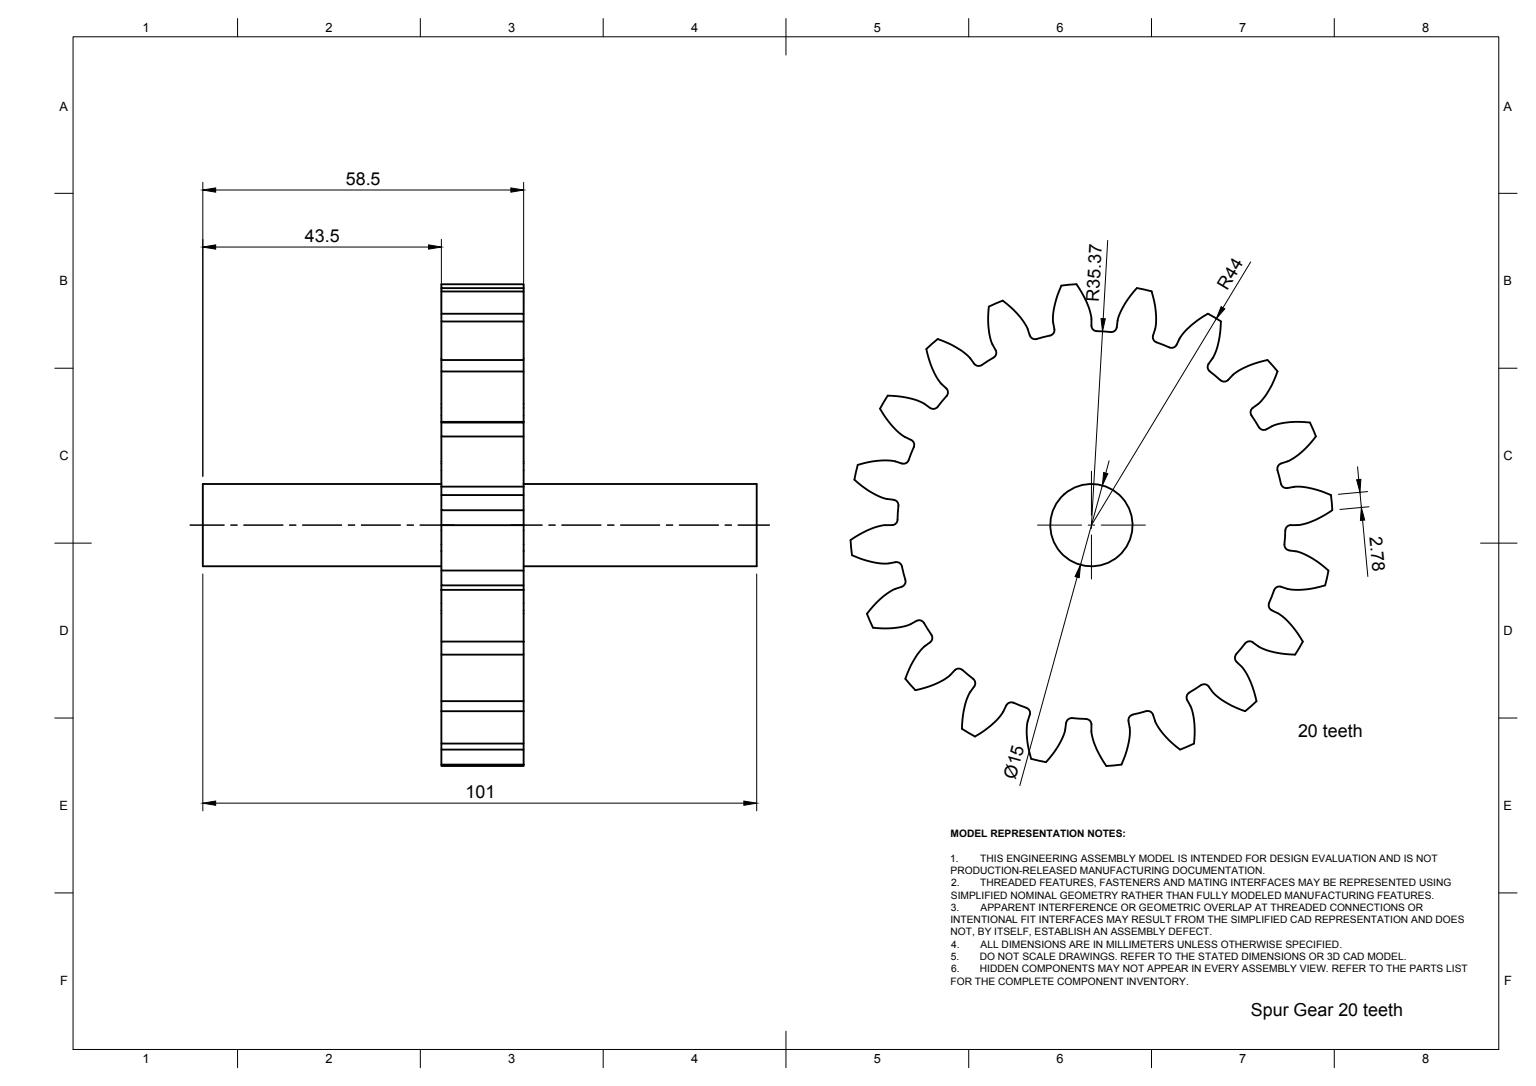
ISO-10303-21;
HEADER;
/* Generated by software containing ST-Developer
 * from STEP Tools, Inc. (www.steptools.com) 
 */

FILE_DESCRIPTION(
/* description */ (''),
/* implementation_level */ '2;1');

FILE_NAME(
/* name */ 'Spur Gear 20 teeth.step',
/* time_stamp */ '2026-10-05T21:54:13-07:00',
/* author */ (''),
/* organization */ (''),
/* preprocessor_version */ 'ST-DEVELOPER v20.2',
/* originating_system */ 'Autodesk Translation Framework v15.15.0.0',
/* authorisation */ '');

FILE_SCHEMA (('AUTOMOTIVE_DESIGN { 1 0 10303 214 3 1 1 }'));
ENDSEC;

DATA;
#10=MECHANICAL_DESIGN_GEOMETRIC_PRESENTATION_REPRESENTATION('',(#191),#43781);
#175=SHAPE_REPRESENTATION_RELATIONSHIP('SRR','None',#43813,#183);
#183=ADVANCED_BREP_SHAPE_REPRESENTATION('',(#235),#43773);
#191=STYLED_ITEM('',(#43862),#235);
#235=MANIFOLD_SOLID_BREP('Body1',#13051);
#279=FACE_BOUND('',#2177,.T.);
#280=FACE_BOUND('',#2179,.T.);
#491=B_SPLINE_CURVE_WITH_KNOTS('',5,(#19556,#19557,#19558,#19559,#19560,
#19561,#19562,#19563,#19564,#19565,#19566,#19567,#19568,#19569,#19570,#19571,
#19572,#19573,#19574,#19575,#19576,#19577,#19578,#19579,#19580,#19581,#19582,
#19583,#19584,#19585,#19586,#19587,#19588,#19589,#19590,#19591,#19592,#19593,
#19594,#19595,#19596,#19597,#19598,#19599,#19600,#19601,#19602,#19603,#19604,
#19605,#19606,#19607,#19608,#19609,#19610,#19611,#19612,#19613,#19614,#19615,
#19616,#19617,#19618,#19619,#19620,#19621,#19622,#19623,#19624,#19625,#19626,
#19627,#19628,#19629),.UNSPECIFIED.,.F.,.F.,(6,1,1,1,1,1,1,1,1,1,1,1,1,
1,1,1,1,1,1,1,1,1,1,1,1,1,1,1,1,1,1,1,1,1,1,1,1,1,1,1,1,1,1,1,1,1,1,1,1,
1,1,1,1,1,1,1,1,1,1,1,1,1,1,1,1,1,1,1,1,6),(0.,0.0142857142857143,0.0285714285714286,
0.0428571428571429,0.0571428571428571,0.0714285714285714,0.0857142857142857,
0.1,0.114285714285714,0.128571428571429,0.142857142857143,0.157142857142857,
0.171428571428571,0.185714285714286,0.2,0.214285714285714,0.228571428571429,
0.242857142857143,0.257142857142857,0.271428571428571,0.285714285714286,
0.3,0.314285714285714,0.328571428571429,0.342857142857143,0.357142857142857,
0.371428571428571,0.385714285714286,0.4,0.414285714285714,0.428571428571429,
0.442857142857143,0.457142857142857,0.471428571428572,0.485714285714286,
0.5,0.514285714285714,0.528571428571429,0.542857142857143,0.557142857142857,
0.571428571428571,0.585714285714286,0.6,0.614285714285714,0.628571428571428,
0.642857142857142,0.657142857142857,0.671428571428571,0.685714285714285,
0.699999999999999,0.714285714285714,0.728571428571428,0.742857142857142,
0.757142857142856,0.771428571428571,0.785714285714285,0.799999999999999,
0.814285714285713,0.828571428571428,0.842857142857142,0.857142857142856,
0.87142857142857,0.885714285714284,0.899999999999999,0.914285714285713,
0.928571428571427,0.942857142857141,0.957142857142856,0.97142857142857,
1.),.UNSPECIFIED.);
#492=B_SPLINE_CURVE_WITH_KNOTS('',5,(#19631,#19632,#19633,#19634,#19635,
#19636,#19637,#19638,#19639,#19640,#19641,#19642,#19643,#19644,#19645,#19646,
#19647,#19648,#19649,#19650,#19651,#19652,#19653,#19654,#19655,#19656,#19657,
#19658,#19659,#19660,#19661,#19662,#19663,#19664,#19665,#19666,#19667,#19668,
#19669,#19670,#19671,#19672,#19673,#19674,#19675,#19676,#19677,#19678,#19679,
#19680,#19681,#19682,#19683,#19684,#19685,#19686,#19687,#19688,#19689,#19690,
#19691,#19692,#19693,#19694,#19695,#19696,#19697,#19698,#19699,#19700,#19701,
#19702,#19703,#19704,#19705),.UNSPECIFIED.,.F.,.F.,(6,1,1,1,1,1,1,1,1,1,
1,1,1,1,1,1,1,1,1,1,1,1,1,1,1,1,1,1,1,1,1,1,1,1,1,1,1,1,1,1,1,1,1,1,1,1,
1,1,1,1,1,1,1,1,1,1,1,1,1,1,1,1,1,1,1,1,1,1,1,1,6),(-1.,-0.985714285714284,
-0.97142857142857,-0.957142857142856,-0.942857142857141,-0.928571428571427,
-0.914285714285713,-0.899999999999999,-0.885714285714284,-0.87142857142857,
-0.857142857142856,-0.842857142857142,-0.828571428571428,-0.814285714285713,
-0.799999999999999,-0.785714285714285,-0.771428571428571,-0.757142857142856,
-0.742857142857142,-0.728571428571428,-0.714285714285714,-0.699999999999999,
-0.685714285714285,-0.671428571428571,-0.657142857142857,-0.642857142857142,
-0.628571428571428,-0.614285714285714,-0.6,-0.585714285714286,-0.571428571428571,
-0.557142857142857,-0.542857142857143,-0.528571428571429,-0.514285714285714,
-0.5,-0.485714285714286,-0.471428571428572,-0.457142857142857,-0.442857142857143,
-0.428571428571429,-0.414285714285714,-0.4,-0.385714285714286,-0.371428571428571,
-0.357142857142857,-0.342857142857143,-0.328571428571429,-0.314285714285714,
-0.3,-0.285714285714286,-0.271428571428571,-0.257142857142857,-0.242857142857143,
-0.228571428571429,-0.214285714285714,-0.2,-0.185714285714286,-0.171428571428571,
-0.157142857142857,-0.142857142857143,-0.128571428571429,-0.114285714285714,
-0.1,-0.0857142857142857,-0.0714285714285714,-0.0571428571428571,-0.0428571428571429,
-0.0285714285714286,-0.0142857142857143,0.),.UNSPECIFIED.);
#493=B_SPLINE_CURVE_WITH_KNOTS('',5,(#19863,#19864,#19865,#19866,#19867,
#19868,#19869,#19870,#19871,#19872,#19873,#19874,#19875,#19876,#19877,#19878,
#19879,#19880,#19881,#19882,#19883,#19884,#19885,#19886,#19887,#19888,#19889,
#19890,#19891,#19892,#19893,#19894,#19895,#19896,#19897,#19898,#19899,#19900,
#19901,#19902,#19903,#19904,#19905,#19906,#19907,#19908,#19909,#19910,#19911,
#19912,#19913,#19914,#19915,#19916,#19917,#19918,#19919,#19920,#19921,#19922,
#19923,#19924,#19925,#19926,#19927,#19928,#19929,#19930,#19931,#19932,#19933,
#19934,#19935,#19936),.UNSPECIFIED.,.F.,.F.,(6,1,1,1,1,1,1,1,1,1,1,1,1,
1,1,1,1,1,1,1,1,1,1,1,1,1,1,1,1,1,1,1,1,1,1,1,1,1,1,1,1,1,1,1,1,1,1,1,1,
1,1,1,1,1,1,1,1,1,1,1,1,1,1,1,1,1,1,1,1,6),(0.,0.0142857142857143,0.0285714285714286,
0.0428571428571429,0.0571428571428571,0.0714285714285714,0.0857142857142857,
0.1,0.114285714285714,0.128571428571429,0.142857142857143,0.157142857142857,
0.171428571428571,0.185714285714286,0.2,0.214285714285714,0.228571428571429,
0.242857142857143,0.257142857142857,0.271428571428571,0.285714285714286,
0.3,0.314285714285714,0.328571428571429,0.342857142857143,0.357142857142857,
0.371428571428571,0.385714285714286,0.4,0.414285714285714,0.428571428571429,
0.442857142857143,0.457142857142857,0.471428571428572,0.485714285714286,
0.5,0.514285714285714,0.528571428571429,0.542857142857143,0.557142857142857,
0.571428571428571,0.585714285714286,0.6,0.614285714285714,0.628571428571428,
0.642857142857142,0.657142857142857,0.671428571428571,0.685714285714285,
0.699999999999999,0.714285714285714,0.728571428571428,0.742857142857142,
0.757142857142856,0.771428571428571,0.785714285714285,0.799999999999999,
0.814285714285713,0.828571428571428,0.842857142857142,0.857142857142856,
0.87142857142857,0.885714285714284,0.899999999999999,0.914285714285713,
0.928571428571427,0.942857142857141,0.957142857142856,0.97142857142857,
1.),.UNSPECIFIED.);
#494=B_SPLINE_CURVE_WITH_KNOTS('',5,(#19937,#19938,#19939,#19940,#19941,
#19942,#19943,#19944,#19945,#19946,#19947,#19948,#19949,#19950,#19951,#19952,
#19953,#19954,#19955,#19956,#19957,#19958,#19959,#19960,#19961,#19962,#19963,
#19964,#19965,#19966,#19967,#19968,#19969,#19970,#19971,#19972,#19973,#19974,
#19975,#19976,#19977,#19978,#19979,#19980,#19981,#19982,#19983,#19984,#19985,
#19986,#19987,#19988,#19989,#19990,#19991,#19992,#19993,#19994,#19995,#19996,
#19997,#19998,#19999,#20000,#20001,#20002,#20003,#20004,#20005,#20006,#20007,
#20008,#20009,#20010),.UNSPECIFIED.,.F.,.F.,(6,1,1,1,1,1,1,1,1,1,1,1,1,
1,1,1,1,1,1,1,1,1,1,1,1,1,1,1,1,1,1,1,1,1,1,1,1,1,1,1,1,1,1,1,1,1,1,1,1,
1,1,1,1,1,1,1,1,1,1,1,1,1,1,1,1,1,1,1,1,6),(0.,0.0142857142857143,0.0285714285714286,
0.0428571428571429,0.0571428571428571,0.0714285714285714,0.0857142857142857,
0.1,0.114285714285714,0.128571428571429,0.142857142857143,0.157142857142857,
0.171428571428571,0.185714285714286,0.2,0.214285714285714,0.228571428571429,
0.242857142857143,0.257142857142857,0.271428571428571,0.285714285714286,
0.3,0.314285714285714,0.328571428571429,0.342857142857143,0.357142857142857,
0.371428571428571,0.385714285714286,0.4,0.414285714285714,0.428571428571429,
0.442857142857143,0.457142857142857,0.471428571428572,0.485714285714286,
0.5,0.514285714285714,0.528571428571429,0.542857142857143,0.557142857142857,
0.571428571428571,0.585714285714286,0.6,0.614285714285714,0.628571428571428,
0.642857142857142,0.657142857142857,0.671428571428571,0.685714285714285,
0.699999999999999,0.714285714285714,0.728571428571428,0.742857142857142,
0.757142857142856,0.771428571428571,0.785714285714285,0.799999999999999,
0.814285714285713,0.828571428571428,0.842857142857142,0.857142857142856,
0.87142857142857,0.885714285714284,0.899999999999999,0.914285714285713,
0.928571428571427,0.942857142857141,0.957142857142856,0.97142857142857,
1.),.UNSPECIFIED.);
#495=B_SPLINE_CURVE_WITH_KNOTS('',5,(#20162,#20163,#20164,#20165,#20166,
#20167,#20168,#20169,#20170,#20171,#20172,#20173,#20174,#20175,#20176,#20177,
#20178,#20179,#20180,#20181,#20182,#20183,#20184,#20185,#20186,#20187,#20188,
#20189,#20190,#20191,#20192,#20193,#20194,#20195,#20196,#20197,#20198,#20199,
#20200,#20201,#20202,#20203,#20204,#20205,#20206,#20207,#20208,#20209,#20210,
#20211,#20212,#20213,#20214,#20215,#20216,#20217,#20218,#20219,#20220,#20221,
#20222,#20223,#20224,#20225,#20226,#20227,#20228,#20229,#20230,#20231,#20232,
#20233,#20234,#20235),.UNSPECIFIED.,.F.,.F.,(6,1,1,1,1,1,1,1,1,1,1,1,1,
1,1,1,1,1,1,1,1,1,1,1,1,1,1,1,1,1,1,1,1,1,1,1,1,1,1,1,1,1,1,1,1,1,1,1,1,
1,1,1,1,1,1,1,1,1,1,1,1,1,1,1,1,1,1,1,1,6),(0.,0.0142857142857143,0.0285714285714286,
0.0428571428571429,0.0571428571428571,0.0714285714285714,0.0857142857142857,
0.1,0.114285714285714,0.128571428571429,0.142857142857143,0.157142857142857,
0.171428571428571,0.185714285714286,0.2,0.214285714285714,0.228571428571429,
0.242857142857143,0.257142857142857,0.271428571428571,0.285714285714286,
0.3,0.314285714285714,0.328571428571429,0.342857142857143,0.357142857142857,
0.371428571428571,0.385714285714286,0.4,0.414285714285714,0.428571428571429,
0.442857142857143,0.457142857142857,0.471428571428572,0.485714285714286,
0.5,0.514285714285714,0.528571428571429,0.542857142857143,0.557142857142857,
0.571428571428571,0.585714285714286,0.6,0.614285714285714,0.628571428571428,
0.642857142857142,0.657142857142857,0.671428571428571,0.685714285714285,
0.699999999999999,0.714285714285714,0.728571428571428,0.742857142857142,
0.757142857142856,0.771428571428571,0.785714285714285,0.799999999999999,
0.814285714285713,0.828571428571428,0.842857142857142,0.857142857142856,
0.87142857142857,0.885714285714284,0.899999999999999,0.914285714285713,
0.928571428571427,0.942857142857141,0.957142857142856,0.97142857142857,
1.),.UNSPECIFIED.);
#496=B_SPLINE_CURVE_WITH_KNOTS('',5,(#20237,#20238,#20239,#20240,#20241,
#20242,#20243,#20244,#20245,#20246,#20247,#20248,#20249,#20250,#20251,#20252,
#20253,#20254,#20255,#20256,#20257,#20258,#20259,#20260,#20261,#20262,#20263,
#20264,#20265,#20266,#20267,#20268,#20269,#20270,#20271,#20272,#20273,#20274,
#20275,#20276,#20277,#20278,#20279,#20280,#20281,#20282,#20283,#20284,#20285,
#20286,#20287,#20288,#20289,#20290,#20291,#20292,#20293,#20294,#20295,#20296,
#20297,#20298,#20299,#20300,#20301,#20302,#20303,#20304,#20305,#20306,#20307,
#20308,#20309,#20310,#20311),.UNSPECIFIED.,.F.,.F.,(6,1,1,1,1,1,1,1,1,1,
1,1,1,1,1,1,1,1,1,1,1,1,1,1,1,1,1,1,1,1,1,1,1,1,1,1,1,1,1,1,1,1,1,1,1,1,
1,1,1,1,1,1,1,1,1,1,1,1,1,1,1,1,1,1,1,1,1,1,1,1,6),(-1.,-0.985714285714284,
-0.97142857142857,-0.957142857142856,-0.942857142857141,-0.928571428571427,
-0.914285714285713,-0.899999999999999,-0.885714285714284,-0.87142857142857,
-0.857142857142856,-0.842857142857142,-0.828571428571428,-0.814285714285713,
-0.799999999999999,-0.785714285714285,-0.771428571428571,-0.757142857142856,
-0.742857142857142,-0.728571428571428,-0.714285714285714,-0.699999999999999,
-0.685714285714285,-0.671428571428571,-0.657142857142857,-0.642857142857142,
-0.628571428571428,-0.614285714285714,-0.6,-0.585714285714286,-0.571428571428571,
-0.557142857142857,-0.542857142857143,-0.528571428571429,-0.514285714285714,
-0.5,-0.485714285714286,-0.471428571428572,-0.457142857142857,-0.442857142857143,
-0.428571428571429,-0.414285714285714,-0.4,-0.385714285714286,-0.371428571428571,
-0.357142857142857,-0.342857142857143,-0.328571428571429,-0.314285714285714,
-0.3,-0.285714285714286,-0.271428571428571,-0.257142857142857,-0.242857142857143,
-0.228571428571429,-0.214285714285714,-0.2,-0.185714285714286,-0.171428571428571,
-0.157142857142857,-0.142857142857143,-0.128571428571429,-0.114285714285714,
-0.1,-0.0857142857142857,-0.0714285714285714,-0.0571428571428571,-0.0428571428571429,
-0.0285714285714286,-0.0142857142857143,0.),.UNSPECIFIED.);
#497=B_SPLINE_CURVE_WITH_KNOTS('',5,(#20469,#20470,#20471,#20472,#20473,
#20474,#20475,#20476,#20477,#20478,#20479,#20480,#20481,#20482,#20483,#20484,
#20485,#20486,#20487,#20488,#20489,#20490,#20491,#20492,#20493,#20494,#20495,
#20496,#20497,#20498,#20499,#20500,#20501,#20502,#20503,#20504,#20505,#20506,
#20507,#20508,#20509,#20510,#20511,#20512,#20513,#20514,#20515,#20516,#20517,
#20518,#20519,#20520,#20521,#20522,#20523,#20524,#20525,#20526,#20527,#20528,
#20529,#20530,#20531,#20532,#20533,#20534,#20535,#20536,#20537,#20538,#20539,
#20540,#20541,#20542),.UNSPECIFIED.,.F.,.F.,(6,1,1,1,1,1,1,1,1,1,1,1,1,
1,1,1,1,1,1,1,1,1,1,1,1,1,1,1,1,1,1,1,1,1,1,1,1,1,1,1,1,1,1,1,1,1,1,1,1,
1,1,1,1,1,1,1,1,1,1,1,1,1,1,1,1,1,1,1,1,6),(0.,0.0142857142857143,0.0285714285714286,
0.0428571428571429,0.0571428571428571,0.0714285714285714,0.0857142857142857,
0.1,0.114285714285714,0.128571428571429,0.142857142857143,0.157142857142857,
0.171428571428571,0.185714285714286,0.2,0.214285714285714,0.228571428571429,
0.242857142857143,0.257142857142857,0.271428571428571,0.285714285714286,
0.3,0.314285714285714,0.328571428571429,0.342857142857143,0.357142857142857,
0.371428571428571,0.385714285714286,0.4,0.414285714285714,0.428571428571429,
0.442857142857143,0.457142857142857,0.471428571428572,0.485714285714286,
0.5,0.514285714285714,0.528571428571429,0.542857142857143,0.557142857142857,
0.571428571428571,0.585714285714286,0.6,0.614285714285714,0.628571428571428,
0.642857142857142,0.657142857142857,0.671428571428571,0.685714285714285,
0.699999999999999,0.714285714285714,0.728571428571428,0.742857142857142,
0.757142857142856,0.771428571428571,0.785714285714285,0.799999999999999,
0.814285714285713,0.828571428571428,0.842857142857142,0.857142857142856,
0.87142857142857,0.885714285714284,0.899999999999999,0.914285714285713,
0.928571428571427,0.942857142857141,0.957142857142856,0.97142857142857,
1.),.UNSPECIFIED.);
#498=B_SPLINE_CURVE_WITH_KNOTS('',5,(#20543,#20544,#20545,#20546,#20547,
#20548,#20549,#20550,#20551,#20552,#20553,#20554,#20555,#20556,#20557,#20558,
#20559,#20560,#20561,#20562,#20563,#20564,#20565,#20566,#20567,#20568,#20569,
#20570,#20571,#20572,#20573,#20574,#20575,#20576,#20577,#20578,#20579,#20580,
#20581,#20582,#20583,#20584,#20585,#20586,#20587,#20588,#20589,#20590,#20591,
#20592,#20593,#20594,#20595,#20596,#20597,#20598,#20599,#20600,#20601,#20602,
#20603,#20604,#20605,#20606,#20607,#20608,#20609,#20610,#20611,#20612,#20613,
#20614,#20615,#20616),.UNSPECIFIED.,.F.,.F.,(6,1,1,1,1,1,1,1,1,1,1,1,1,
1,1,1,1,1,1,1,1,1,1,1,1,1,1,1,1,1,1,1,1,1,1,1,1,1,1,1,1,1,1,1,1,1,1,1,1,
1,1,1,1,1,1,1,1,1,1,1,1,1,1,1,1,1,1,1,1,6),(0.,0.0142857142857143,0.0285714285714286,
0.0428571428571429,0.0571428571428571,0.0714285714285714,0.0857142857142857,
0.1,0.114285714285714,0.128571428571429,0.142857142857143,0.157142857142857,
0.171428571428571,0.185714285714286,0.2,0.214285714285714,0.228571428571429,
0.242857142857143,0.257142857142857,0.271428571428571,0.285714285714286,
0.3,0.314285714285714,0.328571428571429,0.342857142857143,0.357142857142857,
0.371428571428571,0.385714285714286,0.4,0.414285714285714,0.428571428571429,
0.442857142857143,0.457142857142857,0.471428571428572,0.485714285714286,
0.5,0.514285714285714,0.528571428571429,0.542857142857143,0.557142857142857,
0.571428571428571,0.585714285714286,0.6,0.614285714285714,0.628571428571428,
0.642857142857142,0.657142857142857,0.671428571428571,0.685714285714285,
0.699999999999999,0.714285714285714,0.728571428571428,0.742857142857142,
0.757142857142856,0.771428571428571,0.785714285714285,0.799999999999999,
0.814285714285713,0.828571428571428,0.842857142857142,0.857142857142856,
0.87142857142857,0.885714285714284,0.899999999999999,0.914285714285713,
0.928571428571427,0.942857142857141,0.957142857142856,0.97142857142857,
1.),.UNSPECIFIED.);
#499=B_SPLINE_CURVE_WITH_KNOTS('',5,(#20768,#20769,#20770,#20771,#20772,
#20773,#20774,#20775,#20776,#20777,#20778,#20779,#20780,#20781,#20782,#20783,
#20784,#20785,#20786,#20787,#20788,#20789,#20790,#20791,#20792,#20793,#20794,
#20795,#20796,#20797,#20798,#20799,#20800,#20801,#20802,#20803,#20804,#20805,
#20806,#20807,#20808,#20809,#20810,#20811,#20812,#20813,#20814,#20815,#20816,
#20817,#20818,#20819,#20820,#20821,#20822,#20823,#20824,#20825,#20826,#20827,
#20828,#20829,#20830,#20831,#20832,#20833,#20834,#20835,#20836,#20837,#20838,
#20839,#20840,#20841),.UNSPECIFIED.,.F.,.F.,(6,1,1,1,1,1,1,1,1,1,1,1,1,
1,1,1,1,1,1,1,1,1,1,1,1,1,1,1,1,1,1,1,1,1,1,1,1,1,1,1,1,1,1,1,1,1,1,1,1,
1,1,1,1,1,1,1,1,1,1,1,1,1,1,1,1,1,1,1,1,6),(0.,0.0142857142857143,0.0285714285714286,
0.0428571428571429,0.0571428571428571,0.0714285714285714,0.0857142857142857,
0.1,0.114285714285714,0.128571428571429,0.142857142857143,0.157142857142857,
0.171428571428571,0.185714285714286,0.2,0.214285714285714,0.228571428571429,
0.242857142857143,0.257142857142857,0.271428571428571,0.285714285714286,
0.3,0.314285714285714,0.328571428571429,0.342857142857143,0.357142857142857,
0.371428571428571,0.385714285714286,0.4,0.414285714285714,0.428571428571429,
0.442857142857143,0.457142857142857,0.471428571428572,0.485714285714286,
0.5,0.514285714285714,0.528571428571429,0.542857142857143,0.557142857142857,
0.571428571428571,0.585714285714286,0.6,0.614285714285714,0.628571428571428,
0.642857142857142,0.657142857142857,0.671428571428571,0.685714285714285,
0.699999999999999,0.714285714285714,0.728571428571428,0.742857142857142,
0.757142857142856,0.771428571428571,0.785714285714285,0.799999999999999,
0.814285714285713,0.828571428571428,0.842857142857142,0.857142857142856,
0.87142857142857,0.885714285714284,0.899999999999999,0.914285714285713,
0.928571428571427,0.942857142857141,0.957142857142856,0.97142857142857,
1.),.UNSPECIFIED.);
#500=B_SPLINE_CURVE_WITH_KNOTS('',5,(#20843,#20844,#20845,#20846,#20847,
#20848,#20849,#20850,#20851,#20852,#20853,#20854,#20855,#20856,#20857,#20858,
#20859,#20860,#20861,#20862,#20863,#20864,#20865,#20866,#20867,#20868,#20869,
#20870,#20871,#20872,#20873,#20874,#20875,#20876,#20877,#20878,#20879,#20880,
#20881,#20882,#20883,#20884,#20885,#20886,#20887,#20888,#20889,#20890,#20891,
#20892,#20893,#20894,#20895,#20896,#20897,#20898,#20899,#20900,#20901,#20902,
#20903,#20904,#20905,#20906,#20907,#20908,#20909,#20910,#20911,#20912,#20913,
#20914,#20915,#20916,#20917),.UNSPECIFIED.,.F.,.F.,(6,1,1,1,1,1,1,1,1,1,
1,1,1,1,1,1,1,1,1,1,1,1,1,1,1,1,1,1,1,1,1,1,1,1,1,1,1,1,1,1,1,1,1,1,1,1,
1,1,1,1,1,1,1,1,1,1,1,1,1,1,1,1,1,1,1,1,1,1,1,1,6),(-1.,-0.985714285714284,
-0.97142857142857,-0.957142857142856,-0.942857142857141,-0.928571428571427,
-0.914285714285713,-0.899999999999999,-0.885714285714284,-0.87142857142857,
-0.857142857142856,-0.842857142857142,-0.828571428571428,-0.814285714285713,
-0.799999999999999,-0.785714285714285,-0.771428571428571,-0.757142857142856,
-0.742857142857142,-0.728571428571428,-0.714285714285714,-0.699999999999999,
-0.685714285714285,-0.671428571428571,-0.657142857142857,-0.642857142857142,
-0.628571428571428,-0.614285714285714,-0.6,-0.585714285714286,-0.571428571428571,
-0.557142857142857,-0.542857142857143,-0.528571428571429,-0.514285714285714,
-0.5,-0.485714285714286,-0.471428571428572,-0.457142857142857,-0.442857142857143,
-0.428571428571429,-0.414285714285714,-0.4,-0.385714285714286,-0.371428571428571,
-0.357142857142857,-0.342857142857143,-0.328571428571429,-0.314285714285714,
-0.3,-0.285714285714286,-0.271428571428571,-0.257142857142857,-0.242857142857143,
-0.228571428571429,-0.214285714285714,-0.2,-0.185714285714286,-0.171428571428571,
-0.157142857142857,-0.142857142857143,-0.128571428571429,-0.114285714285714,
-0.1,-0.0857142857142857,-0.0714285714285714,-0.0571428571428571,-0.0428571428571429,
-0.0285714285714286,-0.0142857142857143,0.),.UNSPECIFIED.);
#501=B_SPLINE_CURVE_WITH_KNOTS('',5,(#21075,#21076,#21077,#21078,#21079,
#21080,#21081,#21082,#21083,#21084,#21085,#21086,#21087,#21088,#21089,#21090,
#21091,#21092,#21093,#21094,#21095,#21096,#21097,#21098,#21099,#21100,#21101,
#21102,#21103,#21104,#21105,#21106,#21107,#21108,#21109,#21110,#21111,#21112,
#21113,#21114,#21115,#21116,#21117,#21118,#21119,#21120,#21121,#21122,#21123,
#21124,#21125,#21126,#21127,#21128,#21129,#21130,#21131,#21132,#21133,#21134,
#21135,#21136,#21137,#21138,#21139,#21140,#21141,#21142,#21143,#21144,#21145,
#21146,#21147,#21148),.UNSPECIFIED.,.F.,.F.,(6,1,1,1,1,1,1,1,1,1,1,1,1,
1,1,1,1,1,1,1,1,1,1,1,1,1,1,1,1,1,1,1,1,1,1,1,1,1,1,1,1,1,1,1,1,1,1,1,1,
1,1,1,1,1,1,1,1,1,1,1,1,1,1,1,1,1,1,1,1,6),(0.,0.0142857142857143,0.0285714285714286,
0.0428571428571429,0.0571428571428571,0.0714285714285714,0.0857142857142857,
0.1,0.114285714285714,0.128571428571429,0.142857142857143,0.157142857142857,
0.171428571428571,0.185714285714286,0.2,0.214285714285714,0.228571428571429,
0.242857142857143,0.257142857142857,0.271428571428571,0.285714285714286,
0.3,0.314285714285714,0.328571428571429,0.342857142857143,0.357142857142857,
0.371428571428571,0.385714285714286,0.4,0.414285714285714,0.428571428571429,
0.442857142857143,0.457142857142857,0.471428571428572,0.485714285714286,
0.5,0.514285714285714,0.528571428571429,0.542857142857143,0.557142857142857,
0.571428571428571,0.585714285714286,0.6,0.614285714285714,0.628571428571428,
0.642857142857142,0.657142857142857,0.671428571428571,0.685714285714285,
0.699999999999999,0.714285714285714,0.728571428571428,0.742857142857142,
0.757142857142856,0.771428571428571,0.785714285714285,0.799999999999999,
0.814285714285713,0.828571428571428,0.842857142857142,0.857142857142856,
0.87142857142857,0.885714285714284,0.899999999999999,0.914285714285713,
0.928571428571427,0.942857142857141,0.957142857142856,0.97142857142857,
1.),.UNSPECIFIED.);
#502=B_SPLINE_CURVE_WITH_KNOTS('',5,(#21149,#21150,#21151,#21152,#21153,
#21154,#21155,#21156,#21157,#21158,#21159,#21160,#21161,#21162,#21163,#21164,
#21165,#21166,#21167,#21168,#21169,#21170,#21171,#21172,#21173,#21174,#21175,
#21176,#21177,#21178,#21179,#21180,#21181,#21182,#21183,#21184,#21185,#21186,
#21187,#21188,#21189,#21190,#21191,#21192,#21193,#21194,#21195,#21196,#21197,
#21198,#21199,#21200,#21201,#21202,#21203,#21204,#21205,#21206,#21207,#21208,
#21209,#21210,#21211,#21212,#21213,#21214,#21215,#21216,#21217,#21218,#21219,
#21220,#21221,#21222),.UNSPECIFIED.,.F.,.F.,(6,1,1,1,1,1,1,1,1,1,1,1,1,
1,1,1,1,1,1,1,1,1,1,1,1,1,1,1,1,1,1,1,1,1,1,1,1,1,1,1,1,1,1,1,1,1,1,1,1,
1,1,1,1,1,1,1,1,1,1,1,1,1,1,1,1,1,1,1,1,6),(0.,0.0142857142857143,0.0285714285714286,
0.0428571428571429,0.0571428571428571,0.0714285714285714,0.0857142857142857,
0.1,0.114285714285714,0.128571428571429,0.142857142857143,0.157142857142857,
0.171428571428571,0.185714285714286,0.2,0.214285714285714,0.228571428571429,
0.242857142857143,0.257142857142857,0.271428571428571,0.285714285714286,
0.3,0.314285714285714,0.328571428571429,0.342857142857143,0.357142857142857,
0.371428571428571,0.385714285714286,0.4,0.414285714285714,0.428571428571429,
0.442857142857143,0.457142857142857,0.471428571428572,0.485714285714286,
0.5,0.514285714285714,0.528571428571429,0.542857142857143,0.557142857142857,
0.571428571428571,0.585714285714286,0.6,0.614285714285714,0.628571428571428,
0.642857142857142,0.657142857142857,0.671428571428571,0.685714285714285,
0.699999999999999,0.714285714285714,0.728571428571428,0.742857142857142,
0.757142857142856,0.771428571428571,0.785714285714285,0.799999999999999,
0.814285714285713,0.828571428571428,0.842857142857142,0.857142857142856,
0.87142857142857,0.885714285714284,0.899999999999999,0.914285714285713,
0.928571428571427,0.942857142857141,0.957142857142856,0.97142857142857,
1.),.UNSPECIFIED.);
#503=B_SPLINE_CURVE_WITH_KNOTS('',5,(#21374,#21375,#21376,#21377,#21378,
#21379,#21380,#21381,#21382,#21383,#21384,#21385,#21386,#21387,#21388,#21389,
#21390,#21391,#21392,#21393,#21394,#21395,#21396,#21397,#21398,#21399,#21400,
#21401,#21402,#21403,#21404,#21405,#21406,#21407,#21408,#21409,#21410,#21411,
#21412,#21413,#21414,#21415,#21416,#21417,#21418,#21419,#21420,#21421,#21422,
#21423,#21424,#21425,#21426,#21427,#21428,#21429,#21430,#21431,#21432,#21433,
#21434,#21435,#21436,#21437,#21438,#21439,#21440,#21441,#21442,#21443,#21444,
#21445,#21446,#21447),.UNSPECIFIED.,.F.,.F.,(6,1,1,1,1,1,1,1,1,1,1,1,1,
1,1,1,1,1,1,1,1,1,1,1,1,1,1,1,1,1,1,1,1,1,1,1,1,1,1,1,1,1,1,1,1,1,1,1,1,
1,1,1,1,1,1,1,1,1,1,1,1,1,1,1,1,1,1,1,1,6),(0.,0.0142857142857143,0.0285714285714286,
0.0428571428571429,0.0571428571428571,0.0714285714285714,0.0857142857142857,
0.1,0.114285714285714,0.128571428571429,0.142857142857143,0.157142857142857,
0.171428571428571,0.185714285714286,0.2,0.214285714285714,0.228571428571429,
0.242857142857143,0.257142857142857,0.271428571428571,0.285714285714286,
0.3,0.314285714285714,0.328571428571429,0.342857142857143,0.357142857142857,
0.371428571428571,0.385714285714286,0.4,0.414285714285714,0.428571428571429,
0.442857142857143,0.457142857142857,0.471428571428572,0.485714285714286,
0.5,0.514285714285714,0.528571428571429,0.542857142857143,0.557142857142857,
0.571428571428571,0.585714285714286,0.6,0.614285714285714,0.628571428571428,
0.642857142857142,0.657142857142857,0.671428571428571,0.685714285714285,
0.699999999999999,0.714285714285714,0.728571428571428,0.742857142857142,
0.757142857142856,0.771428571428571,0.785714285714285,0.799999999999999,
0.814285714285713,0.828571428571428,0.842857142857142,0.857142857142856,
0.87142857142857,0.885714285714284,0.899999999999999,0.914285714285713,
0.928571428571427,0.942857142857141,0.957142857142856,0.97142857142857,
1.),.UNSPECIFIED.);
#504=B_SPLINE_CURVE_WITH_KNOTS('',5,(#21449,#21450,#21451,#21452,#21453,
#21454,#21455,#21456,#21457,#21458,#21459,#21460,#21461,#21462,#21463,#21464,
#21465,#21466,#21467,#21468,#21469,#21470,#21471,#21472,#21473,#21474,#21475,
#21476,#21477,#21478,#21479,#21480,#21481,#21482,#21483,#21484,#21485,#21486,
#21487,#21488,#21489,#21490,#21491,#21492,#21493,#21494,#21495,#21496,#21497,
#21498,#21499,#21500,#21501,#21502,#21503,#21504,#21505,#21506,#21507,#21508,
#21509,#21510,#21511,#21512,#21513,#21514,#21515,#21516,#21517,#21518,#21519,
#21520,#21521,#21522,#21523),.UNSPECIFIED.,.F.,.F.,(6,1,1,1,1,1,1,1,1,1,
1,1,1,1,1,1,1,1,1,1,1,1,1,1,1,1,1,1,1,1,1,1,1,1,1,1,1,1,1,1,1,1,1,1,1,1,
1,1,1,1,1,1,1,1,1,1,1,1,1,1,1,1,1,1,1,1,1,1,1,1,6),(-1.,-0.985714285714284,
-0.97142857142857,-0.957142857142856,-0.942857142857141,-0.928571428571427,
-0.914285714285713,-0.899999999999999,-0.885714285714284,-0.87142857142857,
-0.857142857142856,-0.842857142857142,-0.828571428571428,-0.814285714285713,
-0.799999999999999,-0.785714285714285,-0.771428571428571,-0.757142857142856,
-0.742857142857142,-0.728571428571428,-0.714285714285714,-0.699999999999999,
-0.685714285714285,-0.671428571428571,-0.657142857142857,-0.642857142857142,
-0.628571428571428,-0.614285714285714,-0.6,-0.585714285714286,-0.571428571428571,
-0.557142857142857,-0.542857142857143,-0.528571428571429,-0.514285714285714,
-0.5,-0.485714285714286,-0.471428571428572,-0.457142857142857,-0.442857142857143,
-0.428571428571429,-0.414285714285714,-0.4,-0.385714285714286,-0.371428571428571,
-0.357142857142857,-0.342857142857143,-0.328571428571429,-0.314285714285714,
-0.3,-0.285714285714286,-0.271428571428571,-0.257142857142857,-0.242857142857143,
-0.228571428571429,-0.214285714285714,-0.2,-0.185714285714286,-0.171428571428571,
-0.157142857142857,-0.142857142857143,-0.128571428571429,-0.114285714285714,
-0.1,-0.0857142857142857,-0.0714285714285714,-0.0571428571428571,-0.0428571428571429,
-0.0285714285714286,-0.0142857142857143,0.),.UNSPECIFIED.);
#505=B_SPLINE_CURVE_WITH_KNOTS('',5,(#21681,#21682,#21683,#21684,#21685,
#21686,#21687,#21688,#21689,#21690,#21691,#21692,#21693,#21694,#21695,#21696,
#21697,#21698,#21699,#21700,#21701,#21702,#21703,#21704,#21705,#21706,#21707,
#21708,#21709,#21710,#21711,#21712,#21713,#21714,#21715,#21716,#21717,#21718,
#21719,#21720,#21721,#21722,#21723,#21724,#21725,#21726,#21727,#21728,#21729,
#21730,#21731,#21732,#21733,#21734,#21735,#21736,#21737,#21738,#21739,#21740,
#21741,#21742,#21743,#21744,#21745,#21746,#21747,#21748,#21749,#21750,#21751,
#21752,#21753,#21754),.UNSPECIFIED.,.F.,.F.,(6,1,1,1,1,1,1,1,1,1,1,1,1,
1,1,1,1,1,1,1,1,1,1,1,1,1,1,1,1,1,1,1,1,1,1,1,1,1,1,1,1,1,1,1,1,1,1,1,1,
1,1,1,1,1,1,1,1,1,1,1,1,1,1,1,1,1,1,1,1,6),(0.,0.0142857142857143,0.0285714285714286,
0.0428571428571429,0.0571428571428571,0.0714285714285714,0.0857142857142857,
0.1,0.114285714285714,0.128571428571429,0.142857142857143,0.157142857142857,
0.171428571428571,0.185714285714286,0.2,0.214285714285714,0.228571428571429,
0.242857142857143,0.257142857142857,0.271428571428571,0.285714285714286,
0.3,0.314285714285714,0.328571428571429,0.342857142857143,0.357142857142857,
0.371428571428571,0.385714285714286,0.4,0.414285714285714,0.428571428571429,
0.442857142857143,0.457142857142857,0.471428571428572,0.485714285714286,
0.5,0.514285714285714,0.528571428571429,0.542857142857143,0.557142857142857,
0.571428571428571,0.585714285714286,0.6,0.614285714285714,0.628571428571428,
0.642857142857142,0.657142857142857,0.671428571428571,0.685714285714285,
0.699999999999999,0.714285714285714,0.728571428571428,0.742857142857142,
0.757142857142856,0.771428571428571,0.785714285714285,0.799999999999999,
0.814285714285713,0.828571428571428,0.842857142857142,0.857142857142856,
0.87142857142857,0.885714285714284,0.899999999999999,0.914285714285713,
0.928571428571427,0.942857142857141,0.957142857142856,0.97142857142857,
1.),.UNSPECIFIED.);
#506=B_SPLINE_CURVE_WITH_KNOTS('',5,(#21755,#21756,#21757,#21758,#21759,
#21760,#21761,#21762,#21763,#21764,#21765,#21766,#21767,#21768,#21769,#21770,
#21771,#21772,#21773,#21774,#21775,#21776,#21777,#21778,#21779,#21780,#21781,
#21782,#21783,#21784,#21785,#21786,#21787,#21788,#21789,#21790,#21791,#21792,
#21793,#21794,#21795,#21796,#21797,#21798,#21799,#21800,#21801,#21802,#21803,
#21804,#21805,#21806,#21807,#21808,#21809,#21810,#21811,#21812,#21813,#21814,
#21815,#21816,#21817,#21818,#21819,#21820,#21821,#21822,#21823,#21824,#21825,
#21826,#21827,#21828),.UNSPECIFIED.,.F.,.F.,(6,1,1,1,1,1,1,1,1,1,1,1,1,
1,1,1,1,1,1,1,1,1,1,1,1,1,1,1,1,1,1,1,1,1,1,1,1,1,1,1,1,1,1,1,1,1,1,1,1,
1,1,1,1,1,1,1,1,1,1,1,1,1,1,1,1,1,1,1,1,6),(0.,0.0142857142857143,0.0285714285714286,
0.0428571428571429,0.0571428571428571,0.0714285714285714,0.0857142857142857,
0.1,0.114285714285714,0.128571428571429,0.142857142857143,0.157142857142857,
0.171428571428571,0.185714285714286,0.2,0.214285714285714,0.228571428571429,
0.242857142857143,0.257142857142857,0.271428571428571,0.285714285714286,
0.3,0.314285714285714,0.328571428571429,0.342857142857143,0.357142857142857,
0.371428571428571,0.385714285714286,0.4,0.414285714285714,0.428571428571429,
0.442857142857143,0.457142857142857,0.471428571428572,0.485714285714286,
0.5,0.514285714285714,0.528571428571429,0.542857142857143,0.557142857142857,
0.571428571428571,0.585714285714286,0.6,0.614285714285714,0.628571428571428,
0.642857142857142,0.657142857142857,0.671428571428571,0.685714285714285,
0.699999999999999,0.714285714285714,0.728571428571428,0.742857142857142,
0.757142857142856,0.771428571428571,0.785714285714285,0.799999999999999,
0.814285714285713,0.828571428571428,0.842857142857142,0.857142857142856,
0.87142857142857,0.885714285714284,0.899999999999999,0.914285714285713,
0.928571428571427,0.942857142857141,0.957142857142856,0.97142857142857,
1.),.UNSPECIFIED.);
#507=B_SPLINE_CURVE_WITH_KNOTS('',5,(#21980,#21981,#21982,#21983,#21984,
#21985,#21986,#21987,#21988,#21989,#21990,#21991,#21992,#21993,#21994,#21995,
#21996,#21997,#21998,#21999,#22000,#22001,#22002,#22003,#22004,#22005,#22006,
#22007,#22008,#22009,#22010,#22011,#22012,#22013,#22014,#22015,#22016,#22017,
#22018,#22019,#22020,#22021,#22022,#22023,#22024,#22025,#22026,#22027,#22028,
#22029,#22030,#22031,#22032,#22033,#22034,#22035,#22036,#22037,#22038,#22039,
#22040,#22041,#22042,#22043,#22044,#22045,#22046,#22047,#22048,#22049,#22050,
#22051,#22052,#22053),.UNSPECIFIED.,.F.,.F.,(6,1,1,1,1,1,1,1,1,1,1,1,1,
1,1,1,1,1,1,1,1,1,1,1,1,1,1,1,1,1,1,1,1,1,1,1,1,1,1,1,1,1,1,1,1,1,1,1,1,
1,1,1,1,1,1,1,1,1,1,1,1,1,1,1,1,1,1,1,1,6),(0.,0.0142857142857143,0.0285714285714286,
0.0428571428571429,0.0571428571428571,0.0714285714285714,0.0857142857142857,
0.1,0.114285714285714,0.128571428571429,0.142857142857143,0.157142857142857,
0.171428571428571,0.185714285714286,0.2,0.214285714285714,0.228571428571429,
0.242857142857143,0.257142857142857,0.271428571428571,0.285714285714286,
0.3,0.314285714285714,0.328571428571429,0.342857142857143,0.357142857142857,
0.371428571428571,0.385714285714286,0.4,0.414285714285714,0.428571428571429,
0.442857142857143,0.457142857142857,0.471428571428572,0.485714285714286,
0.5,0.514285714285714,0.528571428571429,0.542857142857143,0.557142857142857,
0.571428571428571,0.585714285714286,0.6,0.614285714285714,0.628571428571428,
0.642857142857142,0.657142857142857,0.671428571428571,0.685714285714285,
0.699999999999999,0.714285714285714,0.728571428571428,0.742857142857142,
0.757142857142856,0.771428571428571,0.785714285714285,0.799999999999999,
0.814285714285713,0.828571428571428,0.842857142857142,0.857142857142856,
0.87142857142857,0.885714285714284,0.899999999999999,0.914285714285713,
0.928571428571427,0.942857142857141,0.957142857142856,0.97142857142857,
1.),.UNSPECIFIED.);
#508=B_SPLINE_CURVE_WITH_KNOTS('',5,(#22055,#22056,#22057,#22058,#22059,
#22060,#22061,#22062,#22063,#22064,#22065,#22066,#22067,#22068,#22069,#22070,
#22071,#22072,#22073,#22074,#22075,#22076,#22077,#22078,#22079,#22080,#22081,
#22082,#22083,#22084,#22085,#22086,#22087,#22088,#22089,#22090,#22091,#22092,
#22093,#22094,#22095,#22096,#22097,#22098,#22099,#22100,#22101,#22102,#22103,
#22104,#22105,#22106,#22107,#22108,#22109,#22110,#22111,#22112,#22113,#22114,
#22115,#22116,#22117,#22118,#22119,#22120,#22121,#22122,#22123,#22124,#22125,
#22126,#22127,#22128,#22129),.UNSPECIFIED.,.F.,.F.,(6,1,1,1,1,1,1,1,1,1,
1,1,1,1,1,1,1,1,1,1,1,1,1,1,1,1,1,1,1,1,1,1,1,1,1,1,1,1,1,1,1,1,1,1,1,1,
1,1,1,1,1,1,1,1,1,1,1,1,1,1,1,1,1,1,1,1,1,1,1,1,6),(-1.,-0.985714285714284,
-0.97142857142857,-0.957142857142856,-0.942857142857141,-0.928571428571427,
-0.914285714285713,-0.899999999999999,-0.885714285714284,-0.87142857142857,
-0.857142857142856,-0.842857142857142,-0.828571428571428,-0.814285714285713,
-0.799999999999999,-0.785714285714285,-0.771428571428571,-0.757142857142856,
-0.742857142857142,-0.728571428571428,-0.714285714285714,-0.699999999999999,
-0.685714285714285,-0.671428571428571,-0.657142857142857,-0.642857142857142,
-0.628571428571428,-0.614285714285714,-0.6,-0.585714285714286,-0.571428571428571,
-0.557142857142857,-0.542857142857143,-0.528571428571429,-0.514285714285714,
-0.5,-0.485714285714286,-0.471428571428572,-0.457142857142857,-0.442857142857143,
-0.428571428571429,-0.414285714285714,-0.4,-0.385714285714286,-0.371428571428571,
-0.357142857142857,-0.342857142857143,-0.328571428571429,-0.314285714285714,
-0.3,-0.285714285714286,-0.271428571428571,-0.257142857142857,-0.242857142857143,
-0.228571428571429,-0.214285714285714,-0.2,-0.185714285714286,-0.171428571428571,
-0.157142857142857,-0.142857142857143,-0.128571428571429,-0.114285714285714,
-0.1,-0.0857142857142857,-0.0714285714285714,-0.0571428571428571,-0.0428571428571429,
-0.0285714285714286,-0.0142857142857143,0.),.UNSPECIFIED.);
#509=B_SPLINE_CURVE_WITH_KNOTS('',5,(#22287,#22288,#22289,#22290,#22291,
#22292,#22293,#22294,#22295,#22296,#22297,#22298,#22299,#22300,#22301,#22302,
#22303,#22304,#22305,#22306,#22307,#22308,#22309,#22310,#22311,#22312,#22313,
#22314,#22315,#22316,#22317,#22318,#22319,#22320,#22321,#22322,#22323,#22324,
#22325,#22326,#22327,#22328,#22329,#22330,#22331,#22332,#22333,#22334,#22335,
#22336,#22337,#22338,#22339,#22340,#22341,#22342,#22343,#22344,#22345,#22346,
#22347,#22348,#22349,#22350,#22351,#22352,#22353,#22354,#22355,#22356,#22357,
#22358,#22359,#22360),.UNSPECIFIED.,.F.,.F.,(6,1,1,1,1,1,1,1,1,1,1,1,1,
1,1,1,1,1,1,1,1,1,1,1,1,1,1,1,1,1,1,1,1,1,1,1,1,1,1,1,1,1,1,1,1,1,1,1,1,
1,1,1,1,1,1,1,1,1,1,1,1,1,1,1,1,1,1,1,1,6),(0.,0.0142857142857143,0.0285714285714286,
0.0428571428571429,0.0571428571428571,0.0714285714285714,0.0857142857142857,
0.1,0.114285714285714,0.128571428571429,0.142857142857143,0.157142857142857,
0.171428571428571,0.185714285714286,0.2,0.214285714285714,0.228571428571429,
0.242857142857143,0.257142857142857,0.271428571428571,0.285714285714286,
0.3,0.314285714285714,0.328571428571429,0.342857142857143,0.357142857142857,
0.371428571428571,0.385714285714286,0.4,0.414285714285714,0.428571428571429,
0.442857142857143,0.457142857142857,0.471428571428572,0.485714285714286,
0.5,0.514285714285714,0.528571428571429,0.542857142857143,0.557142857142857,
0.571428571428571,0.585714285714286,0.6,0.614285714285714,0.628571428571428,
0.642857142857142,0.657142857142857,0.671428571428571,0.685714285714285,
0.699999999999999,0.714285714285714,0.728571428571428,0.742857142857142,
0.757142857142856,0.771428571428571,0.785714285714285,0.799999999999999,
0.814285714285713,0.828571428571428,0.842857142857142,0.857142857142856,
0.87142857142857,0.885714285714284,0.899999999999999,0.914285714285713,
0.928571428571427,0.942857142857141,0.957142857142856,0.97142857142857,
1.),.UNSPECIFIED.);
#510=B_SPLINE_CURVE_WITH_KNOTS('',5,(#22361,#22362,#22363,#22364,#22365,
#22366,#22367,#22368,#22369,#22370,#22371,#22372,#22373,#22374,#22375,#22376,
#22377,#22378,#22379,#22380,#22381,#22382,#22383,#22384,#22385,#22386,#22387,
#22388,#22389,#22390,#22391,#22392,#22393,#22394,#22395,#22396,#22397,#22398,
#22399,#22400,#22401,#22402,#22403,#22404,#22405,#22406,#22407,#22408,#22409,
#22410,#22411,#22412,#22413,#22414,#22415,#22416,#22417,#22418,#22419,#22420,
#22421,#22422,#22423,#22424,#22425,#22426,#22427,#22428,#22429,#22430,#22431,
#22432,#22433,#22434),.UNSPECIFIED.,.F.,.F.,(6,1,1,1,1,1,1,1,1,1,1,1,1,
1,1,1,1,1,1,1,1,1,1,1,1,1,1,1,1,1,1,1,1,1,1,1,1,1,1,1,1,1,1,1,1,1,1,1,1,
1,1,1,1,1,1,1,1,1,1,1,1,1,1,1,1,1,1,1,1,6),(0.,0.0142857142857143,0.0285714285714286,
0.0428571428571429,0.0571428571428571,0.0714285714285714,0.0857142857142857,
0.1,0.114285714285714,0.128571428571429,0.142857142857143,0.157142857142857,
0.171428571428571,0.185714285714286,0.2,0.214285714285714,0.228571428571429,
0.242857142857143,0.257142857142857,0.271428571428571,0.285714285714286,
0.3,0.314285714285714,0.328571428571429,0.342857142857143,0.357142857142857,
0.371428571428571,0.385714285714286,0.4,0.414285714285714,0.428571428571429,
0.442857142857143,0.457142857142857,0.471428571428572,0.485714285714286,
0.5,0.514285714285714,0.528571428571429,0.542857142857143,0.557142857142857,
0.571428571428571,0.585714285714286,0.6,0.614285714285714,0.628571428571428,
0.642857142857142,0.657142857142857,0.671428571428571,0.685714285714285,
0.699999999999999,0.714285714285714,0.728571428571428,0.742857142857142,
0.757142857142856,0.771428571428571,0.785714285714285,0.799999999999999,
0.814285714285713,0.828571428571428,0.842857142857142,0.857142857142856,
0.87142857142857,0.885714285714284,0.899999999999999,0.914285714285713,
0.928571428571427,0.942857142857141,0.957142857142856,0.97142857142857,
1.),.UNSPECIFIED.);
#511=B_SPLINE_CURVE_WITH_KNOTS('',5,(#22586,#22587,#22588,#22589,#22590,
#22591,#22592,#22593,#22594,#22595,#22596,#22597,#22598,#22599,#22600,#22601,
#22602,#22603,#22604,#22605,#22606,#22607,#22608,#22609,#22610,#22611,#22612,
#22613,#22614,#22615,#22616,#22617,#22618,#22619,#22620,#22621,#22622,#22623,
#22624,#22625,#22626,#22627,#22628,#22629,#22630,#22631,#22632,#22633,#22634,
#22635,#22636,#22637,#22638,#22639,#22640,#22641,#22642,#22643,#22644,#22645,
#22646,#22647,#22648,#22649,#22650,#22651,#22652,#22653,#22654,#22655,#22656,
#22657,#22658,#22659),.UNSPECIFIED.,.F.,.F.,(6,1,1,1,1,1,1,1,1,1,1,1,1,
1,1,1,1,1,1,1,1,1,1,1,1,1,1,1,1,1,1,1,1,1,1,1,1,1,1,1,1,1,1,1,1,1,1,1,1,
1,1,1,1,1,1,1,1,1,1,1,1,1,1,1,1,1,1,1,1,6),(0.,0.0142857142857143,0.0285714285714286,
0.0428571428571429,0.0571428571428571,0.0714285714285714,0.0857142857142857,
0.1,0.114285714285714,0.128571428571429,0.142857142857143,0.157142857142857,
0.171428571428571,0.185714285714286,0.2,0.214285714285714,0.228571428571429,
0.242857142857143,0.257142857142857,0.271428571428571,0.285714285714286,
0.3,0.314285714285714,0.328571428571429,0.342857142857143,0.357142857142857,
0.371428571428571,0.385714285714286,0.4,0.414285714285714,0.428571428571429,
0.442857142857143,0.457142857142857,0.471428571428572,0.485714285714286,
0.5,0.514285714285714,0.528571428571429,0.542857142857143,0.557142857142857,
0.571428571428571,0.585714285714286,0.6,0.614285714285714,0.628571428571428,
0.642857142857142,0.657142857142857,0.671428571428571,0.685714285714285,
0.699999999999999,0.714285714285714,0.728571428571428,0.742857142857142,
0.757142857142856,0.771428571428571,0.785714285714285,0.799999999999999,
0.814285714285713,0.828571428571428,0.842857142857142,0.857142857142856,
0.87142857142857,0.885714285714284,0.899999999999999,0.914285714285713,
0.928571428571427,0.942857142857141,0.957142857142856,0.97142857142857,
1.),.UNSPECIFIED.);
#512=B_SPLINE_CURVE_WITH_KNOTS('',5,(#22661,#22662,#22663,#22664,#22665,
#22666,#22667,#22668,#22669,#22670,#22671,#22672,#22673,#22674,#22675,#22676,
#22677,#22678,#22679,#22680,#22681,#22682,#22683,#22684,#22685,#22686,#22687,
#22688,#22689,#22690,#22691,#22692,#22693,#22694,#22695,#22696,#22697,#22698,
#22699,#22700,#22701,#22702,#22703,#22704,#22705,#22706,#22707,#22708,#22709,
#22710,#22711,#22712,#22713,#22714,#22715,#22716,#22717,#22718,#22719,#22720,
#22721,#22722,#22723,#22724,#22725,#22726,#22727,#22728,#22729,#22730,#22731,
#22732,#22733,#22734,#22735),.UNSPECIFIED.,.F.,.F.,(6,1,1,1,1,1,1,1,1,1,
1,1,1,1,1,1,1,1,1,1,1,1,1,1,1,1,1,1,1,1,1,1,1,1,1,1,1,1,1,1,1,1,1,1,1,1,
1,1,1,1,1,1,1,1,1,1,1,1,1,1,1,1,1,1,1,1,1,1,1,1,6),(-1.,-0.985714285714284,
-0.97142857142857,-0.957142857142856,-0.942857142857141,-0.928571428571427,
-0.914285714285713,-0.899999999999999,-0.885714285714284,-0.87142857142857,
-0.857142857142856,-0.842857142857142,-0.828571428571428,-0.814285714285713,
-0.799999999999999,-0.785714285714285,-0.771428571428571,-0.757142857142856,
-0.742857142857142,-0.728571428571428,-0.714285714285714,-0.699999999999999,
-0.685714285714285,-0.671428571428571,-0.657142857142857,-0.642857142857142,
-0.628571428571428,-0.614285714285714,-0.6,-0.585714285714286,-0.571428571428571,
-0.557142857142857,-0.542857142857143,-0.528571428571429,-0.514285714285714,
-0.5,-0.485714285714286,-0.471428571428572,-0.457142857142857,-0.442857142857143,
-0.428571428571429,-0.414285714285714,-0.4,-0.385714285714286,-0.371428571428571,
-0.357142857142857,-0.342857142857143,-0.328571428571429,-0.314285714285714,
-0.3,-0.285714285714286,-0.271428571428571,-0.257142857142857,-0.242857142857143,
-0.228571428571429,-0.214285714285714,-0.2,-0.185714285714286,-0.171428571428571,
-0.157142857142857,-0.142857142857143,-0.128571428571429,-0.114285714285714,
-0.1,-0.0857142857142857,-0.0714285714285714,-0.0571428571428571,-0.0428571428571429,
-0.0285714285714286,-0.0142857142857143,0.),.UNSPECIFIED.);
#513=B_SPLINE_CURVE_WITH_KNOTS('',5,(#22893,#22894,#22895,#22896,#22897,
#22898,#22899,#22900,#22901,#22902,#22903,#22904,#22905,#22906,#22907,#22908,
#22909,#22910,#22911,#22912,#22913,#22914,#22915,#22916,#22917,#22918,#22919,
#22920,#22921,#22922,#22923,#22924,#22925,#22926,#22927,#22928,#22929,#22930,
#22931,#22932,#22933,#22934,#22935,#22936,#22937,#22938,#22939,#22940,#22941,
#22942,#22943,#22944,#22945,#22946,#22947,#22948,#22949,#22950,#22951,#22952,
#22953,#22954,#22955,#22956,#22957,#22958,#22959,#22960,#22961,#22962,#22963,
#22964,#22965,#22966),.UNSPECIFIED.,.F.,.F.,(6,1,1,1,1,1,1,1,1,1,1,1,1,
1,1,1,1,1,1,1,1,1,1,1,1,1,1,1,1,1,1,1,1,1,1,1,1,1,1,1,1,1,1,1,1,1,1,1,1,
1,1,1,1,1,1,1,1,1,1,1,1,1,1,1,1,1,1,1,1,6),(0.,0.0142857142857143,0.0285714285714286,
0.0428571428571429,0.0571428571428571,0.0714285714285714,0.0857142857142857,
0.1,0.114285714285714,0.128571428571429,0.142857142857143,0.157142857142857,
0.171428571428571,0.185714285714286,0.2,0.214285714285714,0.228571428571429,
0.242857142857143,0.257142857142857,0.271428571428571,0.285714285714286,
0.3,0.314285714285714,0.328571428571429,0.342857142857143,0.357142857142857,
0.371428571428571,0.385714285714286,0.4,0.414285714285714,0.428571428571429,
0.442857142857143,0.457142857142857,0.471428571428572,0.485714285714286,
0.5,0.514285714285714,0.528571428571429,0.542857142857143,0.557142857142857,
0.571428571428571,0.585714285714286,0.6,0.614285714285714,0.628571428571428,
0.642857142857142,0.657142857142857,0.671428571428571,0.685714285714285,
0.699999999999999,0.714285714285714,0.728571428571428,0.742857142857142,
0.757142857142856,0.771428571428571,0.785714285714285,0.799999999999999,
0.814285714285713,0.828571428571428,0.842857142857142,0.857142857142856,
0.87142857142857,0.885714285714284,0.899999999999999,0.914285714285713,
0.928571428571427,0.942857142857141,0.957142857142856,0.97142857142857,
1.),.UNSPECIFIED.);
#514=B_SPLINE_CURVE_WITH_KNOTS('',5,(#22967,#22968,#22969,#22970,#22971,
#22972,#22973,#22974,#22975,#22976,#22977,#22978,#22979,#22980,#22981,#22982,
#22983,#22984,#22985,#22986,#22987,#22988,#22989,#22990,#22991,#22992,#22993,
#22994,#22995,#22996,#22997,#22998,#22999,#23000,#23001,#23002,#23003,#23004,
#23005,#23006,#23007,#23008,#23009,#23010,#23011,#23012,#23013,#23014,#23015,
#23016,#23017,#23018,#23019,#23020,#23021,#23022,#23023,#23024,#23025,#23026,
#23027,#23028,#23029,#23030,#23031,#23032,#23033,#23034,#23035,#23036,#23037,
#23038,#23039,#23040),.UNSPECIFIED.,.F.,.F.,(6,1,1,1,1,1,1,1,1,1,1,1,1,
1,1,1,1,1,1,1,1,1,1,1,1,1,1,1,1,1,1,1,1,1,1,1,1,1,1,1,1,1,1,1,1,1,1,1,1,
1,1,1,1,1,1,1,1,1,1,1,1,1,1,1,1,1,1,1,1,6),(0.,0.0142857142857143,0.0285714285714286,
0.0428571428571429,0.0571428571428571,0.0714285714285714,0.0857142857142857,
0.1,0.114285714285714,0.128571428571429,0.142857142857143,0.157142857142857,
0.171428571428571,0.185714285714286,0.2,0.214285714285714,0.228571428571429,
0.242857142857143,0.257142857142857,0.271428571428571,0.285714285714286,
0.3,0.314285714285714,0.328571428571429,0.342857142857143,0.357142857142857,
0.371428571428571,0.385714285714286,0.4,0.414285714285714,0.428571428571429,
0.442857142857143,0.457142857142857,0.471428571428572,0.485714285714286,
0.5,0.514285714285714,0.528571428571429,0.542857142857143,0.557142857142857,
0.571428571428571,0.585714285714286,0.6,0.614285714285714,0.628571428571428,
0.642857142857142,0.657142857142857,0.671428571428571,0.685714285714285,
0.699999999999999,0.714285714285714,0.728571428571428,0.742857142857142,
0.757142857142856,0.771428571428571,0.785714285714285,0.799999999999999,
0.814285714285713,0.828571428571428,0.842857142857142,0.857142857142856,
0.87142857142857,0.885714285714284,0.899999999999999,0.914285714285713,
0.928571428571427,0.942857142857141,0.957142857142856,0.97142857142857,
1.),.UNSPECIFIED.);
#515=B_SPLINE_CURVE_WITH_KNOTS('',5,(#23192,#23193,#23194,#23195,#23196,
#23197,#23198,#23199,#23200,#23201,#23202,#23203,#23204,#23205,#23206,#23207,
#23208,#23209,#23210,#23211,#23212,#23213,#23214,#23215,#23216,#23217,#23218,
#23219,#23220,#23221,#23222,#23223,#23224,#23225,#23226,#23227,#23228,#23229,
#23230,#23231,#23232,#23233,#23234,#23235,#23236,#23237,#23238,#23239,#23240,
#23241,#23242,#23243,#23244,#23245,#23246,#23247,#23248,#23249,#23250,#23251,
#23252,#23253,#23254,#23255,#23256,#23257,#23258,#23259,#23260,#23261,#23262,
#23263,#23264,#23265),.UNSPECIFIED.,.F.,.F.,(6,1,1,1,1,1,1,1,1,1,1,1,1,
1,1,1,1,1,1,1,1,1,1,1,1,1,1,1,1,1,1,1,1,1,1,1,1,1,1,1,1,1,1,1,1,1,1,1,1,
1,1,1,1,1,1,1,1,1,1,1,1,1,1,1,1,1,1,1,1,6),(0.,0.0142857142857143,0.0285714285714286,
0.0428571428571429,0.0571428571428571,0.0714285714285714,0.0857142857142857,
0.1,0.114285714285714,0.128571428571429,0.142857142857143,0.157142857142857,
0.171428571428571,0.185714285714286,0.2,0.214285714285714,0.228571428571429,
0.242857142857143,0.257142857142857,0.271428571428571,0.285714285714286,
0.3,0.314285714285714,0.328571428571429,0.342857142857143,0.357142857142857,
0.371428571428571,0.385714285714286,0.4,0.414285714285714,0.428571428571429,
0.442857142857143,0.457142857142857,0.471428571428572,0.485714285714286,
0.5,0.514285714285714,0.528571428571429,0.542857142857143,0.557142857142857,
0.571428571428571,0.585714285714286,0.6,0.614285714285714,0.628571428571428,
0.642857142857142,0.657142857142857,0.671428571428571,0.685714285714285,
0.699999999999999,0.714285714285714,0.728571428571428,0.742857142857142,
0.757142857142856,0.771428571428571,0.785714285714285,0.799999999999999,
0.814285714285713,0.828571428571428,0.842857142857142,0.857142857142856,
0.87142857142857,0.885714285714284,0.899999999999999,0.914285714285713,
0.928571428571427,0.942857142857141,0.957142857142856,0.97142857142857,
1.),.UNSPECIFIED.);
#516=B_SPLINE_CURVE_WITH_KNOTS('',5,(#23267,#23268,#23269,#23270,#23271,
#23272,#23273,#23274,#23275,#23276,#23277,#23278,#23279,#23280,#23281,#23282,
#23283,#23284,#23285,#23286,#23287,#23288,#23289,#23290,#23291,#23292,#23293,
#23294,#23295,#23296,#23297,#23298,#23299,#23300,#23301,#23302,#23303,#23304,
#23305,#23306,#23307,#23308,#23309,#23310,#23311,#23312,#23313,#23314,#23315,
#23316,#23317,#23318,#23319,#23320,#23321,#23322,#23323,#23324,#23325,#23326,
#23327,#23328,#23329,#23330,#23331,#23332,#23333,#23334,#23335,#23336,#23337,
#23338,#23339,#23340,#23341),.UNSPECIFIED.,.F.,.F.,(6,1,1,1,1,1,1,1,1,1,
1,1,1,1,1,1,1,1,1,1,1,1,1,1,1,1,1,1,1,1,1,1,1,1,1,1,1,1,1,1,1,1,1,1,1,1,
1,1,1,1,1,1,1,1,1,1,1,1,1,1,1,1,1,1,1,1,1,1,1,1,6),(-1.,-0.985714285714284,
-0.97142857142857,-0.957142857142856,-0.942857142857141,-0.928571428571427,
-0.914285714285713,-0.899999999999999,-0.885714285714284,-0.87142857142857,
-0.857142857142856,-0.842857142857142,-0.828571428571428,-0.814285714285713,
-0.799999999999999,-0.785714285714285,-0.771428571428571,-0.757142857142856,
-0.742857142857142,-0.728571428571428,-0.714285714285714,-0.699999999999999,
-0.685714285714285,-0.671428571428571,-0.657142857142857,-0.642857142857142,
-0.628571428571428,-0.614285714285714,-0.6,-0.585714285714286,-0.571428571428571,
-0.557142857142857,-0.542857142857143,-0.528571428571429,-0.514285714285714,
-0.5,-0.485714285714286,-0.471428571428572,-0.457142857142857,-0.442857142857143,
-0.428571428571429,-0.414285714285714,-0.4,-0.385714285714286,-0.371428571428571,
-0.357142857142857,-0.342857142857143,-0.328571428571429,-0.314285714285714,
-0.3,-0.285714285714286,-0.271428571428571,-0.257142857142857,-0.242857142857143,
-0.228571428571429,-0.214285714285714,-0.2,-0.185714285714286,-0.171428571428571,
-0.157142857142857,-0.142857142857143,-0.128571428571429,-0.114285714285714,
-0.1,-0.0857142857142857,-0.0714285714285714,-0.0571428571428571,-0.0428571428571429,
-0.0285714285714286,-0.0142857142857143,0.),.UNSPECIFIED.);
#517=B_SPLINE_CURVE_WITH_KNOTS('',5,(#23499,#23500,#23501,#23502,#23503,
#23504,#23505,#23506,#23507,#23508,#23509,#23510,#23511,#23512,#23513,#23514,
#23515,#23516,#23517,#23518,#23519,#23520,#23521,#23522,#23523,#23524,#23525,
#23526,#23527,#23528,#23529,#23530,#23531,#23532,#23533,#23534,#23535,#23536,
#23537,#23538,#23539,#23540,#23541,#23542,#23543,#23544,#23545,#23546,#23547,
#23548,#23549,#23550,#23551,#23552,#23553,#23554,#23555,#23556,#23557,#23558,
#23559,#23560,#23561,#23562,#23563,#23564,#23565,#23566,#23567,#23568,#23569,
#23570,#23571,#23572),.UNSPECIFIED.,.F.,.F.,(6,1,1,1,1,1,1,1,1,1,1,1,1,
1,1,1,1,1,1,1,1,1,1,1,1,1,1,1,1,1,1,1,1,1,1,1,1,1,1,1,1,1,1,1,1,1,1,1,1,
1,1,1,1,1,1,1,1,1,1,1,1,1,1,1,1,1,1,1,1,6),(0.,0.0142857142857143,0.0285714285714286,
0.0428571428571429,0.0571428571428571,0.0714285714285714,0.0857142857142857,
0.1,0.114285714285714,0.128571428571429,0.142857142857143,0.157142857142857,
0.171428571428571,0.185714285714286,0.2,0.214285714285714,0.228571428571429,
0.242857142857143,0.257142857142857,0.271428571428571,0.285714285714286,
0.3,0.314285714285714,0.328571428571429,0.342857142857143,0.357142857142857,
0.371428571428571,0.385714285714286,0.4,0.414285714285714,0.428571428571429,
0.442857142857143,0.457142857142857,0.471428571428572,0.485714285714286,
0.5,0.514285714285714,0.528571428571429,0.542857142857143,0.557142857142857,
0.571428571428571,0.585714285714286,0.6,0.614285714285714,0.628571428571428,
0.642857142857142,0.657142857142857,0.671428571428571,0.685714285714285,
0.699999999999999,0.714285714285714,0.728571428571428,0.742857142857142,
0.757142857142856,0.771428571428571,0.785714285714285,0.799999999999999,
0.814285714285713,0.828571428571428,0.842857142857142,0.857142857142856,
0.87142857142857,0.885714285714284,0.899999999999999,0.914285714285713,
0.928571428571427,0.942857142857141,0.957142857142856,0.97142857142857,
1.),.UNSPECIFIED.);
#518=B_SPLINE_CURVE_WITH_KNOTS('',5,(#23573,#23574,#23575,#23576,#23577,
#23578,#23579,#23580,#23581,#23582,#23583,#23584,#23585,#23586,#23587,#23588,
#23589,#23590,#23591,#23592,#23593,#23594,#23595,#23596,#23597,#23598,#23599,
#23600,#23601,#23602,#23603,#23604,#23605,#23606,#23607,#23608,#23609,#23610,
#23611,#23612,#23613,#23614,#23615,#23616,#23617,#23618,#23619,#23620,#23621,
#23622,#23623,#23624,#23625,#23626,#23627,#23628,#23629,#23630,#23631,#23632,
#23633,#23634,#23635,#23636,#23637,#23638,#23639,#23640,#23641,#23642,#23643,
#23644,#23645,#23646),.UNSPECIFIED.,.F.,.F.,(6,1,1,1,1,1,1,1,1,1,1,1,1,
1,1,1,1,1,1,1,1,1,1,1,1,1,1,1,1,1,1,1,1,1,1,1,1,1,1,1,1,1,1,1,1,1,1,1,1,
1,1,1,1,1,1,1,1,1,1,1,1,1,1,1,1,1,1,1,1,6),(0.,0.0142857142857143,0.0285714285714286,
0.0428571428571429,0.0571428571428571,0.0714285714285714,0.0857142857142857,
0.1,0.114285714285714,0.128571428571429,0.142857142857143,0.157142857142857,
0.171428571428571,0.185714285714286,0.2,0.214285714285714,0.228571428571429,
0.242857142857143,0.257142857142857,0.271428571428571,0.285714285714286,
0.3,0.314285714285714,0.328571428571429,0.342857142857143,0.357142857142857,
0.371428571428571,0.385714285714286,0.4,0.414285714285714,0.428571428571429,
0.442857142857143,0.457142857142857,0.471428571428572,0.485714285714286,
0.5,0.514285714285714,0.528571428571429,0.542857142857143,0.557142857142857,
0.571428571428571,0.585714285714286,0.6,0.614285714285714,0.628571428571428,
0.642857142857142,0.657142857142857,0.671428571428571,0.685714285714285,
0.699999999999999,0.714285714285714,0.728571428571428,0.742857142857142,
0.757142857142856,0.771428571428571,0.785714285714285,0.799999999999999,
0.814285714285713,0.828571428571428,0.842857142857142,0.857142857142856,
0.87142857142857,0.885714285714284,0.899999999999999,0.914285714285713,
0.928571428571427,0.942857142857141,0.957142857142856,0.97142857142857,
1.),.UNSPECIFIED.);
#519=B_SPLINE_CURVE_WITH_KNOTS('',5,(#23798,#23799,#23800,#23801,#23802,
#23803,#23804,#23805,#23806,#23807,#23808,#23809,#23810,#23811,#23812,#23813,
#23814,#23815,#23816,#23817,#23818,#23819,#23820,#23821,#23822,#23823,#23824,
#23825,#23826,#23827,#23828,#23829,#23830,#23831,#23832,#23833,#23834,#23835,
#23836,#23837,#23838,#23839,#23840,#23841,#23842,#23843,#23844,#23845,#23846,
#23847,#23848,#23849,#23850,#23851,#23852,#23853,#23854,#23855,#23856,#23857,
#23858,#23859,#23860,#23861,#23862,#23863,#23864,#23865,#23866,#23867,#23868,
#23869,#23870,#23871),.UNSPECIFIED.,.F.,.F.,(6,1,1,1,1,1,1,1,1,1,1,1,1,
1,1,1,1,1,1,1,1,1,1,1,1,1,1,1,1,1,1,1,1,1,1,1,1,1,1,1,1,1,1,1,1,1,1,1,1,
1,1,1,1,1,1,1,1,1,1,1,1,1,1,1,1,1,1,1,1,6),(0.,0.0142857142857143,0.0285714285714286,
0.0428571428571429,0.0571428571428571,0.0714285714285714,0.0857142857142857,
0.1,0.114285714285714,0.128571428571429,0.142857142857143,0.157142857142857,
0.171428571428571,0.185714285714286,0.2,0.214285714285714,0.228571428571429,
0.242857142857143,0.257142857142857,0.271428571428571,0.285714285714286,
0.3,0.314285714285714,0.328571428571429,0.342857142857143,0.357142857142857,
0.371428571428571,0.385714285714286,0.4,0.414285714285714,0.428571428571429,
0.442857142857143,0.457142857142857,0.471428571428572,0.485714285714286,
0.5,0.514285714285714,0.528571428571429,0.542857142857143,0.557142857142857,
0.571428571428571,0.585714285714286,0.6,0.614285714285714,0.628571428571428,
0.642857142857142,0.657142857142857,0.671428571428571,0.685714285714285,
0.699999999999999,0.714285714285714,0.728571428571428,0.742857142857142,
0.757142857142856,0.771428571428571,0.785714285714285,0.799999999999999,
0.814285714285713,0.828571428571428,0.842857142857142,0.857142857142856,
0.87142857142857,0.885714285714284,0.899999999999999,0.914285714285713,
0.928571428571427,0.942857142857141,0.957142857142856,0.97142857142857,
1.),.UNSPECIFIED.);
#520=B_SPLINE_CURVE_WITH_KNOTS('',5,(#23873,#23874,#23875,#23876,#23877,
#23878,#23879,#23880,#23881,#23882,#23883,#23884,#23885,#23886,#23887,#23888,
#23889,#23890,#23891,#23892,#23893,#23894,#23895,#23896,#23897,#23898,#23899,
#23900,#23901,#23902,#23903,#23904,#23905,#23906,#23907,#23908,#23909,#23910,
#23911,#23912,#23913,#23914,#23915,#23916,#23917,#23918,#23919,#23920,#23921,
#23922,#23923,#23924,#23925,#23926,#23927,#23928,#23929,#23930,#23931,#23932,
#23933,#23934,#23935,#23936,#23937,#23938,#23939,#23940,#23941,#23942,#23943,
#23944,#23945,#23946,#23947),.UNSPECIFIED.,.F.,.F.,(6,1,1,1,1,1,1,1,1,1,
1,1,1,1,1,1,1,1,1,1,1,1,1,1,1,1,1,1,1,1,1,1,1,1,1,1,1,1,1,1,1,1,1,1,1,1,
1,1,1,1,1,1,1,1,1,1,1,1,1,1,1,1,1,1,1,1,1,1,1,1,6),(-1.,-0.985714285714284,
-0.97142857142857,-0.957142857142856,-0.942857142857141,-0.928571428571427,
-0.914285714285713,-0.899999999999999,-0.885714285714284,-0.87142857142857,
-0.857142857142856,-0.842857142857142,-0.828571428571428,-0.814285714285713,
-0.799999999999999,-0.785714285714285,-0.771428571428571,-0.757142857142856,
-0.742857142857142,-0.728571428571428,-0.714285714285714,-0.699999999999999,
-0.685714285714285,-0.671428571428571,-0.657142857142857,-0.642857142857142,
-0.628571428571428,-0.614285714285714,-0.6,-0.585714285714286,-0.571428571428571,
-0.557142857142857,-0.542857142857143,-0.528571428571429,-0.514285714285714,
-0.5,-0.485714285714286,-0.471428571428572,-0.457142857142857,-0.442857142857143,
-0.428571428571429,-0.414285714285714,-0.4,-0.385714285714286,-0.371428571428571,
-0.357142857142857,-0.342857142857143,-0.328571428571429,-0.314285714285714,
-0.3,-0.285714285714286,-0.271428571428571,-0.257142857142857,-0.242857142857143,
-0.228571428571429,-0.214285714285714,-0.2,-0.185714285714286,-0.171428571428571,
-0.157142857142857,-0.142857142857143,-0.128571428571429,-0.114285714285714,
-0.1,-0.0857142857142857,-0.0714285714285714,-0.0571428571428571,-0.0428571428571429,
-0.0285714285714286,-0.0142857142857143,0.),.UNSPECIFIED.);
#521=B_SPLINE_CURVE_WITH_KNOTS('',5,(#24105,#24106,#24107,#24108,#24109,
#24110,#24111,#24112,#24113,#24114,#24115,#24116,#24117,#24118,#24119,#24120,
#24121,#24122,#24123,#24124,#24125,#24126,#24127,#24128,#24129,#24130,#24131,
#24132,#24133,#24134,#24135,#24136,#24137,#24138,#24139,#24140,#24141,#24142,
#24143,#24144,#24145,#24146,#24147,#24148,#24149,#24150,#24151,#24152,#24153,
#24154,#24155,#24156,#24157,#24158,#24159,#24160,#24161,#24162,#24163,#24164,
#24165,#24166,#24167,#24168,#24169,#24170,#24171,#24172,#24173,#24174,#24175,
#24176,#24177,#24178),.UNSPECIFIED.,.F.,.F.,(6,1,1,1,1,1,1,1,1,1,1,1,1,
1,1,1,1,1,1,1,1,1,1,1,1,1,1,1,1,1,1,1,1,1,1,1,1,1,1,1,1,1,1,1,1,1,1,1,1,
1,1,1,1,1,1,1,1,1,1,1,1,1,1,1,1,1,1,1,1,6),(0.,0.0142857142857143,0.0285714285714286,
0.0428571428571429,0.0571428571428571,0.0714285714285714,0.0857142857142857,
0.1,0.114285714285714,0.128571428571429,0.142857142857143,0.157142857142857,
0.171428571428571,0.185714285714286,0.2,0.214285714285714,0.228571428571429,
0.242857142857143,0.257142857142857,0.271428571428571,0.285714285714286,
0.3,0.314285714285714,0.328571428571429,0.342857142857143,0.357142857142857,
0.371428571428571,0.385714285714286,0.4,0.414285714285714,0.428571428571429,
0.442857142857143,0.457142857142857,0.471428571428572,0.485714285714286,
0.5,0.514285714285714,0.528571428571429,0.542857142857143,0.557142857142857,
0.571428571428571,0.585714285714286,0.6,0.614285714285714,0.628571428571428,
0.642857142857142,0.657142857142857,0.671428571428571,0.685714285714285,
0.699999999999999,0.714285714285714,0.728571428571428,0.742857142857142,
0.757142857142856,0.771428571428571,0.785714285714285,0.799999999999999,
0.814285714285713,0.828571428571428,0.842857142857142,0.857142857142856,
0.87142857142857,0.885714285714284,0.899999999999999,0.914285714285713,
0.928571428571427,0.942857142857141,0.957142857142856,0.97142857142857,
1.),.UNSPECIFIED.);
#522=B_SPLINE_CURVE_WITH_KNOTS('',5,(#24179,#24180,#24181,#24182,#24183,
#24184,#24185,#24186,#24187,#24188,#24189,#24190,#24191,#24192,#24193,#24194,
#24195,#24196,#24197,#24198,#24199,#24200,#24201,#24202,#24203,#24204,#24205,
#24206,#24207,#24208,#24209,#24210,#24211,#24212,#24213,#24214,#24215,#24216,
#24217,#24218,#24219,#24220,#24221,#24222,#24223,#24224,#24225,#24226,#24227,
#24228,#24229,#24230,#24231,#24232,#24233,#24234,#24235,#24236,#24237,#24238,
#24239,#24240,#24241,#24242,#24243,#24244,#24245,#24246,#24247,#24248,#24249,
#24250,#24251,#24252),.UNSPECIFIED.,.F.,.F.,(6,1,1,1,1,1,1,1,1,1,1,1,1,
1,1,1,1,1,1,1,1,1,1,1,1,1,1,1,1,1,1,1,1,1,1,1,1,1,1,1,1,1,1,1,1,1,1,1,1,
1,1,1,1,1,1,1,1,1,1,1,1,1,1,1,1,1,1,1,1,6),(0.,0.0142857142857143,0.0285714285714286,
0.0428571428571429,0.0571428571428571,0.0714285714285714,0.0857142857142857,
0.1,0.114285714285714,0.128571428571429,0.142857142857143,0.157142857142857,
0.171428571428571,0.185714285714286,0.2,0.214285714285714,0.228571428571429,
0.242857142857143,0.257142857142857,0.271428571428571,0.285714285714286,
0.3,0.314285714285714,0.328571428571429,0.342857142857143,0.357142857142857,
0.371428571428571,0.385714285714286,0.4,0.414285714285714,0.428571428571429,
0.442857142857143,0.457142857142857,0.471428571428572,0.485714285714286,
0.5,0.514285714285714,0.528571428571429,0.542857142857143,0.557142857142857,
0.571428571428571,0.585714285714286,0.6,0.614285714285714,0.628571428571428,
0.642857142857142,0.657142857142857,0.671428571428571,0.685714285714285,
0.699999999999999,0.714285714285714,0.728571428571428,0.742857142857142,
0.757142857142856,0.771428571428571,0.785714285714285,0.799999999999999,
0.814285714285713,0.828571428571428,0.842857142857142,0.857142857142856,
0.87142857142857,0.885714285714284,0.899999999999999,0.914285714285713,
0.928571428571427,0.942857142857141,0.957142857142856,0.97142857142857,
1.),.UNSPECIFIED.);
#523=B_SPLINE_CURVE_WITH_KNOTS('',5,(#24404,#24405,#24406,#24407,#24408,
#24409,#24410,#24411,#24412,#24413,#24414,#24415,#24416,#24417,#24418,#24419,
#24420,#24421,#24422,#24423,#24424,#24425,#24426,#24427,#24428,#24429,#24430,
#24431,#24432,#24433,#24434,#24435,#24436,#24437,#24438,#24439,#24440,#24441,
#24442,#24443,#24444,#24445,#24446,#24447,#24448,#24449,#24450,#24451,#24452,
#24453,#24454,#24455,#24456,#24457,#24458,#24459,#24460,#24461,#24462,#24463,
#24464,#24465,#24466,#24467,#24468,#24469,#24470,#24471,#24472,#24473,#24474,
#24475,#24476,#24477),.UNSPECIFIED.,.F.,.F.,(6,1,1,1,1,1,1,1,1,1,1,1,1,
1,1,1,1,1,1,1,1,1,1,1,1,1,1,1,1,1,1,1,1,1,1,1,1,1,1,1,1,1,1,1,1,1,1,1,1,
1,1,1,1,1,1,1,1,1,1,1,1,1,1,1,1,1,1,1,1,6),(0.,0.0142857142857143,0.0285714285714286,
0.0428571428571429,0.0571428571428571,0.0714285714285714,0.0857142857142857,
0.1,0.114285714285714,0.128571428571429,0.142857142857143,0.157142857142857,
0.171428571428571,0.185714285714286,0.2,0.214285714285714,0.228571428571429,
0.242857142857143,0.257142857142857,0.271428571428571,0.285714285714286,
0.3,0.314285714285714,0.328571428571429,0.342857142857143,0.357142857142857,
0.371428571428571,0.385714285714286,0.4,0.414285714285714,0.428571428571429,
0.442857142857143,0.457142857142857,0.471428571428572,0.485714285714286,
0.5,0.514285714285714,0.528571428571429,0.542857142857143,0.557142857142857,
0.571428571428571,0.585714285714286,0.6,0.614285714285714,0.628571428571428,
0.642857142857142,0.657142857142857,0.671428571428571,0.685714285714285,
0.699999999999999,0.714285714285714,0.728571428571428,0.742857142857142,
0.757142857142856,0.771428571428571,0.785714285714285,0.799999999999999,
0.814285714285713,0.828571428571428,0.842857142857142,0.857142857142856,
0.87142857142857,0.885714285714284,0.899999999999999,0.914285714285713,
0.928571428571427,0.942857142857141,0.957142857142856,0.97142857142857,
1.),.UNSPECIFIED.);
#524=B_SPLINE_CURVE_WITH_KNOTS('',5,(#24479,#24480,#24481,#24482,#24483,
#24484,#24485,#24486,#24487,#24488,#24489,#24490,#24491,#24492,#24493,#24494,
#24495,#24496,#24497,#24498,#24499,#24500,#24501,#24502,#24503,#24504,#24505,
#24506,#24507,#24508,#24509,#24510,#24511,#24512,#24513,#24514,#24515,#24516,
#24517,#24518,#24519,#24520,#24521,#24522,#24523,#24524,#24525,#24526,#24527,
#24528,#24529,#24530,#24531,#24532,#24533,#24534,#24535,#24536,#24537,#24538,
#24539,#24540,#24541,#24542,#24543,#24544,#24545,#24546,#24547,#24548,#24549,
#24550,#24551,#24552,#24553),.UNSPECIFIED.,.F.,.F.,(6,1,1,1,1,1,1,1,1,1,
1,1,1,1,1,1,1,1,1,1,1,1,1,1,1,1,1,1,1,1,1,1,1,1,1,1,1,1,1,1,1,1,1,1,1,1,
1,1,1,1,1,1,1,1,1,1,1,1,1,1,1,1,1,1,1,1,1,1,1,1,6),(-1.,-0.985714285714284,
-0.97142857142857,-0.957142857142856,-0.942857142857141,-0.928571428571427,
-0.914285714285713,-0.899999999999999,-0.885714285714284,-0.87142857142857,
-0.857142857142856,-0.842857142857142,-0.828571428571428,-0.814285714285713,
-0.799999999999999,-0.785714285714285,-0.771428571428571,-0.757142857142856,
-0.742857142857142,-0.728571428571428,-0.714285714285714,-0.699999999999999,
-0.685714285714285,-0.671428571428571,-0.657142857142857,-0.642857142857142,
-0.628571428571428,-0.614285714285714,-0.6,-0.585714285714286,-0.571428571428571,
-0.557142857142857,-0.542857142857143,-0.528571428571429,-0.514285714285714,
-0.5,-0.485714285714286,-0.471428571428572,-0.457142857142857,-0.442857142857143,
-0.428571428571429,-0.414285714285714,-0.4,-0.385714285714286,-0.371428571428571,
-0.357142857142857,-0.342857142857143,-0.328571428571429,-0.314285714285714,
-0.3,-0.285714285714286,-0.271428571428571,-0.257142857142857,-0.242857142857143,
-0.228571428571429,-0.214285714285714,-0.2,-0.185714285714286,-0.171428571428571,
-0.157142857142857,-0.142857142857143,-0.128571428571429,-0.114285714285714,
-0.1,-0.0857142857142857,-0.0714285714285714,-0.0571428571428571,-0.0428571428571429,
-0.0285714285714286,-0.0142857142857143,0.),.UNSPECIFIED.);
#525=B_SPLINE_CURVE_WITH_KNOTS('',5,(#24711,#24712,#24713,#24714,#24715,
#24716,#24717,#24718,#24719,#24720,#24721,#24722,#24723,#24724,#24725,#24726,
#24727,#24728,#24729,#24730,#24731,#24732,#24733,#24734,#24735,#24736,#24737,
#24738,#24739,#24740,#24741,#24742,#24743,#24744,#24745,#24746,#24747,#24748,
#24749,#24750,#24751,#24752,#24753,#24754,#24755,#24756,#24757,#24758,#24759,
#24760,#24761,#24762,#24763,#24764,#24765,#24766,#24767,#24768,#24769,#24770,
#24771,#24772,#24773,#24774,#24775,#24776,#24777,#24778,#24779,#24780,#24781,
#24782,#24783,#24784),.UNSPECIFIED.,.F.,.F.,(6,1,1,1,1,1,1,1,1,1,1,1,1,
1,1,1,1,1,1,1,1,1,1,1,1,1,1,1,1,1,1,1,1,1,1,1,1,1,1,1,1,1,1,1,1,1,1,1,1,
1,1,1,1,1,1,1,1,1,1,1,1,1,1,1,1,1,1,1,1,6),(0.,0.0142857142857143,0.0285714285714286,
0.0428571428571429,0.0571428571428571,0.0714285714285714,0.0857142857142857,
0.1,0.114285714285714,0.128571428571429,0.142857142857143,0.157142857142857,
0.171428571428571,0.185714285714286,0.2,0.214285714285714,0.228571428571429,
0.242857142857143,0.257142857142857,0.271428571428571,0.285714285714286,
0.3,0.314285714285714,0.328571428571429,0.342857142857143,0.357142857142857,
0.371428571428571,0.385714285714286,0.4,0.414285714285714,0.428571428571429,
0.442857142857143,0.457142857142857,0.471428571428572,0.485714285714286,
0.5,0.514285714285714,0.528571428571429,0.542857142857143,0.557142857142857,
0.571428571428571,0.585714285714286,0.6,0.614285714285714,0.628571428571428,
0.642857142857142,0.657142857142857,0.671428571428571,0.685714285714285,
0.699999999999999,0.714285714285714,0.728571428571428,0.742857142857142,
0.757142857142856,0.771428571428571,0.785714285714285,0.799999999999999,
0.814285714285713,0.828571428571428,0.842857142857142,0.857142857142856,
0.87142857142857,0.885714285714284,0.899999999999999,0.914285714285713,
0.928571428571427,0.942857142857141,0.957142857142856,0.97142857142857,
1.),.UNSPECIFIED.);
#526=B_SPLINE_CURVE_WITH_KNOTS('',5,(#24785,#24786,#24787,#24788,#24789,
#24790,#24791,#24792,#24793,#24794,#24795,#24796,#24797,#24798,#24799,#24800,
#24801,#24802,#24803,#24804,#24805,#24806,#24807,#24808,#24809,#24810,#24811,
#24812,#24813,#24814,#24815,#24816,#24817,#24818,#24819,#24820,#24821,#24822,
#24823,#24824,#24825,#24826,#24827,#24828,#24829,#24830,#24831,#24832,#24833,
#24834,#24835,#24836,#24837,#24838,#24839,#24840,#24841,#24842,#24843,#24844,
#24845,#24846,#24847,#24848,#24849,#24850,#24851,#24852,#24853,#24854,#24855,
#24856,#24857,#24858),.UNSPECIFIED.,.F.,.F.,(6,1,1,1,1,1,1,1,1,1,1,1,1,
1,1,1,1,1,1,1,1,1,1,1,1,1,1,1,1,1,1,1,1,1,1,1,1,1,1,1,1,1,1,1,1,1,1,1,1,
1,1,1,1,1,1,1,1,1,1,1,1,1,1,1,1,1,1,1,1,6),(0.,0.0142857142857143,0.0285714285714286,
0.0428571428571429,0.0571428571428571,0.0714285714285714,0.0857142857142857,
0.1,0.114285714285714,0.128571428571429,0.142857142857143,0.157142857142857,
0.171428571428571,0.185714285714286,0.2,0.214285714285714,0.228571428571429,
0.242857142857143,0.257142857142857,0.271428571428571,0.285714285714286,
0.3,0.314285714285714,0.328571428571429,0.342857142857143,0.357142857142857,
0.371428571428571,0.385714285714286,0.4,0.414285714285714,0.428571428571429,
0.442857142857143,0.457142857142857,0.471428571428572,0.485714285714286,
0.5,0.514285714285714,0.528571428571429,0.542857142857143,0.557142857142857,
0.571428571428571,0.585714285714286,0.6,0.614285714285714,0.628571428571428,
0.642857142857142,0.657142857142857,0.671428571428571,0.685714285714285,
0.699999999999999,0.714285714285714,0.728571428571428,0.742857142857142,
0.757142857142856,0.771428571428571,0.785714285714285,0.799999999999999,
0.814285714285713,0.828571428571428,0.842857142857142,0.857142857142856,
0.87142857142857,0.885714285714284,0.899999999999999,0.914285714285713,
0.928571428571427,0.942857142857141,0.957142857142856,0.97142857142857,
1.),.UNSPECIFIED.);
#527=B_SPLINE_CURVE_WITH_KNOTS('',5,(#25010,#25011,#25012,#25013,#25014,
#25015,#25016,#25017,#25018,#25019,#25020,#25021,#25022,#25023,#25024,#25025,
#25026,#25027,#25028,#25029,#25030,#25031,#25032,#25033,#25034,#25035,#25036,
#25037,#25038,#25039,#25040,#25041,#25042,#25043,#25044,#25045,#25046,#25047,
#25048,#25049,#25050,#25051,#25052,#25053,#25054,#25055,#25056,#25057,#25058,
#25059,#25060,#25061,#25062,#25063,#25064,#25065,#25066,#25067,#25068,#25069,
#25070,#25071,#25072,#25073,#25074,#25075,#25076,#25077,#25078,#25079,#25080,
#25081,#25082,#25083),.UNSPECIFIED.,.F.,.F.,(6,1,1,1,1,1,1,1,1,1,1,1,1,
1,1,1,1,1,1,1,1,1,1,1,1,1,1,1,1,1,1,1,1,1,1,1,1,1,1,1,1,1,1,1,1,1,1,1,1,
1,1,1,1,1,1,1,1,1,1,1,1,1,1,1,1,1,1,1,1,6),(0.,0.0142857142857143,0.0285714285714286,
0.0428571428571429,0.0571428571428571,0.0714285714285714,0.0857142857142857,
0.1,0.114285714285714,0.128571428571429,0.142857142857143,0.157142857142857,
0.171428571428571,0.185714285714286,0.2,0.214285714285714,0.228571428571429,
0.242857142857143,0.257142857142857,0.271428571428571,0.285714285714286,
0.3,0.314285714285714,0.328571428571429,0.342857142857143,0.357142857142857,
0.371428571428571,0.385714285714286,0.4,0.414285714285714,0.428571428571429,
0.442857142857143,0.457142857142857,0.471428571428572,0.485714285714286,
0.5,0.514285714285714,0.528571428571429,0.542857142857143,0.557142857142857,
0.571428571428571,0.585714285714286,0.6,0.614285714285714,0.628571428571428,
0.642857142857142,0.657142857142857,0.671428571428571,0.685714285714285,
0.699999999999999,0.714285714285714,0.728571428571428,0.742857142857142,
0.757142857142856,0.771428571428571,0.785714285714285,0.799999999999999,
0.814285714285713,0.828571428571428,0.842857142857142,0.857142857142856,
0.87142857142857,0.885714285714284,0.899999999999999,0.914285714285713,
0.928571428571427,0.942857142857141,0.957142857142856,0.97142857142857,
1.),.UNSPECIFIED.);
#528=B_SPLINE_CURVE_WITH_KNOTS('',5,(#25085,#25086,#25087,#25088,#25089,
#25090,#25091,#25092,#25093,#25094,#25095,#25096,#25097,#25098,#25099,#25100,
#25101,#25102,#25103,#25104,#25105,#25106,#25107,#25108,#25109,#25110,#25111,
#25112,#25113,#25114,#25115,#25116,#25117,#25118,#25119,#25120,#25121,#25122,
#25123,#25124,#25125,#25126,#25127,#25128,#25129,#25130,#25131,#25132,#25133,
#25134,#25135,#25136,#25137,#25138,#25139,#25140,#25141,#25142,#25143,#25144,
#25145,#25146,#25147,#25148,#25149,#25150,#25151,#25152,#25153,#25154,#25155,
#25156,#25157,#25158,#25159),.UNSPECIFIED.,.F.,.F.,(6,1,1,1,1,1,1,1,1,1,
1,1,1,1,1,1,1,1,1,1,1,1,1,1,1,1,1,1,1,1,1,1,1,1,1,1,1,1,1,1,1,1,1,1,1,1,
1,1,1,1,1,1,1,1,1,1,1,1,1,1,1,1,1,1,1,1,1,1,1,1,6),(-1.,-0.985714285714284,
-0.97142857142857,-0.957142857142856,-0.942857142857141,-0.928571428571427,
-0.914285714285713,-0.899999999999999,-0.885714285714284,-0.87142857142857,
-0.857142857142856,-0.842857142857142,-0.828571428571428,-0.814285714285713,
-0.799999999999999,-0.785714285714285,-0.771428571428571,-0.757142857142856,
-0.742857142857142,-0.728571428571428,-0.714285714285714,-0.699999999999999,
-0.685714285714285,-0.671428571428571,-0.657142857142857,-0.642857142857142,
-0.628571428571428,-0.614285714285714,-0.6,-0.585714285714286,-0.571428571428571,
-0.557142857142857,-0.542857142857143,-0.528571428571429,-0.514285714285714,
-0.5,-0.485714285714286,-0.471428571428572,-0.457142857142857,-0.442857142857143,
-0.428571428571429,-0.414285714285714,-0.4,-0.385714285714286,-0.371428571428571,
-0.357142857142857,-0.342857142857143,-0.328571428571429,-0.314285714285714,
-0.3,-0.285714285714286,-0.271428571428571,-0.257142857142857,-0.242857142857143,
-0.228571428571429,-0.214285714285714,-0.2,-0.185714285714286,-0.171428571428571,
-0.157142857142857,-0.142857142857143,-0.128571428571429,-0.114285714285714,
-0.1,-0.0857142857142857,-0.0714285714285714,-0.0571428571428571,-0.0428571428571429,
-0.0285714285714286,-0.0142857142857143,0.),.UNSPECIFIED.);
#529=B_SPLINE_CURVE_WITH_KNOTS('',5,(#25317,#25318,#25319,#25320,#25321,
#25322,#25323,#25324,#25325,#25326,#25327,#25328,#25329,#25330,#25331,#25332,
#25333,#25334,#25335,#25336,#25337,#25338,#25339,#25340,#25341,#25342,#25343,
#25344,#25345,#25346,#25347,#25348,#25349,#25350,#25351,#25352,#25353,#25354,
#25355,#25356,#25357,#25358,#25359,#25360,#25361,#25362,#25363,#25364,#25365,
#25366,#25367,#25368,#25369,#25370,#25371,#25372,#25373,#25374,#25375,#25376,
#25377,#25378,#25379,#25380,#25381,#25382,#25383,#25384,#25385,#25386,#25387,
#25388,#25389,#25390),.UNSPECIFIED.,.F.,.F.,(6,1,1,1,1,1,1,1,1,1,1,1,1,
1,1,1,1,1,1,1,1,1,1,1,1,1,1,1,1,1,1,1,1,1,1,1,1,1,1,1,1,1,1,1,1,1,1,1,1,
1,1,1,1,1,1,1,1,1,1,1,1,1,1,1,1,1,1,1,1,6),(0.,0.0142857142857143,0.0285714285714286,
0.0428571428571429,0.0571428571428571,0.0714285714285714,0.0857142857142857,
0.1,0.114285714285714,0.128571428571429,0.142857142857143,0.157142857142857,
0.171428571428571,0.185714285714286,0.2,0.214285714285714,0.228571428571429,
0.242857142857143,0.257142857142857,0.271428571428571,0.285714285714286,
0.3,0.314285714285714,0.328571428571429,0.342857142857143,0.357142857142857,
0.371428571428571,0.385714285714286,0.4,0.414285714285714,0.428571428571429,
0.442857142857143,0.457142857142857,0.471428571428572,0.485714285714286,
0.5,0.514285714285714,0.528571428571429,0.542857142857143,0.557142857142857,
0.571428571428571,0.585714285714286,0.6,0.614285714285714,0.628571428571428,
0.642857142857142,0.657142857142857,0.671428571428571,0.685714285714285,
0.699999999999999,0.714285714285714,0.728571428571428,0.742857142857142,
0.757142857142856,0.771428571428571,0.785714285714285,0.799999999999999,
0.814285714285713,0.828571428571428,0.842857142857142,0.857142857142856,
0.87142857142857,0.885714285714284,0.899999999999999,0.914285714285713,
0.928571428571427,0.942857142857141,0.957142857142856,0.97142857142857,
1.),.UNSPECIFIED.);
#530=B_SPLINE_CURVE_WITH_KNOTS('',5,(#25391,#25392,#25393,#25394,#25395,
#25396,#25397,#25398,#25399,#25400,#25401,#25402,#25403,#25404,#25405,#25406,
#25407,#25408,#25409,#25410,#25411,#25412,#25413,#25414,#25415,#25416,#25417,
#25418,#25419,#25420,#25421,#25422,#25423,#25424,#25425,#25426,#25427,#25428,
#25429,#25430,#25431,#25432,#25433,#25434,#25435,#25436,#25437,#25438,#25439,
#25440,#25441,#25442,#25443,#25444,#25445,#25446,#25447,#25448,#25449,#25450,
#25451,#25452,#25453,#25454,#25455,#25456,#25457,#25458,#25459,#25460,#25461,
#25462,#25463,#25464),.UNSPECIFIED.,.F.,.F.,(6,1,1,1,1,1,1,1,1,1,1,1,1,
1,1,1,1,1,1,1,1,1,1,1,1,1,1,1,1,1,1,1,1,1,1,1,1,1,1,1,1,1,1,1,1,1,1,1,1,
1,1,1,1,1,1,1,1,1,1,1,1,1,1,1,1,1,1,1,1,6),(0.,0.0142857142857143,0.0285714285714286,
0.0428571428571429,0.0571428571428571,0.0714285714285714,0.0857142857142857,
0.1,0.114285714285714,0.128571428571429,0.142857142857143,0.157142857142857,
0.171428571428571,0.185714285714286,0.2,0.214285714285714,0.228571428571429,
0.242857142857143,0.257142857142857,0.271428571428571,0.285714285714286,
0.3,0.314285714285714,0.328571428571429,0.342857142857143,0.357142857142857,
0.371428571428571,0.385714285714286,0.4,0.414285714285714,0.428571428571429,
0.442857142857143,0.457142857142857,0.471428571428572,0.485714285714286,
0.5,0.514285714285714,0.528571428571429,0.542857142857143,0.557142857142857,
0.571428571428571,0.585714285714286,0.6,0.614285714285714,0.628571428571428,
0.642857142857142,0.657142857142857,0.671428571428571,0.685714285714285,
0.699999999999999,0.714285714285714,0.728571428571428,0.742857142857142,
0.757142857142856,0.771428571428571,0.785714285714285,0.799999999999999,
0.814285714285713,0.828571428571428,0.842857142857142,0.857142857142856,
0.87142857142857,0.885714285714284,0.899999999999999,0.914285714285713,
0.928571428571427,0.942857142857141,0.957142857142856,0.97142857142857,
1.),.UNSPECIFIED.);
#531=B_SPLINE_CURVE_WITH_KNOTS('',5,(#25616,#25617,#25618,#25619,#25620,
#25621,#25622,#25623,#25624,#25625,#25626,#25627,#25628,#25629,#25630,#25631,
#25632,#25633,#25634,#25635,#25636,#25637,#25638,#25639,#25640,#25641,#25642,
#25643,#25644,#25645,#25646,#25647,#25648,#25649,#25650,#25651,#25652,#25653,
#25654,#25655,#25656,#25657,#25658,#25659,#25660,#25661,#25662,#25663,#25664,
#25665,#25666,#25667,#25668,#25669,#25670,#25671,#25672,#25673,#25674,#25675,
#25676,#25677,#25678,#25679,#25680,#25681,#25682,#25683,#25684,#25685,#25686,
#25687,#25688,#25689),.UNSPECIFIED.,.F.,.F.,(6,1,1,1,1,1,1,1,1,1,1,1,1,
1,1,1,1,1,1,1,1,1,1,1,1,1,1,1,1,1,1,1,1,1,1,1,1,1,1,1,1,1,1,1,1,1,1,1,1,
1,1,1,1,1,1,1,1,1,1,1,1,1,1,1,1,1,1,1,1,6),(0.,0.0142857142857143,0.0285714285714286,
0.0428571428571429,0.0571428571428571,0.0714285714285714,0.0857142857142857,
0.1,0.114285714285714,0.128571428571429,0.142857142857143,0.157142857142857,
0.171428571428571,0.185714285714286,0.2,0.214285714285714,0.228571428571429,
0.242857142857143,0.257142857142857,0.271428571428571,0.285714285714286,
0.3,0.314285714285714,0.328571428571429,0.342857142857143,0.357142857142857,
0.371428571428571,0.385714285714286,0.4,0.414285714285714,0.428571428571429,
0.442857142857143,0.457142857142857,0.471428571428572,0.485714285714286,
0.5,0.514285714285714,0.528571428571429,0.542857142857143,0.557142857142857,
0.571428571428571,0.585714285714286,0.6,0.614285714285714,0.628571428571428,
0.642857142857142,0.657142857142857,0.671428571428571,0.685714285714285,
0.699999999999999,0.714285714285714,0.728571428571428,0.742857142857142,
0.757142857142856,0.771428571428571,0.785714285714285,0.799999999999999,
0.814285714285713,0.828571428571428,0.842857142857142,0.857142857142856,
0.87142857142857,0.885714285714284,0.899999999999999,0.914285714285713,
0.928571428571427,0.942857142857141,0.957142857142856,0.97142857142857,
1.),.UNSPECIFIED.);
#532=B_SPLINE_CURVE_WITH_KNOTS('',5,(#25691,#25692,#25693,#25694,#25695,
#25696,#25697,#25698,#25699,#25700,#25701,#25702,#25703,#25704,#25705,#25706,
#25707,#25708,#25709,#25710,#25711,#25712,#25713,#25714,#25715,#25716,#25717,
#25718,#25719,#25720,#25721,#25722,#25723,#25724,#25725,#25726,#25727,#25728,
#25729,#25730,#25731,#25732,#25733,#25734,#25735,#25736,#25737,#25738,#25739,
#25740,#25741,#25742,#25743,#25744,#25745,#25746,#25747,#25748,#25749,#25750,
#25751,#25752,#25753,#25754,#25755,#25756,#25757,#25758,#25759,#25760,#25761,
#25762,#25763,#25764,#25765),.UNSPECIFIED.,.F.,.F.,(6,1,1,1,1,1,1,1,1,1,
1,1,1,1,1,1,1,1,1,1,1,1,1,1,1,1,1,1,1,1,1,1,1,1,1,1,1,1,1,1,1,1,1,1,1,1,
1,1,1,1,1,1,1,1,1,1,1,1,1,1,1,1,1,1,1,1,1,1,1,1,6),(-1.,-0.985714285714284,
-0.97142857142857,-0.957142857142856,-0.942857142857141,-0.928571428571427,
-0.914285714285713,-0.899999999999999,-0.885714285714284,-0.87142857142857,
-0.857142857142856,-0.842857142857142,-0.828571428571428,-0.814285714285713,
-0.799999999999999,-0.785714285714285,-0.771428571428571,-0.757142857142856,
-0.742857142857142,-0.728571428571428,-0.714285714285714,-0.699999999999999,
-0.685714285714285,-0.671428571428571,-0.657142857142857,-0.642857142857142,
-0.628571428571428,-0.614285714285714,-0.6,-0.585714285714286,-0.571428571428571,
-0.557142857142857,-0.542857142857143,-0.528571428571429,-0.514285714285714,
-0.5,-0.485714285714286,-0.471428571428572,-0.457142857142857,-0.442857142857143,
-0.428571428571429,-0.414285714285714,-0.4,-0.385714285714286,-0.371428571428571,
-0.357142857142857,-0.342857142857143,-0.328571428571429,-0.314285714285714,
-0.3,-0.285714285714286,-0.271428571428571,-0.257142857142857,-0.242857142857143,
-0.228571428571429,-0.214285714285714,-0.2,-0.185714285714286,-0.171428571428571,
-0.157142857142857,-0.142857142857143,-0.128571428571429,-0.114285714285714,
-0.1,-0.0857142857142857,-0.0714285714285714,-0.0571428571428571,-0.0428571428571429,
-0.0285714285714286,-0.0142857142857143,0.),.UNSPECIFIED.);
#533=B_SPLINE_CURVE_WITH_KNOTS('',5,(#25923,#25924,#25925,#25926,#25927,
#25928,#25929,#25930,#25931,#25932,#25933,#25934,#25935,#25936,#25937,#25938,
#25939,#25940,#25941,#25942,#25943,#25944,#25945,#25946,#25947,#25948,#25949,
#25950,#25951,#25952,#25953,#25954,#25955,#25956,#25957,#25958,#25959,#25960,
#25961,#25962,#25963,#25964,#25965,#25966,#25967,#25968,#25969,#25970,#25971,
#25972,#25973,#25974,#25975,#25976,#25977,#25978,#25979,#25980,#25981,#25982,
#25983,#25984,#25985,#25986,#25987,#25988,#25989,#25990,#25991,#25992,#25993,
#25994,#25995,#25996),.UNSPECIFIED.,.F.,.F.,(6,1,1,1,1,1,1,1,1,1,1,1,1,
1,1,1,1,1,1,1,1,1,1,1,1,1,1,1,1,1,1,1,1,1,1,1,1,1,1,1,1,1,1,1,1,1,1,1,1,
1,1,1,1,1,1,1,1,1,1,1,1,1,1,1,1,1,1,1,1,6),(0.,0.0142857142857143,0.0285714285714286,
0.0428571428571429,0.0571428571428571,0.0714285714285714,0.0857142857142857,
0.1,0.114285714285714,0.128571428571429,0.142857142857143,0.157142857142857,
0.171428571428571,0.185714285714286,0.2,0.214285714285714,0.228571428571429,
0.242857142857143,0.257142857142857,0.271428571428571,0.285714285714286,
0.3,0.314285714285714,0.328571428571429,0.342857142857143,0.357142857142857,
0.371428571428571,0.385714285714286,0.4,0.414285714285714,0.428571428571429,
0.442857142857143,0.457142857142857,0.471428571428572,0.485714285714286,
0.5,0.514285714285714,0.528571428571429,0.542857142857143,0.557142857142857,
0.571428571428571,0.585714285714286,0.6,0.614285714285714,0.628571428571428,
0.642857142857142,0.657142857142857,0.671428571428571,0.685714285714285,
0.699999999999999,0.714285714285714,0.728571428571428,0.742857142857142,
0.757142857142856,0.771428571428571,0.785714285714285,0.799999999999999,
0.814285714285713,0.828571428571428,0.842857142857142,0.857142857142856,
0.87142857142857,0.885714285714284,0.899999999999999,0.914285714285713,
0.928571428571427,0.942857142857141,0.957142857142856,0.97142857142857,
1.),.UNSPECIFIED.);
#534=B_SPLINE_CURVE_WITH_KNOTS('',5,(#25997,#25998,#25999,#26000,#26001,
#26002,#26003,#26004,#26005,#26006,#26007,#26008,#26009,#26010,#26011,#26012,
#26013,#26014,#26015,#26016,#26017,#26018,#26019,#26020,#26021,#26022,#26023,
#26024,#26025,#26026,#26027,#26028,#26029,#26030,#26031,#26032,#26033,#26034,
#26035,#26036,#26037,#26038,#26039,#26040,#26041,#26042,#26043,#26044,#26045,
#26046,#26047,#26048,#26049,#26050,#26051,#26052,#26053,#26054,#26055,#26056,
#26057,#26058,#26059,#26060,#26061,#26062,#26063,#26064,#26065,#26066,#26067,
#26068,#26069,#26070),.UNSPECIFIED.,.F.,.F.,(6,1,1,1,1,1,1,1,1,1,1,1,1,
1,1,1,1,1,1,1,1,1,1,1,1,1,1,1,1,1,1,1,1,1,1,1,1,1,1,1,1,1,1,1,1,1,1,1,1,
1,1,1,1,1,1,1,1,1,1,1,1,1,1,1,1,1,1,1,1,6),(0.,0.0142857142857143,0.0285714285714286,
0.0428571428571429,0.0571428571428571,0.0714285714285714,0.0857142857142857,
0.1,0.114285714285714,0.128571428571429,0.142857142857143,0.157142857142857,
0.171428571428571,0.185714285714286,0.2,0.214285714285714,0.228571428571429,
0.242857142857143,0.257142857142857,0.271428571428571,0.285714285714286,
0.3,0.314285714285714,0.328571428571429,0.342857142857143,0.357142857142857,
0.371428571428571,0.385714285714286,0.4,0.414285714285714,0.428571428571429,
0.442857142857143,0.457142857142857,0.471428571428572,0.485714285714286,
0.5,0.514285714285714,0.528571428571429,0.542857142857143,0.557142857142857,
0.571428571428571,0.585714285714286,0.6,0.614285714285714,0.628571428571428,
0.642857142857142,0.657142857142857,0.671428571428571,0.685714285714285,
0.699999999999999,0.714285714285714,0.728571428571428,0.742857142857142,
0.757142857142856,0.771428571428571,0.785714285714285,0.799999999999999,
0.814285714285713,0.828571428571428,0.842857142857142,0.857142857142856,
0.87142857142857,0.885714285714284,0.899999999999999,0.914285714285713,
0.928571428571427,0.942857142857141,0.957142857142856,0.97142857142857,
1.),.UNSPECIFIED.);
#535=B_SPLINE_CURVE_WITH_KNOTS('',5,(#26222,#26223,#26224,#26225,#26226,
#26227,#26228,#26229,#26230,#26231,#26232,#26233,#26234,#26235,#26236,#26237,
#26238,#26239,#26240,#26241,#26242,#26243,#26244,#26245,#26246,#26247,#26248,
#26249,#26250,#26251,#26252,#26253,#26254,#26255,#26256,#26257,#26258,#26259,
#26260,#26261,#26262,#26263,#26264,#26265,#26266,#26267,#26268,#26269,#26270,
#26271,#26272,#26273,#26274,#26275,#26276,#26277,#26278,#26279,#26280,#26281,
#26282,#26283,#26284,#26285,#26286,#26287,#26288,#26289,#26290,#26291,#26292,
#26293,#26294,#26295),.UNSPECIFIED.,.F.,.F.,(6,1,1,1,1,1,1,1,1,1,1,1,1,
1,1,1,1,1,1,1,1,1,1,1,1,1,1,1,1,1,1,1,1,1,1,1,1,1,1,1,1,1,1,1,1,1,1,1,1,
1,1,1,1,1,1,1,1,1,1,1,1,1,1,1,1,1,1,1,1,6),(0.,0.0142857142857143,0.0285714285714286,
0.0428571428571429,0.0571428571428571,0.0714285714285714,0.0857142857142857,
0.1,0.114285714285714,0.128571428571429,0.142857142857143,0.157142857142857,
0.171428571428571,0.185714285714286,0.2,0.214285714285714,0.228571428571429,
0.242857142857143,0.257142857142857,0.271428571428571,0.285714285714286,
0.3,0.314285714285714,0.328571428571429,0.342857142857143,0.357142857142857,
0.371428571428571,0.385714285714286,0.4,0.414285714285714,0.428571428571429,
0.442857142857143,0.457142857142857,0.471428571428572,0.485714285714286,
0.5,0.514285714285714,0.528571428571429,0.542857142857143,0.557142857142857,
0.571428571428571,0.585714285714286,0.6,0.614285714285714,0.628571428571428,
0.642857142857142,0.657142857142857,0.671428571428571,0.685714285714285,
0.699999999999999,0.714285714285714,0.728571428571428,0.742857142857142,
0.757142857142856,0.771428571428571,0.785714285714285,0.799999999999999,
0.814285714285713,0.828571428571428,0.842857142857142,0.857142857142856,
0.87142857142857,0.885714285714284,0.899999999999999,0.914285714285713,
0.928571428571427,0.942857142857141,0.957142857142856,0.97142857142857,
1.),.UNSPECIFIED.);
#536=B_SPLINE_CURVE_WITH_KNOTS('',5,(#26297,#26298,#26299,#26300,#26301,
#26302,#26303,#26304,#26305,#26306,#26307,#26308,#26309,#26310,#26311,#26312,
#26313,#26314,#26315,#26316,#26317,#26318,#26319,#26320,#26321,#26322,#26323,
#26324,#26325,#26326,#26327,#26328,#26329,#26330,#26331,#26332,#26333,#26334,
#26335,#26336,#26337,#26338,#26339,#26340,#26341,#26342,#26343,#26344,#26345,
#26346,#26347,#26348,#26349,#26350,#26351,#26352,#26353,#26354,#26355,#26356,
#26357,#26358,#26359,#26360,#26361,#26362,#26363,#26364,#26365,#26366,#26367,
#26368,#26369,#26370,#26371),.UNSPECIFIED.,.F.,.F.,(6,1,1,1,1,1,1,1,1,1,
1,1,1,1,1,1,1,1,1,1,1,1,1,1,1,1,1,1,1,1,1,1,1,1,1,1,1,1,1,1,1,1,1,1,1,1,
1,1,1,1,1,1,1,1,1,1,1,1,1,1,1,1,1,1,1,1,1,1,1,1,6),(-1.,-0.985714285714284,
-0.97142857142857,-0.957142857142856,-0.942857142857141,-0.928571428571427,
-0.914285714285713,-0.899999999999999,-0.885714285714284,-0.87142857142857,
-0.857142857142856,-0.842857142857142,-0.828571428571428,-0.814285714285713,
-0.799999999999999,-0.785714285714285,-0.771428571428571,-0.757142857142856,
-0.742857142857142,-0.728571428571428,-0.714285714285714,-0.699999999999999,
-0.685714285714285,-0.671428571428571,-0.657142857142857,-0.642857142857142,
-0.628571428571428,-0.614285714285714,-0.6,-0.585714285714286,-0.571428571428571,
-0.557142857142857,-0.542857142857143,-0.528571428571429,-0.514285714285714,
-0.5,-0.485714285714286,-0.471428571428572,-0.457142857142857,-0.442857142857143,
-0.428571428571429,-0.414285714285714,-0.4,-0.385714285714286,-0.371428571428571,
-0.357142857142857,-0.342857142857143,-0.328571428571429,-0.314285714285714,
-0.3,-0.285714285714286,-0.271428571428571,-0.257142857142857,-0.242857142857143,
-0.228571428571429,-0.214285714285714,-0.2,-0.185714285714286,-0.171428571428571,
-0.157142857142857,-0.142857142857143,-0.128571428571429,-0.114285714285714,
-0.1,-0.0857142857142857,-0.0714285714285714,-0.0571428571428571,-0.0428571428571429,
-0.0285714285714286,-0.0142857142857143,0.),.UNSPECIFIED.);
#537=B_SPLINE_CURVE_WITH_KNOTS('',5,(#26529,#26530,#26531,#26532,#26533,
#26534,#26535,#26536,#26537,#26538,#26539,#26540,#26541,#26542,#26543,#26544,
#26545,#26546,#26547,#26548,#26549,#26550,#26551,#26552,#26553,#26554,#26555,
#26556,#26557,#26558,#26559,#26560,#26561,#26562,#26563,#26564,#26565,#26566,
#26567,#26568,#26569,#26570,#26571,#26572,#26573,#26574,#26575,#26576,#26577,
#26578,#26579,#26580,#26581,#26582,#26583,#26584,#26585,#26586,#26587,#26588,
#26589,#26590,#26591,#26592,#26593,#26594,#26595,#26596,#26597,#26598,#26599,
#26600,#26601,#26602),.UNSPECIFIED.,.F.,.F.,(6,1,1,1,1,1,1,1,1,1,1,1,1,
1,1,1,1,1,1,1,1,1,1,1,1,1,1,1,1,1,1,1,1,1,1,1,1,1,1,1,1,1,1,1,1,1,1,1,1,
1,1,1,1,1,1,1,1,1,1,1,1,1,1,1,1,1,1,1,1,6),(0.,0.0142857142857143,0.0285714285714286,
0.0428571428571429,0.0571428571428571,0.0714285714285714,0.0857142857142857,
0.1,0.114285714285714,0.128571428571429,0.142857142857143,0.157142857142857,
0.171428571428571,0.185714285714286,0.2,0.214285714285714,0.228571428571429,
0.242857142857143,0.257142857142857,0.271428571428571,0.285714285714286,
0.3,0.314285714285714,0.328571428571429,0.342857142857143,0.357142857142857,
0.371428571428571,0.385714285714286,0.4,0.414285714285714,0.428571428571429,
0.442857142857143,0.457142857142857,0.471428571428572,0.485714285714286,
0.5,0.514285714285714,0.528571428571429,0.542857142857143,0.557142857142857,
0.571428571428571,0.585714285714286,0.6,0.614285714285714,0.628571428571428,
0.642857142857142,0.657142857142857,0.671428571428571,0.685714285714285,
0.699999999999999,0.714285714285714,0.728571428571428,0.742857142857142,
0.757142857142856,0.771428571428571,0.785714285714285,0.799999999999999,
0.814285714285713,0.828571428571428,0.842857142857142,0.857142857142856,
0.87142857142857,0.885714285714284,0.899999999999999,0.914285714285713,
0.928571428571427,0.942857142857141,0.957142857142856,0.97142857142857,
1.),.UNSPECIFIED.);
#538=B_SPLINE_CURVE_WITH_KNOTS('',5,(#26603,#26604,#26605,#26606,#26607,
#26608,#26609,#26610,#26611,#26612,#26613,#26614,#26615,#26616,#26617,#26618,
#26619,#26620,#26621,#26622,#26623,#26624,#26625,#26626,#26627,#26628,#26629,
#26630,#26631,#26632,#26633,#26634,#26635,#26636,#26637,#26638,#26639,#26640,
#26641,#26642,#26643,#26644,#26645,#26646,#26647,#26648,#26649,#26650,#26651,
#26652,#26653,#26654,#26655,#26656,#26657,#26658,#26659,#26660,#26661,#26662,
#26663,#26664,#26665,#26666,#26667,#26668,#26669,#26670,#26671,#26672,#26673,
#26674,#26675,#26676),.UNSPECIFIED.,.F.,.F.,(6,1,1,1,1,1,1,1,1,1,1,1,1,
1,1,1,1,1,1,1,1,1,1,1,1,1,1,1,1,1,1,1,1,1,1,1,1,1,1,1,1,1,1,1,1,1,1,1,1,
1,1,1,1,1,1,1,1,1,1,1,1,1,1,1,1,1,1,1,1,6),(0.,0.0142857142857143,0.0285714285714286,
0.0428571428571429,0.0571428571428571,0.0714285714285714,0.0857142857142857,
0.1,0.114285714285714,0.128571428571429,0.142857142857143,0.157142857142857,
0.171428571428571,0.185714285714286,0.2,0.214285714285714,0.228571428571429,
0.242857142857143,0.257142857142857,0.271428571428571,0.285714285714286,
0.3,0.314285714285714,0.328571428571429,0.342857142857143,0.357142857142857,
0.371428571428571,0.385714285714286,0.4,0.414285714285714,0.428571428571429,
0.442857142857143,0.457142857142857,0.471428571428572,0.485714285714286,
0.5,0.514285714285714,0.528571428571429,0.542857142857143,0.557142857142857,
0.571428571428571,0.585714285714286,0.6,0.614285714285714,0.628571428571428,
0.642857142857142,0.657142857142857,0.671428571428571,0.685714285714285,
0.699999999999999,0.714285714285714,0.728571428571428,0.742857142857142,
0.757142857142856,0.771428571428571,0.785714285714285,0.799999999999999,
0.814285714285713,0.828571428571428,0.842857142857142,0.857142857142856,
0.87142857142857,0.885714285714284,0.899999999999999,0.914285714285713,
0.928571428571427,0.942857142857141,0.957142857142856,0.97142857142857,
1.),.UNSPECIFIED.);
#539=B_SPLINE_CURVE_WITH_KNOTS('',5,(#26828,#26829,#26830,#26831,#26832,
#26833,#26834,#26835,#26836,#26837,#26838,#26839,#26840,#26841,#26842,#26843,
#26844,#26845,#26846,#26847,#26848,#26849,#26850,#26851,#26852,#26853,#26854,
#26855,#26856,#26857,#26858,#26859,#26860,#26861,#26862,#26863,#26864,#26865,
#26866,#26867,#26868,#26869,#26870,#26871,#26872,#26873,#26874,#26875,#26876,
#26877,#26878,#26879,#26880,#26881,#26882,#26883,#26884,#26885,#26886,#26887,
#26888,#26889,#26890,#26891,#26892,#26893,#26894,#26895,#26896,#26897,#26898,
#26899,#26900,#26901),.UNSPECIFIED.,.F.,.F.,(6,1,1,1,1,1,1,1,1,1,1,1,1,
1,1,1,1,1,1,1,1,1,1,1,1,1,1,1,1,1,1,1,1,1,1,1,1,1,1,1,1,1,1,1,1,1,1,1,1,
1,1,1,1,1,1,1,1,1,1,1,1,1,1,1,1,1,1,1,1,6),(0.,0.0142857142857143,0.0285714285714286,
0.0428571428571429,0.0571428571428571,0.0714285714285714,0.0857142857142857,
0.1,0.114285714285714,0.128571428571429,0.142857142857143,0.157142857142857,
0.171428571428571,0.185714285714286,0.2,0.214285714285714,0.228571428571429,
0.242857142857143,0.257142857142857,0.271428571428571,0.285714285714286,
0.3,0.314285714285714,0.328571428571429,0.342857142857143,0.357142857142857,
0.371428571428571,0.385714285714286,0.4,0.414285714285714,0.428571428571429,
0.442857142857143,0.457142857142857,0.471428571428572,0.485714285714286,
0.5,0.514285714285714,0.528571428571429,0.542857142857143,0.557142857142857,
0.571428571428571,0.585714285714286,0.6,0.614285714285714,0.628571428571428,
0.642857142857142,0.657142857142857,0.671428571428571,0.685714285714285,
0.699999999999999,0.714285714285714,0.728571428571428,0.742857142857142,
0.757142857142856,0.771428571428571,0.785714285714285,0.799999999999999,
0.814285714285713,0.828571428571428,0.842857142857142,0.857142857142856,
0.87142857142857,0.885714285714284,0.899999999999999,0.914285714285713,
0.928571428571427,0.942857142857141,0.957142857142856,0.97142857142857,
1.),.UNSPECIFIED.);
#540=B_SPLINE_CURVE_WITH_KNOTS('',5,(#26903,#26904,#26905,#26906,#26907,
#26908,#26909,#26910,#26911,#26912,#26913,#26914,#26915,#26916,#26917,#26918,
#26919,#26920,#26921,#26922,#26923,#26924,#26925,#26926,#26927,#26928,#26929,
#26930,#26931,#26932,#26933,#26934,#26935,#26936,#26937,#26938,#26939,#26940,
#26941,#26942,#26943,#26944,#26945,#26946,#26947,#26948,#26949,#26950,#26951,
#26952,#26953,#26954,#26955,#26956,#26957,#26958,#26959,#26960,#26961,#26962,
#26963,#26964,#26965,#26966,#26967,#26968,#26969,#26970,#26971,#26972,#26973,
#26974,#26975,#26976,#26977),.UNSPECIFIED.,.F.,.F.,(6,1,1,1,1,1,1,1,1,1,
1,1,1,1,1,1,1,1,1,1,1,1,1,1,1,1,1,1,1,1,1,1,1,1,1,1,1,1,1,1,1,1,1,1,1,1,
1,1,1,1,1,1,1,1,1,1,1,1,1,1,1,1,1,1,1,1,1,1,1,1,6),(-1.,-0.985714285714284,
-0.97142857142857,-0.957142857142856,-0.942857142857141,-0.928571428571427,
-0.914285714285713,-0.899999999999999,-0.885714285714284,-0.87142857142857,
-0.857142857142856,-0.842857142857142,-0.828571428571428,-0.814285714285713,
-0.799999999999999,-0.785714285714285,-0.771428571428571,-0.757142857142856,
-0.742857142857142,-0.728571428571428,-0.714285714285714,-0.699999999999999,
-0.685714285714285,-0.671428571428571,-0.657142857142857,-0.642857142857142,
-0.628571428571428,-0.614285714285714,-0.6,-0.585714285714286,-0.571428571428571,
-0.557142857142857,-0.542857142857143,-0.528571428571429,-0.514285714285714,
-0.5,-0.485714285714286,-0.471428571428572,-0.457142857142857,-0.442857142857143,
-0.428571428571429,-0.414285714285714,-0.4,-0.385714285714286,-0.371428571428571,
-0.357142857142857,-0.342857142857143,-0.328571428571429,-0.314285714285714,
-0.3,-0.285714285714286,-0.271428571428571,-0.257142857142857,-0.242857142857143,
-0.228571428571429,-0.214285714285714,-0.2,-0.185714285714286,-0.171428571428571,
-0.157142857142857,-0.142857142857143,-0.128571428571429,-0.114285714285714,
-0.1,-0.0857142857142857,-0.0714285714285714,-0.0571428571428571,-0.0428571428571429,
-0.0285714285714286,-0.0142857142857143,0.),.UNSPECIFIED.);
#541=B_SPLINE_CURVE_WITH_KNOTS('',5,(#27135,#27136,#27137,#27138,#27139,
#27140,#27141,#27142,#27143,#27144,#27145,#27146,#27147,#27148,#27149,#27150,
#27151,#27152,#27153,#27154,#27155,#27156,#27157,#27158,#27159,#27160,#27161,
#27162,#27163,#27164,#27165,#27166,#27167,#27168,#27169,#27170,#27171,#27172,
#27173,#27174,#27175,#27176,#27177,#27178,#27179,#27180,#27181,#27182,#27183,
#27184,#27185,#27186,#27187,#27188,#27189,#27190,#27191,#27192,#27193,#27194,
#27195,#27196,#27197,#27198,#27199,#27200,#27201,#27202,#27203,#27204,#27205,
#27206,#27207,#27208),.UNSPECIFIED.,.F.,.F.,(6,1,1,1,1,1,1,1,1,1,1,1,1,
1,1,1,1,1,1,1,1,1,1,1,1,1,1,1,1,1,1,1,1,1,1,1,1,1,1,1,1,1,1,1,1,1,1,1,1,
1,1,1,1,1,1,1,1,1,1,1,1,1,1,1,1,1,1,1,1,6),(0.,0.0142857142857143,0.0285714285714286,
0.0428571428571429,0.0571428571428571,0.0714285714285714,0.0857142857142857,
0.1,0.114285714285714,0.128571428571429,0.142857142857143,0.157142857142857,
0.171428571428571,0.185714285714286,0.2,0.214285714285714,0.228571428571429,
0.242857142857143,0.257142857142857,0.271428571428571,0.285714285714286,
0.3,0.314285714285714,0.328571428571429,0.342857142857143,0.357142857142857,
0.371428571428571,0.385714285714286,0.4,0.414285714285714,0.428571428571429,
0.442857142857143,0.457142857142857,0.471428571428572,0.485714285714286,
0.5,0.514285714285714,0.528571428571429,0.542857142857143,0.557142857142857,
0.571428571428571,0.585714285714286,0.6,0.614285714285714,0.628571428571428,
0.642857142857142,0.657142857142857,0.671428571428571,0.685714285714285,
0.699999999999999,0.714285714285714,0.728571428571428,0.742857142857142,
0.757142857142856,0.771428571428571,0.785714285714285,0.799999999999999,
0.814285714285713,0.828571428571428,0.842857142857142,0.857142857142856,
0.87142857142857,0.885714285714284,0.899999999999999,0.914285714285713,
0.928571428571427,0.942857142857141,0.957142857142856,0.97142857142857,
1.),.UNSPECIFIED.);
#542=B_SPLINE_CURVE_WITH_KNOTS('',5,(#27209,#27210,#27211,#27212,#27213,
#27214,#27215,#27216,#27217,#27218,#27219,#27220,#27221,#27222,#27223,#27224,
#27225,#27226,#27227,#27228,#27229,#27230,#27231,#27232,#27233,#27234,#27235,
#27236,#27237,#27238,#27239,#27240,#27241,#27242,#27243,#27244,#27245,#27246,
#27247,#27248,#27249,#27250,#27251,#27252,#27253,#27254,#27255,#27256,#27257,
#27258,#27259,#27260,#27261,#27262,#27263,#27264,#27265,#27266,#27267,#27268,
#27269,#27270,#27271,#27272,#27273,#27274,#27275,#27276,#27277,#27278,#27279,
#27280,#27281,#27282),.UNSPECIFIED.,.F.,.F.,(6,1,1,1,1,1,1,1,1,1,1,1,1,
1,1,1,1,1,1,1,1,1,1,1,1,1,1,1,1,1,1,1,1,1,1,1,1,1,1,1,1,1,1,1,1,1,1,1,1,
1,1,1,1,1,1,1,1,1,1,1,1,1,1,1,1,1,1,1,1,6),(0.,0.0142857142857143,0.0285714285714286,
0.0428571428571429,0.0571428571428571,0.0714285714285714,0.0857142857142857,
0.1,0.114285714285714,0.128571428571429,0.142857142857143,0.157142857142857,
0.171428571428571,0.185714285714286,0.2,0.214285714285714,0.228571428571429,
0.242857142857143,0.257142857142857,0.271428571428571,0.285714285714286,
0.3,0.314285714285714,0.328571428571429,0.342857142857143,0.357142857142857,
0.371428571428571,0.385714285714286,0.4,0.414285714285714,0.428571428571429,
0.442857142857143,0.457142857142857,0.471428571428572,0.485714285714286,
0.5,0.514285714285714,0.528571428571429,0.542857142857143,0.557142857142857,
0.571428571428571,0.585714285714286,0.6,0.614285714285714,0.628571428571428,
0.642857142857142,0.657142857142857,0.671428571428571,0.685714285714285,
0.699999999999999,0.714285714285714,0.728571428571428,0.742857142857142,
0.757142857142856,0.771428571428571,0.785714285714285,0.799999999999999,
0.814285714285713,0.828571428571428,0.842857142857142,0.857142857142856,
0.87142857142857,0.885714285714284,0.899999999999999,0.914285714285713,
0.928571428571427,0.942857142857141,0.957142857142856,0.97142857142857,
1.),.UNSPECIFIED.);
#543=B_SPLINE_CURVE_WITH_KNOTS('',5,(#27434,#27435,#27436,#27437,#27438,
#27439,#27440,#27441,#27442,#27443,#27444,#27445,#27446,#27447,#27448,#27449,
#27450,#27451,#27452,#27453,#27454,#27455,#27456,#27457,#27458,#27459,#27460,
#27461,#27462,#27463,#27464,#27465,#27466,#27467,#27468,#27469,#27470,#27471,
#27472,#27473,#27474,#27475,#27476,#27477,#27478,#27479,#27480,#27481,#27482,
#27483,#27484,#27485,#27486,#27487,#27488,#27489,#27490,#27491,#27492,#27493,
#27494,#27495,#27496,#27497,#27498,#27499,#27500,#27501,#27502,#27503,#27504,
#27505,#27506,#27507),.UNSPECIFIED.,.F.,.F.,(6,1,1,1,1,1,1,1,1,1,1,1,1,
1,1,1,1,1,1,1,1,1,1,1,1,1,1,1,1,1,1,1,1,1,1,1,1,1,1,1,1,1,1,1,1,1,1,1,1,
1,1,1,1,1,1,1,1,1,1,1,1,1,1,1,1,1,1,1,1,6),(0.,0.0142857142857143,0.0285714285714286,
0.0428571428571429,0.0571428571428571,0.0714285714285714,0.0857142857142857,
0.1,0.114285714285714,0.128571428571429,0.142857142857143,0.157142857142857,
0.171428571428571,0.185714285714286,0.2,0.214285714285714,0.228571428571429,
0.242857142857143,0.257142857142857,0.271428571428571,0.285714285714286,
0.3,0.314285714285714,0.328571428571429,0.342857142857143,0.357142857142857,
0.371428571428571,0.385714285714286,0.4,0.414285714285714,0.428571428571429,
0.442857142857143,0.457142857142857,0.471428571428572,0.485714285714286,
0.5,0.514285714285714,0.528571428571429,0.542857142857143,0.557142857142857,
0.571428571428571,0.585714285714286,0.6,0.614285714285714,0.628571428571428,
0.642857142857142,0.657142857142857,0.671428571428571,0.685714285714285,
0.699999999999999,0.714285714285714,0.728571428571428,0.742857142857142,
0.757142857142856,0.771428571428571,0.785714285714285,0.799999999999999,
0.814285714285713,0.828571428571428,0.842857142857142,0.857142857142856,
0.87142857142857,0.885714285714284,0.899999999999999,0.914285714285713,
0.928571428571427,0.942857142857141,0.957142857142856,0.97142857142857,
1.),.UNSPECIFIED.);
#544=B_SPLINE_CURVE_WITH_KNOTS('',5,(#27509,#27510,#27511,#27512,#27513,
#27514,#27515,#27516,#27517,#27518,#27519,#27520,#27521,#27522,#27523,#27524,
#27525,#27526,#27527,#27528,#27529,#27530,#27531,#27532,#27533,#27534,#27535,
#27536,#27537,#27538,#27539,#27540,#27541,#27542,#27543,#27544,#27545,#27546,
#27547,#27548,#27549,#27550,#27551,#27552,#27553,#27554,#27555,#27556,#27557,
#27558,#27559,#27560,#27561,#27562,#27563,#27564,#27565,#27566,#27567,#27568,
#27569,#27570,#27571,#27572,#27573,#27574,#27575,#27576,#27577,#27578,#27579,
#27580,#27581,#27582,#27583),.UNSPECIFIED.,.F.,.F.,(6,1,1,1,1,1,1,1,1,1,
1,1,1,1,1,1,1,1,1,1,1,1,1,1,1,1,1,1,1,1,1,1,1,1,1,1,1,1,1,1,1,1,1,1,1,1,
1,1,1,1,1,1,1,1,1,1,1,1,1,1,1,1,1,1,1,1,1,1,1,1,6),(-1.,-0.985714285714284,
-0.97142857142857,-0.957142857142856,-0.942857142857141,-0.928571428571427,
-0.914285714285713,-0.899999999999999,-0.885714285714284,-0.87142857142857,
-0.857142857142856,-0.842857142857142,-0.828571428571428,-0.814285714285713,
-0.799999999999999,-0.785714285714285,-0.771428571428571,-0.757142857142856,
-0.742857142857142,-0.728571428571428,-0.714285714285714,-0.699999999999999,
-0.685714285714285,-0.671428571428571,-0.657142857142857,-0.642857142857142,
-0.628571428571428,-0.614285714285714,-0.6,-0.585714285714286,-0.571428571428571,
-0.557142857142857,-0.542857142857143,-0.528571428571429,-0.514285714285714,
-0.5,-0.485714285714286,-0.471428571428572,-0.457142857142857,-0.442857142857143,
-0.428571428571429,-0.414285714285714,-0.4,-0.385714285714286,-0.371428571428571,
-0.357142857142857,-0.342857142857143,-0.328571428571429,-0.314285714285714,
-0.3,-0.285714285714286,-0.271428571428571,-0.257142857142857,-0.242857142857143,
-0.228571428571429,-0.214285714285714,-0.2,-0.185714285714286,-0.171428571428571,
-0.157142857142857,-0.142857142857143,-0.128571428571429,-0.114285714285714,
-0.1,-0.0857142857142857,-0.0714285714285714,-0.0571428571428571,-0.0428571428571429,
-0.0285714285714286,-0.0142857142857143,0.),.UNSPECIFIED.);
#545=B_SPLINE_CURVE_WITH_KNOTS('',5,(#27741,#27742,#27743,#27744,#27745,
#27746,#27747,#27748,#27749,#27750,#27751,#27752,#27753,#27754,#27755,#27756,
#27757,#27758,#27759,#27760,#27761,#27762,#27763,#27764,#27765,#27766,#27767,
#27768,#27769,#27770,#27771,#27772,#27773,#27774,#27775,#27776,#27777,#27778,
#27779,#27780,#27781,#27782,#27783,#27784,#27785,#27786,#27787,#27788,#27789,
#27790,#27791,#27792,#27793,#27794,#27795,#27796,#27797,#27798,#27799,#27800,
#27801,#27802,#27803,#27804,#27805,#27806,#27807,#27808,#27809,#27810,#27811,
#27812,#27813,#27814),.UNSPECIFIED.,.F.,.F.,(6,1,1,1,1,1,1,1,1,1,1,1,1,
1,1,1,1,1,1,1,1,1,1,1,1,1,1,1,1,1,1,1,1,1,1,1,1,1,1,1,1,1,1,1,1,1,1,1,1,
1,1,1,1,1,1,1,1,1,1,1,1,1,1,1,1,1,1,1,1,6),(0.,0.0142857142857143,0.0285714285714286,
0.0428571428571429,0.0571428571428571,0.0714285714285714,0.0857142857142857,
0.1,0.114285714285714,0.128571428571429,0.142857142857143,0.157142857142857,
0.171428571428571,0.185714285714286,0.2,0.214285714285714,0.228571428571429,
0.242857142857143,0.257142857142857,0.271428571428571,0.285714285714286,
0.3,0.314285714285714,0.328571428571429,0.342857142857143,0.357142857142857,
0.371428571428571,0.385714285714286,0.4,0.414285714285714,0.428571428571429,
0.442857142857143,0.457142857142857,0.471428571428572,0.485714285714286,
0.5,0.514285714285714,0.528571428571429,0.542857142857143,0.557142857142857,
0.571428571428571,0.585714285714286,0.6,0.614285714285714,0.628571428571428,
0.642857142857142,0.657142857142857,0.671428571428571,0.685714285714285,
0.699999999999999,0.714285714285714,0.728571428571428,0.742857142857142,
0.757142857142856,0.771428571428571,0.785714285714285,0.799999999999999,
0.814285714285713,0.828571428571428,0.842857142857142,0.857142857142856,
0.87142857142857,0.885714285714284,0.899999999999999,0.914285714285713,
0.928571428571427,0.942857142857141,0.957142857142856,0.97142857142857,
1.),.UNSPECIFIED.);
#546=B_SPLINE_CURVE_WITH_KNOTS('',5,(#27815,#27816,#27817,#27818,#27819,
#27820,#27821,#27822,#27823,#27824,#27825,#27826,#27827,#27828,#27829,#27830,
#27831,#27832,#27833,#27834,#27835,#27836,#27837,#27838,#27839,#27840,#27841,
#27842,#27843,#27844,#27845,#27846,#27847,#27848,#27849,#27850,#27851,#27852,
#27853,#27854,#27855,#27856,#27857,#27858,#27859,#27860,#27861,#27862,#27863,
#27864,#27865,#27866,#27867,#27868,#27869,#27870,#27871,#27872,#27873,#27874,
#27875,#27876,#27877,#27878,#27879,#27880,#27881,#27882,#27883,#27884,#27885,
#27886,#27887,#27888),.UNSPECIFIED.,.F.,.F.,(6,1,1,1,1,1,1,1,1,1,1,1,1,
1,1,1,1,1,1,1,1,1,1,1,1,1,1,1,1,1,1,1,1,1,1,1,1,1,1,1,1,1,1,1,1,1,1,1,1,
1,1,1,1,1,1,1,1,1,1,1,1,1,1,1,1,1,1,1,1,6),(0.,0.0142857142857143,0.0285714285714286,
0.0428571428571429,0.0571428571428571,0.0714285714285714,0.0857142857142857,
0.1,0.114285714285714,0.128571428571429,0.142857142857143,0.157142857142857,
0.171428571428571,0.185714285714286,0.2,0.214285714285714,0.228571428571429,
0.242857142857143,0.257142857142857,0.271428571428571,0.285714285714286,
0.3,0.314285714285714,0.328571428571429,0.342857142857143,0.357142857142857,
0.371428571428571,0.385714285714286,0.4,0.414285714285714,0.428571428571429,
0.442857142857143,0.457142857142857,0.471428571428572,0.485714285714286,
0.5,0.514285714285714,0.528571428571429,0.542857142857143,0.557142857142857,
0.571428571428571,0.585714285714286,0.6,0.614285714285714,0.628571428571428,
0.642857142857142,0.657142857142857,0.671428571428571,0.685714285714285,
0.699999999999999,0.714285714285714,0.728571428571428,0.742857142857142,
0.757142857142856,0.771428571428571,0.785714285714285,0.799999999999999,
0.814285714285713,0.828571428571428,0.842857142857142,0.857142857142856,
0.87142857142857,0.885714285714284,0.899999999999999,0.914285714285713,
0.928571428571427,0.942857142857141,0.957142857142856,0.97142857142857,
1.),.UNSPECIFIED.);
#547=B_SPLINE_CURVE_WITH_KNOTS('',5,(#28040,#28041,#28042,#28043,#28044,
#28045,#28046,#28047,#28048,#28049,#28050,#28051,#28052,#28053,#28054,#28055,
#28056,#28057,#28058,#28059,#28060,#28061,#28062,#28063,#28064,#28065,#28066,
#28067,#28068,#28069,#28070,#28071,#28072,#28073,#28074,#28075,#28076,#28077,
#28078,#28079,#28080,#28081,#28082,#28083,#28084,#28085,#28086,#28087,#28088,
#28089,#28090,#28091,#28092,#28093,#28094,#28095,#28096,#28097,#28098,#28099,
#28100,#28101,#28102,#28103,#28104,#28105,#28106,#28107,#28108,#28109,#28110,
#28111,#28112,#28113),.UNSPECIFIED.,.F.,.F.,(6,1,1,1,1,1,1,1,1,1,1,1,1,
1,1,1,1,1,1,1,1,1,1,1,1,1,1,1,1,1,1,1,1,1,1,1,1,1,1,1,1,1,1,1,1,1,1,1,1,
1,1,1,1,1,1,1,1,1,1,1,1,1,1,1,1,1,1,1,1,6),(0.,0.0142857142857143,0.0285714285714286,
0.0428571428571429,0.0571428571428571,0.0714285714285714,0.0857142857142857,
0.1,0.114285714285714,0.128571428571429,0.142857142857143,0.157142857142857,
0.171428571428571,0.185714285714286,0.2,0.214285714285714,0.228571428571429,
0.242857142857143,0.257142857142857,0.271428571428571,0.285714285714286,
0.3,0.314285714285714,0.328571428571429,0.342857142857143,0.357142857142857,
0.371428571428571,0.385714285714286,0.4,0.414285714285714,0.428571428571429,
0.442857142857143,0.457142857142857,0.471428571428572,0.485714285714286,
0.5,0.514285714285714,0.528571428571429,0.542857142857143,0.557142857142857,
0.571428571428571,0.585714285714286,0.6,0.614285714285714,0.628571428571428,
0.642857142857142,0.657142857142857,0.671428571428571,0.685714285714285,
0.699999999999999,0.714285714285714,0.728571428571428,0.742857142857142,
0.757142857142856,0.771428571428571,0.785714285714285,0.799999999999999,
0.814285714285713,0.828571428571428,0.842857142857142,0.857142857142856,
0.87142857142857,0.885714285714284,0.899999999999999,0.914285714285713,
0.928571428571427,0.942857142857141,0.957142857142856,0.97142857142857,
1.),.UNSPECIFIED.);
#548=B_SPLINE_CURVE_WITH_KNOTS('',5,(#28115,#28116,#28117,#28118,#28119,
#28120,#28121,#28122,#28123,#28124,#28125,#28126,#28127,#28128,#28129,#28130,
#28131,#28132,#28133,#28134,#28135,#28136,#28137,#28138,#28139,#28140,#28141,
#28142,#28143,#28144,#28145,#28146,#28147,#28148,#28149,#28150,#28151,#28152,
#28153,#28154,#28155,#28156,#28157,#28158,#28159,#28160,#28161,#28162,#28163,
#28164,#28165,#28166,#28167,#28168,#28169,#28170,#28171,#28172,#28173,#28174,
#28175,#28176,#28177,#28178,#28179,#28180,#28181,#28182,#28183,#28184,#28185,
#28186,#28187,#28188,#28189),.UNSPECIFIED.,.F.,.F.,(6,1,1,1,1,1,1,1,1,1,
1,1,1,1,1,1,1,1,1,1,1,1,1,1,1,1,1,1,1,1,1,1,1,1,1,1,1,1,1,1,1,1,1,1,1,1,
1,1,1,1,1,1,1,1,1,1,1,1,1,1,1,1,1,1,1,1,1,1,1,1,6),(-1.,-0.985714285714284,
-0.97142857142857,-0.957142857142856,-0.942857142857141,-0.928571428571427,
-0.914285714285713,-0.899999999999999,-0.885714285714284,-0.87142857142857,
-0.857142857142856,-0.842857142857142,-0.828571428571428,-0.814285714285713,
-0.799999999999999,-0.785714285714285,-0.771428571428571,-0.757142857142856,
-0.742857142857142,-0.728571428571428,-0.714285714285714,-0.699999999999999,
-0.685714285714285,-0.671428571428571,-0.657142857142857,-0.642857142857142,
-0.628571428571428,-0.614285714285714,-0.6,-0.585714285714286,-0.571428571428571,
-0.557142857142857,-0.542857142857143,-0.528571428571429,-0.514285714285714,
-0.5,-0.485714285714286,-0.471428571428572,-0.457142857142857,-0.442857142857143,
-0.428571428571429,-0.414285714285714,-0.4,-0.385714285714286,-0.371428571428571,
-0.357142857142857,-0.342857142857143,-0.328571428571429,-0.314285714285714,
-0.3,-0.285714285714286,-0.271428571428571,-0.257142857142857,-0.242857142857143,
-0.228571428571429,-0.214285714285714,-0.2,-0.185714285714286,-0.171428571428571,
-0.157142857142857,-0.142857142857143,-0.128571428571429,-0.114285714285714,
-0.1,-0.0857142857142857,-0.0714285714285714,-0.0571428571428571,-0.0428571428571429,
-0.0285714285714286,-0.0142857142857143,0.),.UNSPECIFIED.);
#549=B_SPLINE_CURVE_WITH_KNOTS('',5,(#28347,#28348,#28349,#28350,#28351,
#28352,#28353,#28354,#28355,#28356,#28357,#28358,#28359,#28360,#28361,#28362,
#28363,#28364,#28365,#28366,#28367,#28368,#28369,#28370,#28371,#28372,#28373,
#28374,#28375,#28376,#28377,#28378,#28379,#28380,#28381,#28382,#28383,#28384,
#28385,#28386,#28387,#28388,#28389,#28390,#28391,#28392,#28393,#28394,#28395,
#28396,#28397,#28398,#28399,#28400,#28401,#28402,#28403,#28404,#28405,#28406,
#28407,#28408,#28409,#28410,#28411,#28412,#28413,#28414,#28415,#28416,#28417,
#28418,#28419,#28420),.UNSPECIFIED.,.F.,.F.,(6,1,1,1,1,1,1,1,1,1,1,1,1,
1,1,1,1,1,1,1,1,1,1,1,1,1,1,1,1,1,1,1,1,1,1,1,1,1,1,1,1,1,1,1,1,1,1,1,1,
1,1,1,1,1,1,1,1,1,1,1,1,1,1,1,1,1,1,1,1,6),(0.,0.0142857142857143,0.0285714285714286,
0.0428571428571429,0.0571428571428571,0.0714285714285714,0.0857142857142857,
0.1,0.114285714285714,0.128571428571429,0.142857142857143,0.157142857142857,
0.171428571428571,0.185714285714286,0.2,0.214285714285714,0.228571428571429,
0.242857142857143,0.257142857142857,0.271428571428571,0.285714285714286,
0.3,0.314285714285714,0.328571428571429,0.342857142857143,0.357142857142857,
0.371428571428571,0.385714285714286,0.4,0.414285714285714,0.428571428571429,
0.442857142857143,0.457142857142857,0.471428571428572,0.485714285714286,
0.5,0.514285714285714,0.528571428571429,0.542857142857143,0.557142857142857,
0.571428571428571,0.585714285714286,0.6,0.614285714285714,0.628571428571428,
0.642857142857142,0.657142857142857,0.671428571428571,0.685714285714285,
0.699999999999999,0.714285714285714,0.728571428571428,0.742857142857142,
0.757142857142856,0.771428571428571,0.785714285714285,0.799999999999999,
0.814285714285713,0.828571428571428,0.842857142857142,0.857142857142856,
0.87142857142857,0.885714285714284,0.899999999999999,0.914285714285713,
0.928571428571427,0.942857142857141,0.957142857142856,0.97142857142857,
1.),.UNSPECIFIED.);
#550=B_SPLINE_CURVE_WITH_KNOTS('',5,(#28421,#28422,#28423,#28424,#28425,
#28426,#28427,#28428,#28429,#28430,#28431,#28432,#28433,#28434,#28435,#28436,
#28437,#28438,#28439,#28440,#28441,#28442,#28443,#28444,#28445,#28446,#28447,
#28448,#28449,#28450,#28451,#28452,#28453,#28454,#28455,#28456,#28457,#28458,
#28459,#28460,#28461,#28462,#28463,#28464,#28465,#28466,#28467,#28468,#28469,
#28470,#28471,#28472,#28473,#28474,#28475,#28476,#28477,#28478,#28479,#28480,
#28481,#28482,#28483,#28484,#28485,#28486,#28487,#28488,#28489,#28490,#28491,
#28492,#28493,#28494),.UNSPECIFIED.,.F.,.F.,(6,1,1,1,1,1,1,1,1,1,1,1,1,
1,1,1,1,1,1,1,1,1,1,1,1,1,1,1,1,1,1,1,1,1,1,1,1,1,1,1,1,1,1,1,1,1,1,1,1,
1,1,1,1,1,1,1,1,1,1,1,1,1,1,1,1,1,1,1,1,6),(0.,0.0142857142857143,0.0285714285714286,
0.0428571428571429,0.0571428571428571,0.0714285714285714,0.0857142857142857,
0.1,0.114285714285714,0.128571428571429,0.142857142857143,0.157142857142857,
0.171428571428571,0.185714285714286,0.2,0.214285714285714,0.228571428571429,
0.242857142857143,0.257142857142857,0.271428571428571,0.285714285714286,
0.3,0.314285714285714,0.328571428571429,0.342857142857143,0.357142857142857,
0.371428571428571,0.385714285714286,0.4,0.414285714285714,0.428571428571429,
0.442857142857143,0.457142857142857,0.471428571428572,0.485714285714286,
0.5,0.514285714285714,0.528571428571429,0.542857142857143,0.557142857142857,
0.571428571428571,0.585714285714286,0.6,0.614285714285714,0.628571428571428,
0.642857142857142,0.657142857142857,0.671428571428571,0.685714285714285,
0.699999999999999,0.714285714285714,0.728571428571428,0.742857142857142,
0.757142857142856,0.771428571428571,0.785714285714285,0.799999999999999,
0.814285714285713,0.828571428571428,0.842857142857142,0.857142857142856,
0.87142857142857,0.885714285714284,0.899999999999999,0.914285714285713,
0.928571428571427,0.942857142857141,0.957142857142856,0.97142857142857,
1.),.UNSPECIFIED.);
#551=B_SPLINE_CURVE_WITH_KNOTS('',5,(#28646,#28647,#28648,#28649,#28650,
#28651,#28652,#28653,#28654,#28655,#28656,#28657,#28658,#28659,#28660,#28661,
#28662,#28663,#28664,#28665,#28666,#28667,#28668,#28669,#28670,#28671,#28672,
#28673,#28674,#28675,#28676,#28677,#28678,#28679,#28680,#28681,#28682,#28683,
#28684,#28685,#28686,#28687,#28688,#28689,#28690,#28691,#28692,#28693,#28694,
#28695,#28696,#28697,#28698,#28699,#28700,#28701,#28702,#28703,#28704,#28705,
#28706,#28707,#28708,#28709,#28710,#28711,#28712,#28713,#28714,#28715,#28716,
#28717,#28718,#28719),.UNSPECIFIED.,.F.,.F.,(6,1,1,1,1,1,1,1,1,1,1,1,1,
1,1,1,1,1,1,1,1,1,1,1,1,1,1,1,1,1,1,1,1,1,1,1,1,1,1,1,1,1,1,1,1,1,1,1,1,
1,1,1,1,1,1,1,1,1,1,1,1,1,1,1,1,1,1,1,1,6),(0.,0.0142857142857143,0.0285714285714286,
0.0428571428571429,0.0571428571428571,0.0714285714285714,0.0857142857142857,
0.1,0.114285714285714,0.128571428571429,0.142857142857143,0.157142857142857,
0.171428571428571,0.185714285714286,0.2,0.214285714285714,0.228571428571429,
0.242857142857143,0.257142857142857,0.271428571428571,0.285714285714286,
0.3,0.314285714285714,0.328571428571429,0.342857142857143,0.357142857142857,
0.371428571428571,0.385714285714286,0.4,0.414285714285714,0.428571428571429,
0.442857142857143,0.457142857142857,0.471428571428572,0.485714285714286,
0.5,0.514285714285714,0.528571428571429,0.542857142857143,0.557142857142857,
0.571428571428571,0.585714285714286,0.6,0.614285714285714,0.628571428571428,
0.642857142857142,0.657142857142857,0.671428571428571,0.685714285714285,
0.699999999999999,0.714285714285714,0.728571428571428,0.742857142857142,
0.757142857142856,0.771428571428571,0.785714285714285,0.799999999999999,
0.814285714285713,0.828571428571428,0.842857142857142,0.857142857142856,
0.87142857142857,0.885714285714284,0.899999999999999,0.914285714285713,
0.928571428571427,0.942857142857141,0.957142857142856,0.97142857142857,
1.),.UNSPECIFIED.);
#552=B_SPLINE_CURVE_WITH_KNOTS('',5,(#28721,#28722,#28723,#28724,#28725,
#28726,#28727,#28728,#28729,#28730,#28731,#28732,#28733,#28734,#28735,#28736,
#28737,#28738,#28739,#28740,#28741,#28742,#28743,#28744,#28745,#28746,#28747,
#28748,#28749,#28750,#28751,#28752,#28753,#28754,#28755,#28756,#28757,#28758,
#28759,#28760,#28761,#28762,#28763,#28764,#28765,#28766,#28767,#28768,#28769,
#28770,#28771,#28772,#28773,#28774,#28775,#28776,#28777,#28778,#28779,#28780,
#28781,#28782,#28783,#28784,#28785,#28786,#28787,#28788,#28789,#28790,#28791,
#28792,#28793,#28794,#28795),.UNSPECIFIED.,.F.,.F.,(6,1,1,1,1,1,1,1,1,1,
1,1,1,1,1,1,1,1,1,1,1,1,1,1,1,1,1,1,1,1,1,1,1,1,1,1,1,1,1,1,1,1,1,1,1,1,
1,1,1,1,1,1,1,1,1,1,1,1,1,1,1,1,1,1,1,1,1,1,1,1,6),(-1.,-0.985714285714284,
-0.97142857142857,-0.957142857142856,-0.942857142857141,-0.928571428571427,
-0.914285714285713,-0.899999999999999,-0.885714285714284,-0.87142857142857,
-0.857142857142856,-0.842857142857142,-0.828571428571428,-0.814285714285713,
-0.799999999999999,-0.785714285714285,-0.771428571428571,-0.757142857142856,
-0.742857142857142,-0.728571428571428,-0.714285714285714,-0.699999999999999,
-0.685714285714285,-0.671428571428571,-0.657142857142857,-0.642857142857142,
-0.628571428571428,-0.614285714285714,-0.6,-0.585714285714286,-0.571428571428571,
-0.557142857142857,-0.542857142857143,-0.528571428571429,-0.514285714285714,
-0.5,-0.485714285714286,-0.471428571428572,-0.457142857142857,-0.442857142857143,
-0.428571428571429,-0.414285714285714,-0.4,-0.385714285714286,-0.371428571428571,
-0.357142857142857,-0.342857142857143,-0.328571428571429,-0.314285714285714,
-0.3,-0.285714285714286,-0.271428571428571,-0.257142857142857,-0.242857142857143,
-0.228571428571429,-0.214285714285714,-0.2,-0.185714285714286,-0.171428571428571,
-0.157142857142857,-0.142857142857143,-0.128571428571429,-0.114285714285714,
-0.1,-0.0857142857142857,-0.0714285714285714,-0.0571428571428571,-0.0428571428571429,
-0.0285714285714286,-0.0142857142857143,0.),.UNSPECIFIED.);
#553=B_SPLINE_CURVE_WITH_KNOTS('',5,(#28953,#28954,#28955,#28956,#28957,
#28958,#28959,#28960,#28961,#28962,#28963,#28964,#28965,#28966,#28967,#28968,
#28969,#28970,#28971,#28972,#28973,#28974,#28975,#28976,#28977,#28978,#28979,
#28980,#28981,#28982,#28983,#28984,#28985,#28986,#28987,#28988,#28989,#28990,
#28991,#28992,#28993,#28994,#28995,#28996,#28997,#28998,#28999,#29000,#29001,
#29002,#29003,#29004,#29005,#29006,#29007,#29008,#29009,#29010,#29011,#29012,
#29013,#29014,#29015,#29016,#29017,#29018,#29019,#29020,#29021,#29022,#29023,
#29024,#29025,#29026),.UNSPECIFIED.,.F.,.F.,(6,1,1,1,1,1,1,1,1,1,1,1,1,
1,1,1,1,1,1,1,1,1,1,1,1,1,1,1,1,1,1,1,1,1,1,1,1,1,1,1,1,1,1,1,1,1,1,1,1,
1,1,1,1,1,1,1,1,1,1,1,1,1,1,1,1,1,1,1,1,6),(0.,0.0142857142857143,0.0285714285714286,
0.0428571428571429,0.0571428571428571,0.0714285714285714,0.0857142857142857,
0.1,0.114285714285714,0.128571428571429,0.142857142857143,0.157142857142857,
0.171428571428571,0.185714285714286,0.2,0.214285714285714,0.228571428571429,
0.242857142857143,0.257142857142857,0.271428571428571,0.285714285714286,
0.3,0.314285714285714,0.328571428571429,0.342857142857143,0.357142857142857,
0.371428571428571,0.385714285714286,0.4,0.414285714285714,0.428571428571429,
0.442857142857143,0.457142857142857,0.471428571428572,0.485714285714286,
0.5,0.514285714285714,0.528571428571429,0.542857142857143,0.557142857142857,
0.571428571428571,0.585714285714286,0.6,0.614285714285714,0.628571428571428,
0.642857142857142,0.657142857142857,0.671428571428571,0.685714285714285,
0.699999999999999,0.714285714285714,0.728571428571428,0.742857142857142,
0.757142857142856,0.771428571428571,0.785714285714285,0.799999999999999,
0.814285714285713,0.828571428571428,0.842857142857142,0.857142857142856,
0.87142857142857,0.885714285714284,0.899999999999999,0.914285714285713,
0.928571428571427,0.942857142857141,0.957142857142856,0.97142857142857,
1.),.UNSPECIFIED.);
#554=B_SPLINE_CURVE_WITH_KNOTS('',5,(#29027,#29028,#29029,#29030,#29031,
#29032,#29033,#29034,#29035,#29036,#29037,#29038,#29039,#29040,#29041,#29042,
#29043,#29044,#29045,#29046,#29047,#29048,#29049,#29050,#29051,#29052,#29053,
#29054,#29055,#29056,#29057,#29058,#29059,#29060,#29061,#29062,#29063,#29064,
#29065,#29066,#29067,#29068,#29069,#29070,#29071,#29072,#29073,#29074,#29075,
#29076,#29077,#29078,#29079,#29080,#29081,#29082,#29083,#29084,#29085,#29086,
#29087,#29088,#29089,#29090,#29091,#29092,#29093,#29094,#29095,#29096,#29097,
#29098,#29099,#29100),.UNSPECIFIED.,.F.,.F.,(6,1,1,1,1,1,1,1,1,1,1,1,1,
1,1,1,1,1,1,1,1,1,1,1,1,1,1,1,1,1,1,1,1,1,1,1,1,1,1,1,1,1,1,1,1,1,1,1,1,
1,1,1,1,1,1,1,1,1,1,1,1,1,1,1,1,1,1,1,1,6),(0.,0.0142857142857143,0.0285714285714286,
0.0428571428571429,0.0571428571428571,0.0714285714285714,0.0857142857142857,
0.1,0.114285714285714,0.128571428571429,0.142857142857143,0.157142857142857,
0.171428571428571,0.185714285714286,0.2,0.214285714285714,0.228571428571429,
0.242857142857143,0.257142857142857,0.271428571428571,0.285714285714286,
0.3,0.314285714285714,0.328571428571429,0.342857142857143,0.357142857142857,
0.371428571428571,0.385714285714286,0.4,0.414285714285714,0.428571428571429,
0.442857142857143,0.457142857142857,0.471428571428572,0.485714285714286,
0.5,0.514285714285714,0.528571428571429,0.542857142857143,0.557142857142857,
0.571428571428571,0.585714285714286,0.6,0.614285714285714,0.628571428571428,
0.642857142857142,0.657142857142857,0.671428571428571,0.685714285714285,
0.699999999999999,0.714285714285714,0.728571428571428,0.742857142857142,
0.757142857142856,0.771428571428571,0.785714285714285,0.799999999999999,
0.814285714285713,0.828571428571428,0.842857142857142,0.857142857142856,
0.87142857142857,0.885714285714284,0.899999999999999,0.914285714285713,
0.928571428571427,0.942857142857141,0.957142857142856,0.97142857142857,
1.),.UNSPECIFIED.);
#555=B_SPLINE_CURVE_WITH_KNOTS('',5,(#29252,#29253,#29254,#29255,#29256,
#29257,#29258,#29259,#29260,#29261,#29262,#29263,#29264,#29265,#29266,#29267,
#29268,#29269,#29270,#29271,#29272,#29273,#29274,#29275,#29276,#29277,#29278,
#29279,#29280,#29281,#29282,#29283,#29284,#29285,#29286,#29287,#29288,#29289,
#29290,#29291,#29292,#29293,#29294,#29295,#29296,#29297,#29298,#29299,#29300,
#29301,#29302,#29303,#29304,#29305,#29306,#29307,#29308,#29309,#29310,#29311,
#29312,#29313,#29314,#29315,#29316,#29317,#29318,#29319,#29320,#29321,#29322,
#29323,#29324,#29325),.UNSPECIFIED.,.F.,.F.,(6,1,1,1,1,1,1,1,1,1,1,1,1,
1,1,1,1,1,1,1,1,1,1,1,1,1,1,1,1,1,1,1,1,1,1,1,1,1,1,1,1,1,1,1,1,1,1,1,1,
1,1,1,1,1,1,1,1,1,1,1,1,1,1,1,1,1,1,1,1,6),(0.,0.0142857142857143,0.0285714285714286,
0.0428571428571429,0.0571428571428571,0.0714285714285714,0.0857142857142857,
0.1,0.114285714285714,0.128571428571429,0.142857142857143,0.157142857142857,
0.171428571428571,0.185714285714286,0.2,0.214285714285714,0.228571428571429,
0.242857142857143,0.257142857142857,0.271428571428571,0.285714285714286,
0.3,0.314285714285714,0.328571428571429,0.342857142857143,0.357142857142857,
0.371428571428571,0.385714285714286,0.4,0.414285714285714,0.428571428571429,
0.442857142857143,0.457142857142857,0.471428571428572,0.485714285714286,
0.5,0.514285714285714,0.528571428571429,0.542857142857143,0.557142857142857,
0.571428571428571,0.585714285714286,0.6,0.614285714285714,0.628571428571428,
0.642857142857142,0.657142857142857,0.671428571428571,0.685714285714285,
0.699999999999999,0.714285714285714,0.728571428571428,0.742857142857142,
0.757142857142856,0.771428571428571,0.785714285714285,0.799999999999999,
0.814285714285713,0.828571428571428,0.842857142857142,0.857142857142856,
0.87142857142857,0.885714285714284,0.899999999999999,0.914285714285713,
0.928571428571427,0.942857142857141,0.957142857142856,0.97142857142857,
1.),.UNSPECIFIED.);
#556=B_SPLINE_CURVE_WITH_KNOTS('',5,(#29327,#29328,#29329,#29330,#29331,
#29332,#29333,#29334,#29335,#29336,#29337,#29338,#29339,#29340,#29341,#29342,
#29343,#29344,#29345,#29346,#29347,#29348,#29349,#29350,#29351,#29352,#29353,
#29354,#29355,#29356,#29357,#29358,#29359,#29360,#29361,#29362,#29363,#29364,
#29365,#29366,#29367,#29368,#29369,#29370,#29371,#29372,#29373,#29374,#29375,
#29376,#29377,#29378,#29379,#29380,#29381,#29382,#29383,#29384,#29385,#29386,
#29387,#29388,#29389,#29390,#29391,#29392,#29393,#29394,#29395,#29396,#29397,
#29398,#29399,#29400,#29401),.UNSPECIFIED.,.F.,.F.,(6,1,1,1,1,1,1,1,1,1,
1,1,1,1,1,1,1,1,1,1,1,1,1,1,1,1,1,1,1,1,1,1,1,1,1,1,1,1,1,1,1,1,1,1,1,1,
1,1,1,1,1,1,1,1,1,1,1,1,1,1,1,1,1,1,1,1,1,1,1,1,6),(-1.,-0.985714285714284,
-0.97142857142857,-0.957142857142856,-0.942857142857141,-0.928571428571427,
-0.914285714285713,-0.899999999999999,-0.885714285714284,-0.87142857142857,
-0.857142857142856,-0.842857142857142,-0.828571428571428,-0.814285714285713,
-0.799999999999999,-0.785714285714285,-0.771428571428571,-0.757142857142856,
-0.742857142857142,-0.728571428571428,-0.714285714285714,-0.699999999999999,
-0.685714285714285,-0.671428571428571,-0.657142857142857,-0.642857142857142,
-0.628571428571428,-0.614285714285714,-0.6,-0.585714285714286,-0.571428571428571,
-0.557142857142857,-0.542857142857143,-0.528571428571429,-0.514285714285714,
-0.5,-0.485714285714286,-0.471428571428572,-0.457142857142857,-0.442857142857143,
-0.428571428571429,-0.414285714285714,-0.4,-0.385714285714286,-0.371428571428571,
-0.357142857142857,-0.342857142857143,-0.328571428571429,-0.314285714285714,
-0.3,-0.285714285714286,-0.271428571428571,-0.257142857142857,-0.242857142857143,
-0.228571428571429,-0.214285714285714,-0.2,-0.185714285714286,-0.171428571428571,
-0.157142857142857,-0.142857142857143,-0.128571428571429,-0.114285714285714,
-0.1,-0.0857142857142857,-0.0714285714285714,-0.0571428571428571,-0.0428571428571429,
-0.0285714285714286,-0.0142857142857143,0.),.UNSPECIFIED.);
#557=B_SPLINE_CURVE_WITH_KNOTS('',5,(#29559,#29560,#29561,#29562,#29563,
#29564,#29565,#29566,#29567,#29568,#29569,#29570,#29571,#29572,#29573,#29574,
#29575,#29576,#29577,#29578,#29579,#29580,#29581,#29582,#29583,#29584,#29585,
#29586,#29587,#29588,#29589,#29590,#29591,#29592,#29593,#29594,#29595,#29596,
#29597,#29598,#29599,#29600,#29601,#29602,#29603,#29604,#29605,#29606,#29607,
#29608,#29609,#29610,#29611,#29612,#29613,#29614,#29615,#29616,#29617,#29618,
#29619,#29620,#29621,#29622,#29623,#29624,#29625,#29626,#29627,#29628,#29629,
#29630,#29631,#29632),.UNSPECIFIED.,.F.,.F.,(6,1,1,1,1,1,1,1,1,1,1,1,1,
1,1,1,1,1,1,1,1,1,1,1,1,1,1,1,1,1,1,1,1,1,1,1,1,1,1,1,1,1,1,1,1,1,1,1,1,
1,1,1,1,1,1,1,1,1,1,1,1,1,1,1,1,1,1,1,1,6),(0.,0.0142857142857143,0.0285714285714286,
0.0428571428571429,0.0571428571428571,0.0714285714285714,0.0857142857142857,
0.1,0.114285714285714,0.128571428571429,0.142857142857143,0.157142857142857,
0.171428571428571,0.185714285714286,0.2,0.214285714285714,0.228571428571429,
0.242857142857143,0.257142857142857,0.271428571428571,0.285714285714286,
0.3,0.314285714285714,0.328571428571429,0.342857142857143,0.357142857142857,
0.371428571428571,0.385714285714286,0.4,0.414285714285714,0.428571428571429,
0.442857142857143,0.457142857142857,0.471428571428572,0.485714285714286,
0.5,0.514285714285714,0.528571428571429,0.542857142857143,0.557142857142857,
0.571428571428571,0.585714285714286,0.6,0.614285714285714,0.628571428571428,
0.642857142857142,0.657142857142857,0.671428571428571,0.685714285714285,
0.699999999999999,0.714285714285714,0.728571428571428,0.742857142857142,
0.757142857142856,0.771428571428571,0.785714285714285,0.799999999999999,
0.814285714285713,0.828571428571428,0.842857142857142,0.857142857142856,
0.87142857142857,0.885714285714284,0.899999999999999,0.914285714285713,
0.928571428571427,0.942857142857141,0.957142857142856,0.97142857142857,
1.),.UNSPECIFIED.);
#558=B_SPLINE_CURVE_WITH_KNOTS('',5,(#29633,#29634,#29635,#29636,#29637,
#29638,#29639,#29640,#29641,#29642,#29643,#29644,#29645,#29646,#29647,#29648,
#29649,#29650,#29651,#29652,#29653,#29654,#29655,#29656,#29657,#29658,#29659,
#29660,#29661,#29662,#29663,#29664,#29665,#29666,#29667,#29668,#29669,#29670,
#29671,#29672,#29673,#29674,#29675,#29676,#29677,#29678,#29679,#29680,#29681,
#29682,#29683,#29684,#29685,#29686,#29687,#29688,#29689,#29690,#29691,#29692,
#29693,#29694,#29695,#29696,#29697,#29698,#29699,#29700,#29701,#29702,#29703,
#29704,#29705,#29706),.UNSPECIFIED.,.F.,.F.,(6,1,1,1,1,1,1,1,1,1,1,1,1,
1,1,1,1,1,1,1,1,1,1,1,1,1,1,1,1,1,1,1,1,1,1,1,1,1,1,1,1,1,1,1,1,1,1,1,1,
1,1,1,1,1,1,1,1,1,1,1,1,1,1,1,1,1,1,1,1,6),(0.,0.0142857142857143,0.0285714285714286,
0.0428571428571429,0.0571428571428571,0.0714285714285714,0.0857142857142857,
0.1,0.114285714285714,0.128571428571429,0.142857142857143,0.157142857142857,
0.171428571428571,0.185714285714286,0.2,0.214285714285714,0.228571428571429,
0.242857142857143,0.257142857142857,0.271428571428571,0.285714285714286,
0.3,0.314285714285714,0.328571428571429,0.342857142857143,0.357142857142857,
0.371428571428571,0.385714285714286,0.4,0.414285714285714,0.428571428571429,
0.442857142857143,0.457142857142857,0.471428571428572,0.485714285714286,
0.5,0.514285714285714,0.528571428571429,0.542857142857143,0.557142857142857,
0.571428571428571,0.585714285714286,0.6,0.614285714285714,0.628571428571428,
0.642857142857142,0.657142857142857,0.671428571428571,0.685714285714285,
0.699999999999999,0.714285714285714,0.728571428571428,0.742857142857142,
0.757142857142856,0.771428571428571,0.785714285714285,0.799999999999999,
0.814285714285713,0.828571428571428,0.842857142857142,0.857142857142856,
0.87142857142857,0.885714285714284,0.899999999999999,0.914285714285713,
0.928571428571427,0.942857142857141,0.957142857142856,0.97142857142857,
1.),.UNSPECIFIED.);
#559=B_SPLINE_CURVE_WITH_KNOTS('',5,(#29858,#29859,#29860,#29861,#29862,
#29863,#29864,#29865,#29866,#29867,#29868,#29869,#29870,#29871,#29872,#29873,
#29874,#29875,#29876,#29877,#29878,#29879,#29880,#29881,#29882,#29883,#29884,
#29885,#29886,#29887,#29888,#29889,#29890,#29891,#29892,#29893,#29894,#29895,
#29896,#29897,#29898,#29899,#29900,#29901,#29902,#29903,#29904,#29905,#29906,
#29907,#29908,#29909,#29910,#29911,#29912,#29913,#29914,#29915,#29916,#29917,
#29918,#29919,#29920,#29921,#29922,#29923,#29924,#29925,#29926,#29927,#29928,
#29929,#29930,#29931),.UNSPECIFIED.,.F.,.F.,(6,1,1,1,1,1,1,1,1,1,1,1,1,
1,1,1,1,1,1,1,1,1,1,1,1,1,1,1,1,1,1,1,1,1,1,1,1,1,1,1,1,1,1,1,1,1,1,1,1,
1,1,1,1,1,1,1,1,1,1,1,1,1,1,1,1,1,1,1,1,6),(0.,0.0142857142857143,0.0285714285714286,
0.0428571428571429,0.0571428571428571,0.0714285714285714,0.0857142857142857,
0.1,0.114285714285714,0.128571428571429,0.142857142857143,0.157142857142857,
0.171428571428571,0.185714285714286,0.2,0.214285714285714,0.228571428571429,
0.242857142857143,0.257142857142857,0.271428571428571,0.285714285714286,
0.3,0.314285714285714,0.328571428571429,0.342857142857143,0.357142857142857,
0.371428571428571,0.385714285714286,0.4,0.414285714285714,0.428571428571429,
0.442857142857143,0.457142857142857,0.471428571428572,0.485714285714286,
0.5,0.514285714285714,0.528571428571429,0.542857142857143,0.557142857142857,
0.571428571428571,0.585714285714286,0.6,0.614285714285714,0.628571428571428,
0.642857142857142,0.657142857142857,0.671428571428571,0.685714285714285,
0.699999999999999,0.714285714285714,0.728571428571428,0.742857142857142,
0.757142857142856,0.771428571428571,0.785714285714285,0.799999999999999,
0.814285714285713,0.828571428571428,0.842857142857142,0.857142857142856,
0.87142857142857,0.885714285714284,0.899999999999999,0.914285714285713,
0.928571428571427,0.942857142857141,0.957142857142856,0.97142857142857,
1.),.UNSPECIFIED.);
#560=B_SPLINE_CURVE_WITH_KNOTS('',5,(#29933,#29934,#29935,#29936,#29937,
#29938,#29939,#29940,#29941,#29942,#29943,#29944,#29945,#29946,#29947,#29948,
#29949,#29950,#29951,#29952,#29953,#29954,#29955,#29956,#29957,#29958,#29959,
#29960,#29961,#29962,#29963,#29964,#29965,#29966,#29967,#29968,#29969,#29970,
#29971,#29972,#29973,#29974,#29975,#29976,#29977,#29978,#29979,#29980,#29981,
#29982,#29983,#29984,#29985,#29986,#29987,#29988,#29989,#29990,#29991,#29992,
#29993,#29994,#29995,#29996,#29997,#29998,#29999,#30000,#30001,#30002,#30003,
#30004,#30005,#30006,#30007),.UNSPECIFIED.,.F.,.F.,(6,1,1,1,1,1,1,1,1,1,
1,1,1,1,1,1,1,1,1,1,1,1,1,1,1,1,1,1,1,1,1,1,1,1,1,1,1,1,1,1,1,1,1,1,1,1,
1,1,1,1,1,1,1,1,1,1,1,1,1,1,1,1,1,1,1,1,1,1,1,1,6),(-1.,-0.985714285714284,
-0.97142857142857,-0.957142857142856,-0.942857142857141,-0.928571428571427,
-0.914285714285713,-0.899999999999999,-0.885714285714284,-0.87142857142857,
-0.857142857142856,-0.842857142857142,-0.828571428571428,-0.814285714285713,
-0.799999999999999,-0.785714285714285,-0.771428571428571,-0.757142857142856,
-0.742857142857142,-0.728571428571428,-0.714285714285714,-0.699999999999999,
-0.685714285714285,-0.671428571428571,-0.657142857142857,-0.642857142857142,
-0.628571428571428,-0.614285714285714,-0.6,-0.585714285714286,-0.571428571428571,
-0.557142857142857,-0.542857142857143,-0.528571428571429,-0.514285714285714,
-0.5,-0.485714285714286,-0.471428571428572,-0.457142857142857,-0.442857142857143,
-0.428571428571429,-0.414285714285714,-0.4,-0.385714285714286,-0.371428571428571,
-0.357142857142857,-0.342857142857143,-0.328571428571429,-0.314285714285714,
-0.3,-0.285714285714286,-0.271428571428571,-0.257142857142857,-0.242857142857143,
-0.228571428571429,-0.214285714285714,-0.2,-0.185714285714286,-0.171428571428571,
-0.157142857142857,-0.142857142857143,-0.128571428571429,-0.114285714285714,
-0.1,-0.0857142857142857,-0.0714285714285714,-0.0571428571428571,-0.0428571428571429,
-0.0285714285714286,-0.0142857142857143,0.),.UNSPECIFIED.);
#561=B_SPLINE_CURVE_WITH_KNOTS('',5,(#30165,#30166,#30167,#30168,#30169,
#30170,#30171,#30172,#30173,#30174,#30175,#30176,#30177,#30178,#30179,#30180,
#30181,#30182,#30183,#30184,#30185,#30186,#30187,#30188,#30189,#30190,#30191,
#30192,#30193,#30194,#30195,#30196,#30197,#30198,#30199,#30200,#30201,#30202,
#30203,#30204,#30205,#30206,#30207,#30208,#30209,#30210,#30211,#30212,#30213,
#30214,#30215,#30216,#30217,#30218,#30219,#30220,#30221,#30222,#30223,#30224,
#30225,#30226,#30227,#30228,#30229,#30230,#30231,#30232,#30233,#30234,#30235,
#30236,#30237,#30238),.UNSPECIFIED.,.F.,.F.,(6,1,1,1,1,1,1,1,1,1,1,1,1,
1,1,1,1,1,1,1,1,1,1,1,1,1,1,1,1,1,1,1,1,1,1,1,1,1,1,1,1,1,1,1,1,1,1,1,1,
1,1,1,1,1,1,1,1,1,1,1,1,1,1,1,1,1,1,1,1,6),(0.,0.0142857142857143,0.0285714285714286,
0.0428571428571429,0.0571428571428571,0.0714285714285714,0.0857142857142857,
0.1,0.114285714285714,0.128571428571429,0.142857142857143,0.157142857142857,
0.171428571428571,0.185714285714286,0.2,0.214285714285714,0.228571428571429,
0.242857142857143,0.257142857142857,0.271428571428571,0.285714285714286,
0.3,0.314285714285714,0.328571428571429,0.342857142857143,0.357142857142857,
0.371428571428571,0.385714285714286,0.4,0.414285714285714,0.428571428571429,
0.442857142857143,0.457142857142857,0.471428571428572,0.485714285714286,
0.5,0.514285714285714,0.528571428571429,0.542857142857143,0.557142857142857,
0.571428571428571,0.585714285714286,0.6,0.614285714285714,0.628571428571428,
0.642857142857142,0.657142857142857,0.671428571428571,0.685714285714285,
0.699999999999999,0.714285714285714,0.728571428571428,0.742857142857142,
0.757142857142856,0.771428571428571,0.785714285714285,0.799999999999999,
0.814285714285713,0.828571428571428,0.842857142857142,0.857142857142856,
0.87142857142857,0.885714285714284,0.899999999999999,0.914285714285713,
0.928571428571427,0.942857142857141,0.957142857142856,0.97142857142857,
1.),.UNSPECIFIED.);
#562=B_SPLINE_CURVE_WITH_KNOTS('',5,(#30239,#30240,#30241,#30242,#30243,
#30244,#30245,#30246,#30247,#30248,#30249,#30250,#30251,#30252,#30253,#30254,
#30255,#30256,#30257,#30258,#30259,#30260,#30261,#30262,#30263,#30264,#30265,
#30266,#30267,#30268,#30269,#30270,#30271,#30272,#30273,#30274,#30275,#30276,
#30277,#30278,#30279,#30280,#30281,#30282,#30283,#30284,#30285,#30286,#30287,
#30288,#30289,#30290,#30291,#30292,#30293,#30294,#30295,#30296,#30297,#30298,
#30299,#30300,#30301,#30302,#30303,#30304,#30305,#30306,#30307,#30308,#30309,
#30310,#30311,#30312),.UNSPECIFIED.,.F.,.F.,(6,1,1,1,1,1,1,1,1,1,1,1,1,
1,1,1,1,1,1,1,1,1,1,1,1,1,1,1,1,1,1,1,1,1,1,1,1,1,1,1,1,1,1,1,1,1,1,1,1,
1,1,1,1,1,1,1,1,1,1,1,1,1,1,1,1,1,1,1,1,6),(0.,0.0142857142857143,0.0285714285714286,
0.0428571428571429,0.0571428571428571,0.0714285714285714,0.0857142857142857,
0.1,0.114285714285714,0.128571428571429,0.142857142857143,0.157142857142857,
0.171428571428571,0.185714285714286,0.2,0.214285714285714,0.228571428571429,
0.242857142857143,0.257142857142857,0.271428571428571,0.285714285714286,
0.3,0.314285714285714,0.328571428571429,0.342857142857143,0.357142857142857,
0.371428571428571,0.385714285714286,0.4,0.414285714285714,0.428571428571429,
0.442857142857143,0.457142857142857,0.471428571428572,0.485714285714286,
0.5,0.514285714285714,0.528571428571429,0.542857142857143,0.557142857142857,
0.571428571428571,0.585714285714286,0.6,0.614285714285714,0.628571428571428,
0.642857142857142,0.657142857142857,0.671428571428571,0.685714285714285,
0.699999999999999,0.714285714285714,0.728571428571428,0.742857142857142,
0.757142857142856,0.771428571428571,0.785714285714285,0.799999999999999,
0.814285714285713,0.828571428571428,0.842857142857142,0.857142857142856,
0.87142857142857,0.885714285714284,0.899999999999999,0.914285714285713,
0.928571428571427,0.942857142857141,0.957142857142856,0.97142857142857,
1.),.UNSPECIFIED.);
#563=B_SPLINE_CURVE_WITH_KNOTS('',5,(#30464,#30465,#30466,#30467,#30468,
#30469,#30470,#30471,#30472,#30473,#30474,#30475,#30476,#30477,#30478,#30479,
#30480,#30481,#30482,#30483,#30484,#30485,#30486,#30487,#30488,#30489,#30490,
#30491,#30492,#30493,#30494,#30495,#30496,#30497,#30498,#30499,#30500,#30501,
#30502,#30503,#30504,#30505,#30506,#30507,#30508,#30509,#30510,#30511,#30512,
#30513,#30514,#30515,#30516,#30517,#30518,#30519,#30520,#30521,#30522,#30523,
#30524,#30525,#30526,#30527,#30528,#30529,#30530,#30531,#30532,#30533,#30534,
#30535,#30536,#30537),.UNSPECIFIED.,.F.,.F.,(6,1,1,1,1,1,1,1,1,1,1,1,1,
1,1,1,1,1,1,1,1,1,1,1,1,1,1,1,1,1,1,1,1,1,1,1,1,1,1,1,1,1,1,1,1,1,1,1,1,
1,1,1,1,1,1,1,1,1,1,1,1,1,1,1,1,1,1,1,1,6),(0.,0.0142857142857143,0.0285714285714286,
0.0428571428571429,0.0571428571428571,0.0714285714285714,0.0857142857142857,
0.1,0.114285714285714,0.128571428571429,0.142857142857143,0.157142857142857,
0.171428571428571,0.185714285714286,0.2,0.214285714285714,0.228571428571429,
0.242857142857143,0.257142857142857,0.271428571428571,0.285714285714286,
0.3,0.314285714285714,0.328571428571429,0.342857142857143,0.357142857142857,
0.371428571428571,0.385714285714286,0.4,0.414285714285714,0.428571428571429,
0.442857142857143,0.457142857142857,0.471428571428572,0.485714285714286,
0.5,0.514285714285714,0.528571428571429,0.542857142857143,0.557142857142857,
0.571428571428571,0.585714285714286,0.6,0.614285714285714,0.628571428571428,
0.642857142857142,0.657142857142857,0.671428571428571,0.685714285714285,
0.699999999999999,0.714285714285714,0.728571428571428,0.742857142857142,
0.757142857142856,0.771428571428571,0.785714285714285,0.799999999999999,
0.814285714285713,0.828571428571428,0.842857142857142,0.857142857142856,
0.87142857142857,0.885714285714284,0.899999999999999,0.914285714285713,
0.928571428571427,0.942857142857141,0.957142857142856,0.97142857142857,
1.),.UNSPECIFIED.);
#564=B_SPLINE_CURVE_WITH_KNOTS('',5,(#30539,#30540,#30541,#30542,#30543,
#30544,#30545,#30546,#30547,#30548,#30549,#30550,#30551,#30552,#30553,#30554,
#30555,#30556,#30557,#30558,#30559,#30560,#30561,#30562,#30563,#30564,#30565,
#30566,#30567,#30568,#30569,#30570,#30571,#30572,#30573,#30574,#30575,#30576,
#30577,#30578,#30579,#30580,#30581,#30582,#30583,#30584,#30585,#30586,#30587,
#30588,#30589,#30590,#30591,#30592,#30593,#30594,#30595,#30596,#30597,#30598,
#30599,#30600,#30601,#30602,#30603,#30604,#30605,#30606,#30607,#30608,#30609,
#30610,#30611,#30612,#30613),.UNSPECIFIED.,.F.,.F.,(6,1,1,1,1,1,1,1,1,1,
1,1,1,1,1,1,1,1,1,1,1,1,1,1,1,1,1,1,1,1,1,1,1,1,1,1,1,1,1,1,1,1,1,1,1,1,
1,1,1,1,1,1,1,1,1,1,1,1,1,1,1,1,1,1,1,1,1,1,1,1,6),(-1.,-0.985714285714284,
-0.97142857142857,-0.957142857142856,-0.942857142857141,-0.928571428571427,
-0.914285714285713,-0.899999999999999,-0.885714285714284,-0.87142857142857,
-0.857142857142856,-0.842857142857142,-0.828571428571428,-0.814285714285713,
-0.799999999999999,-0.785714285714285,-0.771428571428571,-0.757142857142856,
-0.742857142857142,-0.728571428571428,-0.714285714285714,-0.699999999999999,
-0.685714285714285,-0.671428571428571,-0.657142857142857,-0.642857142857142,
-0.628571428571428,-0.614285714285714,-0.6,-0.585714285714286,-0.571428571428571,
-0.557142857142857,-0.542857142857143,-0.528571428571429,-0.514285714285714,
-0.5,-0.485714285714286,-0.471428571428572,-0.457142857142857,-0.442857142857143,
-0.428571428571429,-0.414285714285714,-0.4,-0.385714285714286,-0.371428571428571,
-0.357142857142857,-0.342857142857143,-0.328571428571429,-0.314285714285714,
-0.3,-0.285714285714286,-0.271428571428571,-0.257142857142857,-0.242857142857143,
-0.228571428571429,-0.214285714285714,-0.2,-0.185714285714286,-0.171428571428571,
-0.157142857142857,-0.142857142857143,-0.128571428571429,-0.114285714285714,
-0.1,-0.0857142857142857,-0.0714285714285714,-0.0571428571428571,-0.0428571428571429,
-0.0285714285714286,-0.0142857142857143,0.),.UNSPECIFIED.);
#565=B_SPLINE_CURVE_WITH_KNOTS('',5,(#30771,#30772,#30773,#30774,#30775,
#30776,#30777,#30778,#30779,#30780,#30781,#30782,#30783,#30784,#30785,#30786,
#30787,#30788,#30789,#30790,#30791,#30792,#30793,#30794,#30795,#30796,#30797,
#30798,#30799,#30800,#30801,#30802,#30803,#30804,#30805,#30806,#30807,#30808,
#30809,#30810,#30811,#30812,#30813,#30814,#30815,#30816,#30817,#30818,#30819,
#30820,#30821,#30822,#30823,#30824,#30825,#30826,#30827,#30828,#30829,#30830,
#30831,#30832,#30833,#30834,#30835,#30836,#30837,#30838,#30839,#30840,#30841,
#30842,#30843,#30844),.UNSPECIFIED.,.F.,.F.,(6,1,1,1,1,1,1,1,1,1,1,1,1,
1,1,1,1,1,1,1,1,1,1,1,1,1,1,1,1,1,1,1,1,1,1,1,1,1,1,1,1,1,1,1,1,1,1,1,1,
1,1,1,1,1,1,1,1,1,1,1,1,1,1,1,1,1,1,1,1,6),(0.,0.0142857142857143,0.0285714285714286,
0.0428571428571429,0.0571428571428571,0.0714285714285714,0.0857142857142857,
0.1,0.114285714285714,0.128571428571429,0.142857142857143,0.157142857142857,
0.171428571428571,0.185714285714286,0.2,0.214285714285714,0.228571428571429,
0.242857142857143,0.257142857142857,0.271428571428571,0.285714285714286,
0.3,0.314285714285714,0.328571428571429,0.342857142857143,0.357142857142857,
0.371428571428571,0.385714285714286,0.4,0.414285714285714,0.428571428571429,
0.442857142857143,0.457142857142857,0.471428571428572,0.485714285714286,
0.5,0.514285714285714,0.528571428571429,0.542857142857143,0.557142857142857,
0.571428571428571,0.585714285714286,0.6,0.614285714285714,0.628571428571428,
0.642857142857142,0.657142857142857,0.671428571428571,0.685714285714285,
0.699999999999999,0.714285714285714,0.728571428571428,0.742857142857142,
0.757142857142856,0.771428571428571,0.785714285714285,0.799999999999999,
0.814285714285713,0.828571428571428,0.842857142857142,0.857142857142856,
0.87142857142857,0.885714285714284,0.899999999999999,0.914285714285713,
0.928571428571427,0.942857142857141,0.957142857142856,0.97142857142857,
1.),.UNSPECIFIED.);
#566=B_SPLINE_CURVE_WITH_KNOTS('',5,(#30845,#30846,#30847,#30848,#30849,
#30850,#30851,#30852,#30853,#30854,#30855,#30856,#30857,#30858,#30859,#30860,
#30861,#30862,#30863,#30864,#30865,#30866,#30867,#30868,#30869,#30870,#30871,
#30872,#30873,#30874,#30875,#30876,#30877,#30878,#30879,#30880,#30881,#30882,
#30883,#30884,#30885,#30886,#30887,#30888,#30889,#30890,#30891,#30892,#30893,
#30894,#30895,#30896,#30897,#30898,#30899,#30900,#30901,#30902,#30903,#30904,
#30905,#30906,#30907,#30908,#30909,#30910,#30911,#30912,#30913,#30914,#30915,
#30916,#30917,#30918),.UNSPECIFIED.,.F.,.F.,(6,1,1,1,1,1,1,1,1,1,1,1,1,
1,1,1,1,1,1,1,1,1,1,1,1,1,1,1,1,1,1,1,1,1,1,1,1,1,1,1,1,1,1,1,1,1,1,1,1,
1,1,1,1,1,1,1,1,1,1,1,1,1,1,1,1,1,1,1,1,6),(0.,0.0142857142857143,0.0285714285714286,
0.0428571428571429,0.0571428571428571,0.0714285714285714,0.0857142857142857,
0.1,0.114285714285714,0.128571428571429,0.142857142857143,0.157142857142857,
0.171428571428571,0.185714285714286,0.2,0.214285714285714,0.228571428571429,
0.242857142857143,0.257142857142857,0.271428571428571,0.285714285714286,
0.3,0.314285714285714,0.328571428571429,0.342857142857143,0.357142857142857,
0.371428571428571,0.385714285714286,0.4,0.414285714285714,0.428571428571429,
0.442857142857143,0.457142857142857,0.471428571428572,0.485714285714286,
0.5,0.514285714285714,0.528571428571429,0.542857142857143,0.557142857142857,
0.571428571428571,0.585714285714286,0.6,0.614285714285714,0.628571428571428,
0.642857142857142,0.657142857142857,0.671428571428571,0.685714285714285,
0.699999999999999,0.714285714285714,0.728571428571428,0.742857142857142,
0.757142857142856,0.771428571428571,0.785714285714285,0.799999999999999,
0.814285714285713,0.828571428571428,0.842857142857142,0.857142857142856,
0.87142857142857,0.885714285714284,0.899999999999999,0.914285714285713,
0.928571428571427,0.942857142857141,0.957142857142856,0.97142857142857,
1.),.UNSPECIFIED.);
#567=B_SPLINE_CURVE_WITH_KNOTS('',5,(#30944,#30945,#30946,#30947,#30948,
#30949,#30950,#30951,#30952,#30953,#30954,#30955,#30956,#30957,#30958,#30959,
#30960,#30961,#30962,#30963,#30964,#30965,#30966,#30967,#30968,#30969,#30970,
#30971,#30972,#30973,#30974,#30975,#30976,#30977,#30978,#30979,#30980,#30981,
#30982,#30983,#30984,#30985,#30986,#30987,#30988,#30989,#30990,#30991,#30992,
#30993,#30994,#30995,#30996,#30997,#30998,#30999,#31000,#31001,#31002,#31003,
#31004,#31005,#31006,#31007,#31008,#31009,#31010,#31011,#31012,#31013,#31014,
#31015,#31016,#31017),.UNSPECIFIED.,.F.,.F.,(6,1,1,1,1,1,1,1,1,1,1,1,1,
1,1,1,1,1,1,1,1,1,1,1,1,1,1,1,1,1,1,1,1,1,1,1,1,1,1,1,1,1,1,1,1,1,1,1,1,
1,1,1,1,1,1,1,1,1,1,1,1,1,1,1,1,1,1,1,1,6),(0.,0.0142857142857143,0.0285714285714286,
0.0428571428571429,0.0571428571428571,0.0714285714285714,0.0857142857142857,
0.1,0.114285714285714,0.128571428571429,0.142857142857143,0.157142857142857,
0.171428571428571,0.185714285714286,0.2,0.214285714285714,0.228571428571429,
0.242857142857143,0.257142857142857,0.271428571428571,0.285714285714286,
0.3,0.314285714285714,0.328571428571429,0.342857142857143,0.357142857142857,
0.371428571428571,0.385714285714286,0.4,0.414285714285714,0.428571428571429,
0.442857142857143,0.457142857142857,0.471428571428572,0.485714285714286,
0.5,0.514285714285714,0.528571428571429,0.542857142857143,0.557142857142857,
0.571428571428571,0.585714285714286,0.6,0.614285714285714,0.628571428571428,
0.642857142857142,0.657142857142857,0.671428571428571,0.685714285714285,
0.699999999999999,0.714285714285714,0.728571428571428,0.742857142857142,
0.757142857142856,0.771428571428571,0.785714285714285,0.799999999999999,
0.814285714285713,0.828571428571428,0.842857142857142,0.857142857142856,
0.87142857142857,0.885714285714284,0.899999999999999,0.914285714285713,
0.928571428571427,0.942857142857141,0.957142857142856,0.97142857142857,
1.),.UNSPECIFIED.);
#568=B_SPLINE_CURVE_WITH_KNOTS('',5,(#31021,#31022,#31023,#31024,#31025,
#31026,#31027,#31028,#31029,#31030,#31031,#31032,#31033,#31034,#31035,#31036,
#31037,#31038,#31039,#31040,#31041,#31042,#31043,#31044,#31045,#31046,#31047,
#31048,#31049,#31050,#31051,#31052,#31053,#31054,#31055,#31056,#31057,#31058,
#31059,#31060,#31061,#31062,#31063,#31064,#31065,#31066,#31067,#31068,#31069,
#31070,#31071,#31072,#31073,#31074,#31075,#31076,#31077,#31078,#31079,#31080,
#31081,#31082,#31083,#31084,#31085,#31086,#31087,#31088,#31089,#31090,#31091,
#31092,#31093,#31094),.UNSPECIFIED.,.F.,.F.,(6,1,1,1,1,1,1,1,1,1,1,1,1,
1,1,1,1,1,1,1,1,1,1,1,1,1,1,1,1,1,1,1,1,1,1,1,1,1,1,1,1,1,1,1,1,1,1,1,1,
1,1,1,1,1,1,1,1,1,1,1,1,1,1,1,1,1,1,1,1,6),(0.,0.0142857142857143,0.0285714285714286,
0.0428571428571429,0.0571428571428571,0.0714285714285714,0.0857142857142857,
0.1,0.114285714285714,0.128571428571429,0.142857142857143,0.157142857142857,
0.171428571428571,0.185714285714286,0.2,0.214285714285714,0.228571428571429,
0.242857142857143,0.257142857142857,0.271428571428571,0.285714285714286,
0.3,0.314285714285714,0.328571428571429,0.342857142857143,0.357142857142857,
0.371428571428571,0.385714285714286,0.4,0.414285714285714,0.428571428571429,
0.442857142857143,0.457142857142857,0.471428571428572,0.485714285714286,
0.5,0.514285714285714,0.528571428571429,0.542857142857143,0.557142857142857,
0.571428571428571,0.585714285714286,0.6,0.614285714285714,0.628571428571428,
0.642857142857142,0.657142857142857,0.671428571428571,0.685714285714285,
0.699999999999999,0.714285714285714,0.728571428571428,0.742857142857142,
0.757142857142856,0.771428571428571,0.785714285714285,0.799999999999999,
0.814285714285713,0.828571428571428,0.842857142857142,0.857142857142856,
0.87142857142857,0.885714285714284,0.899999999999999,0.914285714285713,
0.928571428571427,0.942857142857141,0.957142857142856,0.97142857142857,
1.),.UNSPECIFIED.);
#569=B_SPLINE_CURVE_WITH_KNOTS('',5,(#31109,#31110,#31111,#31112,#31113,
#31114,#31115,#31116,#31117,#31118,#31119,#31120,#31121,#31122,#31123,#31124,
#31125,#31126,#31127,#31128,#31129,#31130,#31131,#31132,#31133,#31134,#31135,
#31136,#31137,#31138,#31139,#31140,#31141,#31142,#31143,#31144,#31145,#31146,
#31147,#31148,#31149,#31150,#31151,#31152,#31153,#31154,#31155,#31156,#31157,
#31158,#31159,#31160,#31161,#31162,#31163,#31164,#31165,#31166,#31167,#31168,
#31169,#31170,#31171,#31172,#31173,#31174,#31175,#31176,#31177,#31178,#31179,
#31180,#31181,#31182),.UNSPECIFIED.,.F.,.F.,(6,1,1,1,1,1,1,1,1,1,1,1,1,
1,1,1,1,1,1,1,1,1,1,1,1,1,1,1,1,1,1,1,1,1,1,1,1,1,1,1,1,1,1,1,1,1,1,1,1,
1,1,1,1,1,1,1,1,1,1,1,1,1,1,1,1,1,1,1,1,6),(0.,0.0142857142857143,0.0285714285714286,
0.0428571428571429,0.0571428571428571,0.0714285714285714,0.0857142857142857,
0.1,0.114285714285714,0.128571428571429,0.142857142857143,0.157142857142857,
0.171428571428571,0.185714285714286,0.2,0.214285714285714,0.228571428571429,
0.242857142857143,0.257142857142857,0.271428571428571,0.285714285714286,
0.3,0.314285714285714,0.328571428571429,0.342857142857143,0.357142857142857,
0.371428571428571,0.385714285714286,0.4,0.414285714285714,0.428571428571429,
0.442857142857143,0.457142857142857,0.471428571428572,0.485714285714286,
0.5,0.514285714285714,0.528571428571429,0.542857142857143,0.557142857142857,
0.571428571428571,0.585714285714286,0.6,0.614285714285714,0.628571428571428,
0.642857142857142,0.657142857142857,0.671428571428571,0.685714285714285,
0.699999999999999,0.714285714285714,0.728571428571428,0.742857142857142,
0.757142857142856,0.771428571428571,0.785714285714285,0.799999999999999,
0.814285714285713,0.828571428571428,0.842857142857142,0.857142857142856,
0.87142857142857,0.885714285714284,0.899999999999999,0.914285714285713,
0.928571428571427,0.942857142857141,0.957142857142856,0.97142857142857,
1.),.UNSPECIFIED.);
#570=B_SPLINE_CURVE_WITH_KNOTS('',5,(#31186,#31187,#31188,#31189,#31190,
#31191,#31192,#31193,#31194,#31195,#31196,#31197,#31198,#31199,#31200,#31201,
#31202,#31203,#31204,#31205,#31206,#31207,#31208,#31209,#31210,#31211,#31212,
#31213,#31214,#31215,#31216,#31217,#31218,#31219,#31220,#31221,#31222,#31223,
#31224,#31225,#31226,#31227,#31228,#31229,#31230,#31231,#31232,#31233,#31234,
#31235,#31236,#31237,#31238,#31239,#31240,#31241,#31242,#31243,#31244,#31245,
#31246,#31247,#31248,#31249,#31250,#31251,#31252,#31253,#31254,#31255,#31256,
#31257,#31258,#31259,#31260),.UNSPECIFIED.,.F.,.F.,(6,1,1,1,1,1,1,1,1,1,
1,1,1,1,1,1,1,1,1,1,1,1,1,1,1,1,1,1,1,1,1,1,1,1,1,1,1,1,1,1,1,1,1,1,1,1,
1,1,1,1,1,1,1,1,1,1,1,1,1,1,1,1,1,1,1,1,1,1,1,1,6),(-1.,-0.985714285714284,
-0.97142857142857,-0.957142857142856,-0.942857142857141,-0.928571428571427,
-0.914285714285713,-0.899999999999999,-0.885714285714284,-0.87142857142857,
-0.857142857142856,-0.842857142857142,-0.828571428571428,-0.814285714285713,
-0.799999999999999,-0.785714285714285,-0.771428571428571,-0.757142857142856,
-0.742857142857142,-0.728571428571428,-0.714285714285714,-0.699999999999999,
-0.685714285714285,-0.671428571428571,-0.657142857142857,-0.642857142857142,
-0.628571428571428,-0.614285714285714,-0.6,-0.585714285714286,-0.571428571428571,
-0.557142857142857,-0.542857142857143,-0.528571428571429,-0.514285714285714,
-0.5,-0.485714285714286,-0.471428571428572,-0.457142857142857,-0.442857142857143,
-0.428571428571429,-0.414285714285714,-0.4,-0.385714285714286,-0.371428571428571,
-0.357142857142857,-0.342857142857143,-0.328571428571429,-0.314285714285714,
-0.3,-0.285714285714286,-0.271428571428571,-0.257142857142857,-0.242857142857143,
-0.228571428571429,-0.214285714285714,-0.2,-0.185714285714286,-0.171428571428571,
-0.157142857142857,-0.142857142857143,-0.128571428571429,-0.114285714285714,
-0.1,-0.0857142857142857,-0.0714285714285714,-0.0571428571428571,-0.0428571428571429,
-0.0285714285714286,-0.0142857142857143,0.),.UNSPECIFIED.);
#947=B_SPLINE_SURFACE_WITH_KNOTS('',5,1,((#19405,#19406),(#19407,#19408),
(#19409,#19410),(#19411,#19412),(#19413,#19414),(#19415,#19416),(#19417,
#19418),(#19419,#19420),(#19421,#19422),(#19423,#19424),(#19425,#19426),
(#19427,#19428),(#19429,#19430),(#19431,#19432),(#19433,#19434),(#19435,
#19436),(#19437,#19438),(#19439,#19440),(#19441,#19442),(#19443,#19444),
(#19445,#19446),(#19447,#19448),(#19449,#19450),(#19451,#19452),(#19453,
#19454),(#19455,#19456),(#19457,#19458),(#19459,#19460),(#19461,#19462),
(#19463,#19464),(#19465,#19466),(#19467,#19468),(#19469,#19470),(#19471,
#19472),(#19473,#19474),(#19475,#19476),(#19477,#19478),(#19479,#19480),
(#19481,#19482),(#19483,#19484),(#19485,#19486),(#19487,#19488),(#19489,
#19490),(#19491,#19492),(#19493,#19494),(#19495,#19496),(#19497,#19498),
(#19499,#19500),(#19501,#19502),(#19503,#19504),(#19505,#19506),(#19507,
#19508),(#19509,#19510),(#19511,#19512),(#19513,#19514),(#19515,#19516),
(#19517,#19518),(#19519,#19520),(#19521,#19522),(#19523,#19524),(#19525,
#19526),(#19527,#19528),(#19529,#19530),(#19531,#19532),(#19533,#19534),
(#19535,#19536),(#19537,#19538),(#19539,#19540),(#19541,#19542),(#19543,
#19544),(#19545,#19546),(#19547,#19548),(#19549,#19550),(#19551,#19552),
(#19553,#19554)),.UNSPECIFIED.,.F.,.F.,.F.,(6,1,1,1,1,1,1,1,1,1,1,1,1,1,
1,1,1,1,1,1,1,1,1,1,1,1,1,1,1,1,1,1,1,1,1,1,1,1,1,1,1,1,1,1,1,1,1,1,1,1,
1,1,1,1,1,1,1,1,1,1,1,1,1,1,1,1,1,1,1,1,6),(2,2),(-1.,-0.985714285714284,
-0.97142857142857,-0.957142857142856,-0.942857142857141,-0.928571428571427,
-0.914285714285713,-0.899999999999999,-0.885714285714284,-0.87142857142857,
-0.857142857142856,-0.842857142857142,-0.828571428571428,-0.814285714285713,
-0.799999999999999,-0.785714285714285,-0.771428571428571,-0.757142857142856,
-0.742857142857142,-0.728571428571428,-0.714285714285714,-0.699999999999999,
-0.685714285714285,-0.671428571428571,-0.657142857142857,-0.642857142857142,
-0.628571428571428,-0.614285714285714,-0.6,-0.585714285714286,-0.571428571428571,
-0.557142857142857,-0.542857142857143,-0.528571428571429,-0.514285714285714,
-0.5,-0.485714285714286,-0.471428571428572,-0.457142857142857,-0.442857142857143,
-0.428571428571429,-0.414285714285714,-0.4,-0.385714285714286,-0.371428571428571,
-0.357142857142857,-0.342857142857143,-0.328571428571429,-0.314285714285714,
-0.3,-0.285714285714286,-0.271428571428571,-0.257142857142857,-0.242857142857143,
-0.228571428571429,-0.214285714285714,-0.2,-0.185714285714286,-0.171428571428571,
-0.157142857142857,-0.142857142857143,-0.128571428571429,-0.114285714285714,
-0.1,-0.0857142857142857,-0.0714285714285714,-0.0571428571428571,-0.0428571428571429,
-0.0285714285714286,-0.0142857142857143,0.),(0.,1.8),.UNSPECIFIED.);
#948=B_SPLINE_SURFACE_WITH_KNOTS('',5,1,((#19713,#19714),(#19715,#19716),
(#19717,#19718),(#19719,#19720),(#19721,#19722),(#19723,#19724),(#19725,
#19726),(#19727,#19728),(#19729,#19730),(#19731,#19732),(#19733,#19734),
(#19735,#19736),(#19737,#19738),(#19739,#19740),(#19741,#19742),(#19743,
#19744),(#19745,#19746),(#19747,#19748),(#19749,#19750),(#19751,#19752),
(#19753,#19754),(#19755,#19756),(#19757,#19758),(#19759,#19760),(#19761,
#19762),(#19763,#19764),(#19765,#19766),(#19767,#19768),(#19769,#19770),
(#19771,#19772),(#19773,#19774),(#19775,#19776),(#19777,#19778),(#19779,
#19780),(#19781,#19782),(#19783,#19784),(#19785,#19786),(#19787,#19788),
(#19789,#19790),(#19791,#19792),(#19793,#19794),(#19795,#19796),(#19797,
#19798),(#19799,#19800),(#19801,#19802),(#19803,#19804),(#19805,#19806),
(#19807,#19808),(#19809,#19810),(#19811,#19812),(#19813,#19814),(#19815,
#19816),(#19817,#19818),(#19819,#19820),(#19821,#19822),(#19823,#19824),
(#19825,#19826),(#19827,#19828),(#19829,#19830),(#19831,#19832),(#19833,
#19834),(#19835,#19836),(#19837,#19838),(#19839,#19840),(#19841,#19842),
(#19843,#19844),(#19845,#19846),(#19847,#19848),(#19849,#19850),(#19851,
#19852),(#19853,#19854),(#19855,#19856),(#19857,#19858),(#19859,#19860),
(#19861,#19862)),.UNSPECIFIED.,.F.,.F.,.F.,(6,1,1,1,1,1,1,1,1,1,1,1,1,1,
1,1,1,1,1,1,1,1,1,1,1,1,1,1,1,1,1,1,1,1,1,1,1,1,1,1,1,1,1,1,1,1,1,1,1,1,
1,1,1,1,1,1,1,1,1,1,1,1,1,1,1,1,1,1,1,1,6),(2,2),(0.,0.0142857142857143,
0.0285714285714286,0.0428571428571429,0.0571428571428571,0.0714285714285714,
0.0857142857142857,0.1,0.114285714285714,0.128571428571429,0.142857142857143,
0.157142857142857,0.171428571428571,0.185714285714286,0.2,0.214285714285714,
0.228571428571429,0.242857142857143,0.257142857142857,0.271428571428571,
0.285714285714286,0.3,0.314285714285714,0.328571428571429,0.342857142857143,
0.357142857142857,0.371428571428571,0.385714285714286,0.4,0.414285714285714,
0.428571428571429,0.442857142857143,0.457142857142857,0.471428571428572,
0.485714285714286,0.5,0.514285714285714,0.528571428571429,0.542857142857143,
0.557142857142857,0.571428571428571,0.585714285714286,0.6,0.614285714285714,
0.628571428571428,0.642857142857142,0.657142857142857,0.671428571428571,
0.685714285714285,0.699999999999999,0.714285714285714,0.728571428571428,
0.742857142857142,0.757142857142856,0.771428571428571,0.785714285714285,
0.799999999999999,0.814285714285713,0.828571428571428,0.842857142857142,
0.857142857142856,0.87142857142857,0.885714285714284,0.899999999999999,
0.914285714285713,0.928571428571427,0.942857142857141,0.957142857142856,
0.97142857142857,0.985714285714284,1.),(0.,1.8),.UNSPECIFIED.);
#949=B_SPLINE_SURFACE_WITH_KNOTS('',5,1,((#20011,#20012),(#20013,#20014),
(#20015,#20016),(#20017,#20018),(#20019,#20020),(#20021,#20022),(#20023,
#20024),(#20025,#20026),(#20027,#20028),(#20029,#20030),(#20031,#20032),
(#20033,#20034),(#20035,#20036),(#20037,#20038),(#20039,#20040),(#20041,
#20042),(#20043,#20044),(#20045,#20046),(#20047,#20048),(#20049,#20050),
(#20051,#20052),(#20053,#20054),(#20055,#20056),(#20057,#20058),(#20059,
#20060),(#20061,#20062),(#20063,#20064),(#20065,#20066),(#20067,#20068),
(#20069,#20070),(#20071,#20072),(#20073,#20074),(#20075,#20076),(#20077,
#20078),(#20079,#20080),(#20081,#20082),(#20083,#20084),(#20085,#20086),
(#20087,#20088),(#20089,#20090),(#20091,#20092),(#20093,#20094),(#20095,
#20096),(#20097,#20098),(#20099,#20100),(#20101,#20102),(#20103,#20104),
(#20105,#20106),(#20107,#20108),(#20109,#20110),(#20111,#20112),(#20113,
#20114),(#20115,#20116),(#20117,#20118),(#20119,#20120),(#20121,#20122),
(#20123,#20124),(#20125,#20126),(#20127,#20128),(#20129,#20130),(#20131,
#20132),(#20133,#20134),(#20135,#20136),(#20137,#20138),(#20139,#20140),
(#20141,#20142),(#20143,#20144),(#20145,#20146),(#20147,#20148),(#20149,
#20150),(#20151,#20152),(#20153,#20154),(#20155,#20156),(#20157,#20158),
(#20159,#20160)),.UNSPECIFIED.,.F.,.F.,.F.,(6,1,1,1,1,1,1,1,1,1,1,1,1,1,
1,1,1,1,1,1,1,1,1,1,1,1,1,1,1,1,1,1,1,1,1,1,1,1,1,1,1,1,1,1,1,1,1,1,1,1,
1,1,1,1,1,1,1,1,1,1,1,1,1,1,1,1,1,1,1,1,6),(2,2),(-1.,-0.985714285714284,
-0.97142857142857,-0.957142857142856,-0.942857142857141,-0.928571428571427,
-0.914285714285713,-0.899999999999999,-0.885714285714284,-0.87142857142857,
-0.857142857142856,-0.842857142857142,-0.828571428571428,-0.814285714285713,
-0.799999999999999,-0.785714285714285,-0.771428571428571,-0.757142857142856,
-0.742857142857142,-0.728571428571428,-0.714285714285714,-0.699999999999999,
-0.685714285714285,-0.671428571428571,-0.657142857142857,-0.642857142857142,
-0.628571428571428,-0.614285714285714,-0.6,-0.585714285714286,-0.571428571428571,
-0.557142857142857,-0.542857142857143,-0.528571428571429,-0.514285714285714,
-0.5,-0.485714285714286,-0.471428571428572,-0.457142857142857,-0.442857142857143,
-0.428571428571429,-0.414285714285714,-0.4,-0.385714285714286,-0.371428571428571,
-0.357142857142857,-0.342857142857143,-0.328571428571429,-0.314285714285714,
-0.3,-0.285714285714286,-0.271428571428571,-0.257142857142857,-0.242857142857143,
-0.228571428571429,-0.214285714285714,-0.2,-0.185714285714286,-0.171428571428571,
-0.157142857142857,-0.142857142857143,-0.128571428571429,-0.114285714285714,
-0.1,-0.0857142857142857,-0.0714285714285714,-0.0571428571428571,-0.0428571428571429,
-0.0285714285714286,-0.0142857142857143,0.),(0.,1.8),.UNSPECIFIED.);
#950=B_SPLINE_SURFACE_WITH_KNOTS('',5,1,((#20319,#20320),(#20321,#20322),
(#20323,#20324),(#20325,#20326),(#20327,#20328),(#20329,#20330),(#20331,
#20332),(#20333,#20334),(#20335,#20336),(#20337,#20338),(#20339,#20340),
(#20341,#20342),(#20343,#20344),(#20345,#20346),(#20347,#20348),(#20349,
#20350),(#20351,#20352),(#20353,#20354),(#20355,#20356),(#20357,#20358),
(#20359,#20360),(#20361,#20362),(#20363,#20364),(#20365,#20366),(#20367,
#20368),(#20369,#20370),(#20371,#20372),(#20373,#20374),(#20375,#20376),
(#20377,#20378),(#20379,#20380),(#20381,#20382),(#20383,#20384),(#20385,
#20386),(#20387,#20388),(#20389,#20390),(#20391,#20392),(#20393,#20394),
(#20395,#20396),(#20397,#20398),(#20399,#20400),(#20401,#20402),(#20403,
#20404),(#20405,#20406),(#20407,#20408),(#20409,#20410),(#20411,#20412),
(#20413,#20414),(#20415,#20416),(#20417,#20418),(#20419,#20420),(#20421,
#20422),(#20423,#20424),(#20425,#20426),(#20427,#20428),(#20429,#20430),
(#20431,#20432),(#20433,#20434),(#20435,#20436),(#20437,#20438),(#20439,
#20440),(#20441,#20442),(#20443,#20444),(#20445,#20446),(#20447,#20448),
(#20449,#20450),(#20451,#20452),(#20453,#20454),(#20455,#20456),(#20457,
#20458),(#20459,#20460),(#20461,#20462),(#20463,#20464),(#20465,#20466),
(#20467,#20468)),.UNSPECIFIED.,.F.,.F.,.F.,(6,1,1,1,1,1,1,1,1,1,1,1,1,1,
1,1,1,1,1,1,1,1,1,1,1,1,1,1,1,1,1,1,1,1,1,1,1,1,1,1,1,1,1,1,1,1,1,1,1,1,
1,1,1,1,1,1,1,1,1,1,1,1,1,1,1,1,1,1,1,1,6),(2,2),(0.,0.0142857142857143,
0.0285714285714286,0.0428571428571429,0.0571428571428571,0.0714285714285714,
0.0857142857142857,0.1,0.114285714285714,0.128571428571429,0.142857142857143,
0.157142857142857,0.171428571428571,0.185714285714286,0.2,0.214285714285714,
0.228571428571429,0.242857142857143,0.257142857142857,0.271428571428571,
0.285714285714286,0.3,0.314285714285714,0.328571428571429,0.342857142857143,
0.357142857142857,0.371428571428571,0.385714285714286,0.4,0.414285714285714,
0.428571428571429,0.442857142857143,0.457142857142857,0.471428571428572,
0.485714285714286,0.5,0.514285714285714,0.528571428571429,0.542857142857143,
0.557142857142857,0.571428571428571,0.585714285714286,0.6,0.614285714285714,
0.628571428571428,0.642857142857142,0.657142857142857,0.671428571428571,
0.685714285714285,0.699999999999999,0.714285714285714,0.728571428571428,
0.742857142857142,0.757142857142856,0.771428571428571,0.785714285714285,
0.799999999999999,0.814285714285713,0.828571428571428,0.842857142857142,
0.857142857142856,0.87142857142857,0.885714285714284,0.899999999999999,
0.914285714285713,0.928571428571427,0.942857142857141,0.957142857142856,
0.97142857142857,0.985714285714284,1.),(0.,1.8),.UNSPECIFIED.);
#951=B_SPLINE_SURFACE_WITH_KNOTS('',5,1,((#20617,#20618),(#20619,#20620),
(#20621,#20622),(#20623,#20624),(#20625,#20626),(#20627,#20628),(#20629,
#20630),(#20631,#20632),(#20633,#20634),(#20635,#20636),(#20637,#20638),
(#20639,#20640),(#20641,#20642),(#20643,#20644),(#20645,#20646),(#20647,
#20648),(#20649,#20650),(#20651,#20652),(#20653,#20654),(#20655,#20656),
(#20657,#20658),(#20659,#20660),(#20661,#20662),(#20663,#20664),(#20665,
#20666),(#20667,#20668),(#20669,#20670),(#20671,#20672),(#20673,#20674),
(#20675,#20676),(#20677,#20678),(#20679,#20680),(#20681,#20682),(#20683,
#20684),(#20685,#20686),(#20687,#20688),(#20689,#20690),(#20691,#20692),
(#20693,#20694),(#20695,#20696),(#20697,#20698),(#20699,#20700),(#20701,
#20702),(#20703,#20704),(#20705,#20706),(#20707,#20708),(#20709,#20710),
(#20711,#20712),(#20713,#20714),(#20715,#20716),(#20717,#20718),(#20719,
#20720),(#20721,#20722),(#20723,#20724),(#20725,#20726),(#20727,#20728),
(#20729,#20730),(#20731,#20732),(#20733,#20734),(#20735,#20736),(#20737,
#20738),(#20739,#20740),(#20741,#20742),(#20743,#20744),(#20745,#20746),
(#20747,#20748),(#20749,#20750),(#20751,#20752),(#20753,#20754),(#20755,
#20756),(#20757,#20758),(#20759,#20760),(#20761,#20762),(#20763,#20764),
(#20765,#20766)),.UNSPECIFIED.,.F.,.F.,.F.,(6,1,1,1,1,1,1,1,1,1,1,1,1,1,
1,1,1,1,1,1,1,1,1,1,1,1,1,1,1,1,1,1,1,1,1,1,1,1,1,1,1,1,1,1,1,1,1,1,1,1,
1,1,1,1,1,1,1,1,1,1,1,1,1,1,1,1,1,1,1,1,6),(2,2),(-1.,-0.985714285714284,
-0.97142857142857,-0.957142857142856,-0.942857142857141,-0.928571428571427,
-0.914285714285713,-0.899999999999999,-0.885714285714284,-0.87142857142857,
-0.857142857142856,-0.842857142857142,-0.828571428571428,-0.814285714285713,
-0.799999999999999,-0.785714285714285,-0.771428571428571,-0.757142857142856,
-0.742857142857142,-0.728571428571428,-0.714285714285714,-0.699999999999999,
-0.685714285714285,-0.671428571428571,-0.657142857142857,-0.642857142857142,
-0.628571428571428,-0.614285714285714,-0.6,-0.585714285714286,-0.571428571428571,
-0.557142857142857,-0.542857142857143,-0.528571428571429,-0.514285714285714,
-0.5,-0.485714285714286,-0.471428571428572,-0.457142857142857,-0.442857142857143,
-0.428571428571429,-0.414285714285714,-0.4,-0.385714285714286,-0.371428571428571,
-0.357142857142857,-0.342857142857143,-0.328571428571429,-0.314285714285714,
-0.3,-0.285714285714286,-0.271428571428571,-0.257142857142857,-0.242857142857143,
-0.228571428571429,-0.214285714285714,-0.2,-0.185714285714286,-0.171428571428571,
-0.157142857142857,-0.142857142857143,-0.128571428571429,-0.114285714285714,
-0.1,-0.0857142857142857,-0.0714285714285714,-0.0571428571428571,-0.0428571428571429,
-0.0285714285714286,-0.0142857142857143,0.),(0.,1.8),.UNSPECIFIED.);
#952=B_SPLINE_SURFACE_WITH_KNOTS('',5,1,((#20925,#20926),(#20927,#20928),
(#20929,#20930),(#20931,#20932),(#20933,#20934),(#20935,#20936),(#20937,
#20938),(#20939,#20940),(#20941,#20942),(#20943,#20944),(#20945,#20946),
(#20947,#20948),(#20949,#20950),(#20951,#20952),(#20953,#20954),(#20955,
#20956),(#20957,#20958),(#20959,#20960),(#20961,#20962),(#20963,#20964),
(#20965,#20966),(#20967,#20968),(#20969,#20970),(#20971,#20972),(#20973,
#20974),(#20975,#20976),(#20977,#20978),(#20979,#20980),(#20981,#20982),
(#20983,#20984),(#20985,#20986),(#20987,#20988),(#20989,#20990),(#20991,
#20992),(#20993,#20994),(#20995,#20996),(#20997,#20998),(#20999,#21000),
(#21001,#21002),(#21003,#21004),(#21005,#21006),(#21007,#21008),(#21009,
#21010),(#21011,#21012),(#21013,#21014),(#21015,#21016),(#21017,#21018),
(#21019,#21020),(#21021,#21022),(#21023,#21024),(#21025,#21026),(#21027,
#21028),(#21029,#21030),(#21031,#21032),(#21033,#21034),(#21035,#21036),
(#21037,#21038),(#21039,#21040),(#21041,#21042),(#21043,#21044),(#21045,
#21046),(#21047,#21048),(#21049,#21050),(#21051,#21052),(#21053,#21054),
(#21055,#21056),(#21057,#21058),(#21059,#21060),(#21061,#21062),(#21063,
#21064),(#21065,#21066),(#21067,#21068),(#21069,#21070),(#21071,#21072),
(#21073,#21074)),.UNSPECIFIED.,.F.,.F.,.F.,(6,1,1,1,1,1,1,1,1,1,1,1,1,1,
1,1,1,1,1,1,1,1,1,1,1,1,1,1,1,1,1,1,1,1,1,1,1,1,1,1,1,1,1,1,1,1,1,1,1,1,
1,1,1,1,1,1,1,1,1,1,1,1,1,1,1,1,1,1,1,1,6),(2,2),(0.,0.0142857142857143,
0.0285714285714286,0.0428571428571429,0.0571428571428571,0.0714285714285714,
0.0857142857142857,0.1,0.114285714285714,0.128571428571429,0.142857142857143,
0.157142857142857,0.171428571428571,0.185714285714286,0.2,0.214285714285714,
0.228571428571429,0.242857142857143,0.257142857142857,0.271428571428571,
0.285714285714286,0.3,0.314285714285714,0.328571428571429,0.342857142857143,
0.357142857142857,0.371428571428571,0.385714285714286,0.4,0.414285714285714,
0.428571428571429,0.442857142857143,0.457142857142857,0.471428571428572,
0.485714285714286,0.5,0.514285714285714,0.528571428571429,0.542857142857143,
0.557142857142857,0.571428571428571,0.585714285714286,0.6,0.614285714285714,
0.628571428571428,0.642857142857142,0.657142857142857,0.671428571428571,
0.685714285714285,0.699999999999999,0.714285714285714,0.728571428571428,
0.742857142857142,0.757142857142856,0.771428571428571,0.785714285714285,
0.799999999999999,0.814285714285713,0.828571428571428,0.842857142857142,
0.857142857142856,0.87142857142857,0.885714285714284,0.899999999999999,
0.914285714285713,0.928571428571427,0.942857142857141,0.957142857142856,
0.97142857142857,0.985714285714284,1.),(0.,1.8),.UNSPECIFIED.);
#953=B_SPLINE_SURFACE_WITH_KNOTS('',5,1,((#21223,#21224),(#21225,#21226),
(#21227,#21228),(#21229,#21230),(#21231,#21232),(#21233,#21234),(#21235,
#21236),(#21237,#21238),(#21239,#21240),(#21241,#21242),(#21243,#21244),
(#21245,#21246),(#21247,#21248),(#21249,#21250),(#21251,#21252),(#21253,
#21254),(#21255,#21256),(#21257,#21258),(#21259,#21260),(#21261,#21262),
(#21263,#21264),(#21265,#21266),(#21267,#21268),(#21269,#21270),(#21271,
#21272),(#21273,#21274),(#21275,#21276),(#21277,#21278),(#21279,#21280),
(#21281,#21282),(#21283,#21284),(#21285,#21286),(#21287,#21288),(#21289,
#21290),(#21291,#21292),(#21293,#21294),(#21295,#21296),(#21297,#21298),
(#21299,#21300),(#21301,#21302),(#21303,#21304),(#21305,#21306),(#21307,
#21308),(#21309,#21310),(#21311,#21312),(#21313,#21314),(#21315,#21316),
(#21317,#21318),(#21319,#21320),(#21321,#21322),(#21323,#21324),(#21325,
#21326),(#21327,#21328),(#21329,#21330),(#21331,#21332),(#21333,#21334),
(#21335,#21336),(#21337,#21338),(#21339,#21340),(#21341,#21342),(#21343,
#21344),(#21345,#21346),(#21347,#21348),(#21349,#21350),(#21351,#21352),
(#21353,#21354),(#21355,#21356),(#21357,#21358),(#21359,#21360),(#21361,
#21362),(#21363,#21364),(#21365,#21366),(#21367,#21368),(#21369,#21370),
(#21371,#21372)),.UNSPECIFIED.,.F.,.F.,.F.,(6,1,1,1,1,1,1,1,1,1,1,1,1,1,
1,1,1,1,1,1,1,1,1,1,1,1,1,1,1,1,1,1,1,1,1,1,1,1,1,1,1,1,1,1,1,1,1,1,1,1,
1,1,1,1,1,1,1,1,1,1,1,1,1,1,1,1,1,1,1,1,6),(2,2),(-1.,-0.985714285714284,
-0.97142857142857,-0.957142857142856,-0.942857142857141,-0.928571428571427,
-0.914285714285713,-0.899999999999999,-0.885714285714284,-0.87142857142857,
-0.857142857142856,-0.842857142857142,-0.828571428571428,-0.814285714285713,
-0.799999999999999,-0.785714285714285,-0.771428571428571,-0.757142857142856,
-0.742857142857142,-0.728571428571428,-0.714285714285714,-0.699999999999999,
-0.685714285714285,-0.671428571428571,-0.657142857142857,-0.642857142857142,
-0.628571428571428,-0.614285714285714,-0.6,-0.585714285714286,-0.571428571428571,
-0.557142857142857,-0.542857142857143,-0.528571428571429,-0.514285714285714,
-0.5,-0.485714285714286,-0.471428571428572,-0.457142857142857,-0.442857142857143,
-0.428571428571429,-0.414285714285714,-0.4,-0.385714285714286,-0.371428571428571,
-0.357142857142857,-0.342857142857143,-0.328571428571429,-0.314285714285714,
-0.3,-0.285714285714286,-0.271428571428571,-0.257142857142857,-0.242857142857143,
-0.228571428571429,-0.214285714285714,-0.2,-0.185714285714286,-0.171428571428571,
-0.157142857142857,-0.142857142857143,-0.128571428571429,-0.114285714285714,
-0.1,-0.0857142857142857,-0.0714285714285714,-0.0571428571428571,-0.0428571428571429,
-0.0285714285714286,-0.0142857142857143,0.),(0.,1.8),.UNSPECIFIED.);
#954=B_SPLINE_SURFACE_WITH_KNOTS('',5,1,((#21531,#21532),(#21533,#21534),
(#21535,#21536),(#21537,#21538),(#21539,#21540),(#21541,#21542),(#21543,
#21544),(#21545,#21546),(#21547,#21548),(#21549,#21550),(#21551,#21552),
(#21553,#21554),(#21555,#21556),(#21557,#21558),(#21559,#21560),(#21561,
#21562),(#21563,#21564),(#21565,#21566),(#21567,#21568),(#21569,#21570),
(#21571,#21572),(#21573,#21574),(#21575,#21576),(#21577,#21578),(#21579,
#21580),(#21581,#21582),(#21583,#21584),(#21585,#21586),(#21587,#21588),
(#21589,#21590),(#21591,#21592),(#21593,#21594),(#21595,#21596),(#21597,
#21598),(#21599,#21600),(#21601,#21602),(#21603,#21604),(#21605,#21606),
(#21607,#21608),(#21609,#21610),(#21611,#21612),(#21613,#21614),(#21615,
#21616),(#21617,#21618),(#21619,#21620),(#21621,#21622),(#21623,#21624),
(#21625,#21626),(#21627,#21628),(#21629,#21630),(#21631,#21632),(#21633,
#21634),(#21635,#21636),(#21637,#21638),(#21639,#21640),(#21641,#21642),
(#21643,#21644),(#21645,#21646),(#21647,#21648),(#21649,#21650),(#21651,
#21652),(#21653,#21654),(#21655,#21656),(#21657,#21658),(#21659,#21660),
(#21661,#21662),(#21663,#21664),(#21665,#21666),(#21667,#21668),(#21669,
#21670),(#21671,#21672),(#21673,#21674),(#21675,#21676),(#21677,#21678),
(#21679,#21680)),.UNSPECIFIED.,.F.,.F.,.F.,(6,1,1,1,1,1,1,1,1,1,1,1,1,1,
1,1,1,1,1,1,1,1,1,1,1,1,1,1,1,1,1,1,1,1,1,1,1,1,1,1,1,1,1,1,1,1,1,1,1,1,
1,1,1,1,1,1,1,1,1,1,1,1,1,1,1,1,1,1,1,1,6),(2,2),(0.,0.0142857142857143,
0.0285714285714286,0.0428571428571429,0.0571428571428571,0.0714285714285714,
0.0857142857142857,0.1,0.114285714285714,0.128571428571429,0.142857142857143,
0.157142857142857,0.171428571428571,0.185714285714286,0.2,0.214285714285714,
0.228571428571429,0.242857142857143,0.257142857142857,0.271428571428571,
0.285714285714286,0.3,0.314285714285714,0.328571428571429,0.342857142857143,
0.357142857142857,0.371428571428571,0.385714285714286,0.4,0.414285714285714,
0.428571428571429,0.442857142857143,0.457142857142857,0.471428571428572,
0.485714285714286,0.5,0.514285714285714,0.528571428571429,0.542857142857143,
0.557142857142857,0.571428571428571,0.585714285714286,0.6,0.614285714285714,
0.628571428571428,0.642857142857142,0.657142857142857,0.671428571428571,
0.685714285714285,0.699999999999999,0.714285714285714,0.728571428571428,
0.742857142857142,0.757142857142856,0.771428571428571,0.785714285714285,
0.799999999999999,0.814285714285713,0.828571428571428,0.842857142857142,
0.857142857142856,0.87142857142857,0.885714285714284,0.899999999999999,
0.914285714285713,0.928571428571427,0.942857142857141,0.957142857142856,
0.97142857142857,0.985714285714284,1.),(0.,1.8),.UNSPECIFIED.);
#955=B_SPLINE_SURFACE_WITH_KNOTS('',5,1,((#21829,#21830),(#21831,#21832),
(#21833,#21834),(#21835,#21836),(#21837,#21838),(#21839,#21840),(#21841,
#21842),(#21843,#21844),(#21845,#21846),(#21847,#21848),(#21849,#21850),
(#21851,#21852),(#21853,#21854),(#21855,#21856),(#21857,#21858),(#21859,
#21860),(#21861,#21862),(#21863,#21864),(#21865,#21866),(#21867,#21868),
(#21869,#21870),(#21871,#21872),(#21873,#21874),(#21875,#21876),(#21877,
#21878),(#21879,#21880),(#21881,#21882),(#21883,#21884),(#21885,#21886),
(#21887,#21888),(#21889,#21890),(#21891,#21892),(#21893,#21894),(#21895,
#21896),(#21897,#21898),(#21899,#21900),(#21901,#21902),(#21903,#21904),
(#21905,#21906),(#21907,#21908),(#21909,#21910),(#21911,#21912),(#21913,
#21914),(#21915,#21916),(#21917,#21918),(#21919,#21920),(#21921,#21922),
(#21923,#21924),(#21925,#21926),(#21927,#21928),(#21929,#21930),(#21931,
#21932),(#21933,#21934),(#21935,#21936),(#21937,#21938),(#21939,#21940),
(#21941,#21942),(#21943,#21944),(#21945,#21946),(#21947,#21948),(#21949,
#21950),(#21951,#21952),(#21953,#21954),(#21955,#21956),(#21957,#21958),
(#21959,#21960),(#21961,#21962),(#21963,#21964),(#21965,#21966),(#21967,
#21968),(#21969,#21970),(#21971,#21972),(#21973,#21974),(#21975,#21976),
(#21977,#21978)),.UNSPECIFIED.,.F.,.F.,.F.,(6,1,1,1,1,1,1,1,1,1,1,1,1,1,
1,1,1,1,1,1,1,1,1,1,1,1,1,1,1,1,1,1,1,1,1,1,1,1,1,1,1,1,1,1,1,1,1,1,1,1,
1,1,1,1,1,1,1,1,1,1,1,1,1,1,1,1,1,1,1,1,6),(2,2),(-1.,-0.985714285714284,
-0.97142857142857,-0.957142857142856,-0.942857142857141,-0.928571428571427,
-0.914285714285713,-0.899999999999999,-0.885714285714284,-0.87142857142857,
-0.857142857142856,-0.842857142857142,-0.828571428571428,-0.814285714285713,
-0.799999999999999,-0.785714285714285,-0.771428571428571,-0.757142857142856,
-0.742857142857142,-0.728571428571428,-0.714285714285714,-0.699999999999999,
-0.685714285714285,-0.671428571428571,-0.657142857142857,-0.642857142857142,
-0.628571428571428,-0.614285714285714,-0.6,-0.585714285714286,-0.571428571428571,
-0.557142857142857,-0.542857142857143,-0.528571428571429,-0.514285714285714,
-0.5,-0.485714285714286,-0.471428571428572,-0.457142857142857,-0.442857142857143,
-0.428571428571429,-0.414285714285714,-0.4,-0.385714285714286,-0.371428571428571,
-0.357142857142857,-0.342857142857143,-0.328571428571429,-0.314285714285714,
-0.3,-0.285714285714286,-0.271428571428571,-0.257142857142857,-0.242857142857143,
-0.228571428571429,-0.214285714285714,-0.2,-0.185714285714286,-0.171428571428571,
-0.157142857142857,-0.142857142857143,-0.128571428571429,-0.114285714285714,
-0.1,-0.0857142857142857,-0.0714285714285714,-0.0571428571428571,-0.0428571428571429,
-0.0285714285714286,-0.0142857142857143,0.),(0.,1.8),.UNSPECIFIED.);
#956=B_SPLINE_SURFACE_WITH_KNOTS('',5,1,((#22137,#22138),(#22139,#22140),
(#22141,#22142),(#22143,#22144),(#22145,#22146),(#22147,#22148),(#22149,
#22150),(#22151,#22152),(#22153,#22154),(#22155,#22156),(#22157,#22158),
(#22159,#22160),(#22161,#22162),(#22163,#22164),(#22165,#22166),(#22167,
#22168),(#22169,#22170),(#22171,#22172),(#22173,#22174),(#22175,#22176),
(#22177,#22178),(#22179,#22180),(#22181,#22182),(#22183,#22184),(#22185,
#22186),(#22187,#22188),(#22189,#22190),(#22191,#22192),(#22193,#22194),
(#22195,#22196),(#22197,#22198),(#22199,#22200),(#22201,#22202),(#22203,
#22204),(#22205,#22206),(#22207,#22208),(#22209,#22210),(#22211,#22212),
(#22213,#22214),(#22215,#22216),(#22217,#22218),(#22219,#22220),(#22221,
#22222),(#22223,#22224),(#22225,#22226),(#22227,#22228),(#22229,#22230),
(#22231,#22232),(#22233,#22234),(#22235,#22236),(#22237,#22238),(#22239,
#22240),(#22241,#22242),(#22243,#22244),(#22245,#22246),(#22247,#22248),
(#22249,#22250),(#22251,#22252),(#22253,#22254),(#22255,#22256),(#22257,
#22258),(#22259,#22260),(#22261,#22262),(#22263,#22264),(#22265,#22266),
(#22267,#22268),(#22269,#22270),(#22271,#22272),(#22273,#22274),(#22275,
#22276),(#22277,#22278),(#22279,#22280),(#22281,#22282),(#22283,#22284),
(#22285,#22286)),.UNSPECIFIED.,.F.,.F.,.F.,(6,1,1,1,1,1,1,1,1,1,1,1,1,1,
1,1,1,1,1,1,1,1,1,1,1,1,1,1,1,1,1,1,1,1,1,1,1,1,1,1,1,1,1,1,1,1,1,1,1,1,
1,1,1,1,1,1,1,1,1,1,1,1,1,1,1,1,1,1,1,1,6),(2,2),(0.,0.0142857142857143,
0.0285714285714286,0.0428571428571429,0.0571428571428571,0.0714285714285714,
0.0857142857142857,0.1,0.114285714285714,0.128571428571429,0.142857142857143,
0.157142857142857,0.171428571428571,0.185714285714286,0.2,0.214285714285714,
0.228571428571429,0.242857142857143,0.257142857142857,0.271428571428571,
0.285714285714286,0.3,0.314285714285714,0.328571428571429,0.342857142857143,
0.357142857142857,0.371428571428571,0.385714285714286,0.4,0.414285714285714,
0.428571428571429,0.442857142857143,0.457142857142857,0.471428571428572,
0.485714285714286,0.5,0.514285714285714,0.528571428571429,0.542857142857143,
0.557142857142857,0.571428571428571,0.585714285714286,0.6,0.614285714285714,
0.628571428571428,0.642857142857142,0.657142857142857,0.671428571428571,
0.685714285714285,0.699999999999999,0.714285714285714,0.728571428571428,
0.742857142857142,0.757142857142856,0.771428571428571,0.785714285714285,
0.799999999999999,0.814285714285713,0.828571428571428,0.842857142857142,
0.857142857142856,0.87142857142857,0.885714285714284,0.899999999999999,
0.914285714285713,0.928571428571427,0.942857142857141,0.957142857142856,
0.97142857142857,0.985714285714284,1.),(0.,1.8),.UNSPECIFIED.);
#957=B_SPLINE_SURFACE_WITH_KNOTS('',5,1,((#22435,#22436),(#22437,#22438),
(#22439,#22440),(#22441,#22442),(#22443,#22444),(#22445,#22446),(#22447,
#22448),(#22449,#22450),(#22451,#22452),(#22453,#22454),(#22455,#22456),
(#22457,#22458),(#22459,#22460),(#22461,#22462),(#22463,#22464),(#22465,
#22466),(#22467,#22468),(#22469,#22470),(#22471,#22472),(#22473,#22474),
(#22475,#22476),(#22477,#22478),(#22479,#22480),(#22481,#22482),(#22483,
#22484),(#22485,#22486),(#22487,#22488),(#22489,#22490),(#22491,#22492),
(#22493,#22494),(#22495,#22496),(#22497,#22498),(#22499,#22500),(#22501,
#22502),(#22503,#22504),(#22505,#22506),(#22507,#22508),(#22509,#22510),
(#22511,#22512),(#22513,#22514),(#22515,#22516),(#22517,#22518),(#22519,
#22520),(#22521,#22522),(#22523,#22524),(#22525,#22526),(#22527,#22528),
(#22529,#22530),(#22531,#22532),(#22533,#22534),(#22535,#22536),(#22537,
#22538),(#22539,#22540),(#22541,#22542),(#22543,#22544),(#22545,#22546),
(#22547,#22548),(#22549,#22550),(#22551,#22552),(#22553,#22554),(#22555,
#22556),(#22557,#22558),(#22559,#22560),(#22561,#22562),(#22563,#22564),
(#22565,#22566),(#22567,#22568),(#22569,#22570),(#22571,#22572),(#22573,
#22574),(#22575,#22576),(#22577,#22578),(#22579,#22580),(#22581,#22582),
(#22583,#22584)),.UNSPECIFIED.,.F.,.F.,.F.,(6,1,1,1,1,1,1,1,1,1,1,1,1,1,
1,1,1,1,1,1,1,1,1,1,1,1,1,1,1,1,1,1,1,1,1,1,1,1,1,1,1,1,1,1,1,1,1,1,1,1,
1,1,1,1,1,1,1,1,1,1,1,1,1,1,1,1,1,1,1,1,6),(2,2),(-1.,-0.985714285714284,
-0.97142857142857,-0.957142857142856,-0.942857142857141,-0.928571428571427,
-0.914285714285713,-0.899999999999999,-0.885714285714284,-0.87142857142857,
-0.857142857142856,-0.842857142857142,-0.828571428571428,-0.814285714285713,
-0.799999999999999,-0.785714285714285,-0.771428571428571,-0.757142857142856,
-0.742857142857142,-0.728571428571428,-0.714285714285714,-0.699999999999999,
-0.685714285714285,-0.671428571428571,-0.657142857142857,-0.642857142857142,
-0.628571428571428,-0.614285714285714,-0.6,-0.585714285714286,-0.571428571428571,
-0.557142857142857,-0.542857142857143,-0.528571428571429,-0.514285714285714,
-0.5,-0.485714285714286,-0.471428571428572,-0.457142857142857,-0.442857142857143,
-0.428571428571429,-0.414285714285714,-0.4,-0.385714285714286,-0.371428571428571,
-0.357142857142857,-0.342857142857143,-0.328571428571429,-0.314285714285714,
-0.3,-0.285714285714286,-0.271428571428571,-0.257142857142857,-0.242857142857143,
-0.228571428571429,-0.214285714285714,-0.2,-0.185714285714286,-0.171428571428571,
-0.157142857142857,-0.142857142857143,-0.128571428571429,-0.114285714285714,
-0.1,-0.0857142857142857,-0.0714285714285714,-0.0571428571428571,-0.0428571428571429,
-0.0285714285714286,-0.0142857142857143,0.),(0.,1.8),.UNSPECIFIED.);
#958=B_SPLINE_SURFACE_WITH_KNOTS('',5,1,((#22743,#22744),(#22745,#22746),
(#22747,#22748),(#22749,#22750),(#22751,#22752),(#22753,#22754),(#22755,
#22756),(#22757,#22758),(#22759,#22760),(#22761,#22762),(#22763,#22764),
(#22765,#22766),(#22767,#22768),(#22769,#22770),(#22771,#22772),(#22773,
#22774),(#22775,#22776),(#22777,#22778),(#22779,#22780),(#22781,#22782),
(#22783,#22784),(#22785,#22786),(#22787,#22788),(#22789,#22790),(#22791,
#22792),(#22793,#22794),(#22795,#22796),(#22797,#22798),(#22799,#22800),
(#22801,#22802),(#22803,#22804),(#22805,#22806),(#22807,#22808),(#22809,
#22810),(#22811,#22812),(#22813,#22814),(#22815,#22816),(#22817,#22818),
(#22819,#22820),(#22821,#22822),(#22823,#22824),(#22825,#22826),(#22827,
#22828),(#22829,#22830),(#22831,#22832),(#22833,#22834),(#22835,#22836),
(#22837,#22838),(#22839,#22840),(#22841,#22842),(#22843,#22844),(#22845,
#22846),(#22847,#22848),(#22849,#22850),(#22851,#22852),(#22853,#22854),
(#22855,#22856),(#22857,#22858),(#22859,#22860),(#22861,#22862),(#22863,
#22864),(#22865,#22866),(#22867,#22868),(#22869,#22870),(#22871,#22872),
(#22873,#22874),(#22875,#22876),(#22877,#22878),(#22879,#22880),(#22881,
#22882),(#22883,#22884),(#22885,#22886),(#22887,#22888),(#22889,#22890),
(#22891,#22892)),.UNSPECIFIED.,.F.,.F.,.F.,(6,1,1,1,1,1,1,1,1,1,1,1,1,1,
1,1,1,1,1,1,1,1,1,1,1,1,1,1,1,1,1,1,1,1,1,1,1,1,1,1,1,1,1,1,1,1,1,1,1,1,
1,1,1,1,1,1,1,1,1,1,1,1,1,1,1,1,1,1,1,1,6),(2,2),(0.,0.0142857142857143,
0.0285714285714286,0.0428571428571429,0.0571428571428571,0.0714285714285714,
0.0857142857142857,0.1,0.114285714285714,0.128571428571429,0.142857142857143,
0.157142857142857,0.171428571428571,0.185714285714286,0.2,0.214285714285714,
0.228571428571429,0.242857142857143,0.257142857142857,0.271428571428571,
0.285714285714286,0.3,0.314285714285714,0.328571428571429,0.342857142857143,
0.357142857142857,0.371428571428571,0.385714285714286,0.4,0.414285714285714,
0.428571428571429,0.442857142857143,0.457142857142857,0.471428571428572,
0.485714285714286,0.5,0.514285714285714,0.528571428571429,0.542857142857143,
0.557142857142857,0.571428571428571,0.585714285714286,0.6,0.614285714285714,
0.628571428571428,0.642857142857142,0.657142857142857,0.671428571428571,
0.685714285714285,0.699999999999999,0.714285714285714,0.728571428571428,
0.742857142857142,0.757142857142856,0.771428571428571,0.785714285714285,
0.799999999999999,0.814285714285713,0.828571428571428,0.842857142857142,
0.857142857142856,0.87142857142857,0.885714285714284,0.899999999999999,
0.914285714285713,0.928571428571427,0.942857142857141,0.957142857142856,
0.97142857142857,0.985714285714284,1.),(0.,1.8),.UNSPECIFIED.);
#959=B_SPLINE_SURFACE_WITH_KNOTS('',5,1,((#23041,#23042),(#23043,#23044),
(#23045,#23046),(#23047,#23048),(#23049,#23050),(#23051,#23052),(#23053,
#23054),(#23055,#23056),(#23057,#23058),(#23059,#23060),(#23061,#23062),
(#23063,#23064),(#23065,#23066),(#23067,#23068),(#23069,#23070),(#23071,
#23072),(#23073,#23074),(#23075,#23076),(#23077,#23078),(#23079,#23080),
(#23081,#23082),(#23083,#23084),(#23085,#23086),(#23087,#23088),(#23089,
#23090),(#23091,#23092),(#23093,#23094),(#23095,#23096),(#23097,#23098),
(#23099,#23100),(#23101,#23102),(#23103,#23104),(#23105,#23106),(#23107,
#23108),(#23109,#23110),(#23111,#23112),(#23113,#23114),(#23115,#23116),
(#23117,#23118),(#23119,#23120),(#23121,#23122),(#23123,#23124),(#23125,
#23126),(#23127,#23128),(#23129,#23130),(#23131,#23132),(#23133,#23134),
(#23135,#23136),(#23137,#23138),(#23139,#23140),(#23141,#23142),(#23143,
#23144),(#23145,#23146),(#23147,#23148),(#23149,#23150),(#23151,#23152),
(#23153,#23154),(#23155,#23156),(#23157,#23158),(#23159,#23160),(#23161,
#23162),(#23163,#23164),(#23165,#23166),(#23167,#23168),(#23169,#23170),
(#23171,#23172),(#23173,#23174),(#23175,#23176),(#23177,#23178),(#23179,
#23180),(#23181,#23182),(#23183,#23184),(#23185,#23186),(#23187,#23188),
(#23189,#23190)),.UNSPECIFIED.,.F.,.F.,.F.,(6,1,1,1,1,1,1,1,1,1,1,1,1,1,
1,1,1,1,1,1,1,1,1,1,1,1,1,1,1,1,1,1,1,1,1,1,1,1,1,1,1,1,1,1,1,1,1,1,1,1,
1,1,1,1,1,1,1,1,1,1,1,1,1,1,1,1,1,1,1,1,6),(2,2),(-1.,-0.985714285714284,
-0.97142857142857,-0.957142857142856,-0.942857142857141,-0.928571428571427,
-0.914285714285713,-0.899999999999999,-0.885714285714284,-0.87142857142857,
-0.857142857142856,-0.842857142857142,-0.828571428571428,-0.814285714285713,
-0.799999999999999,-0.785714285714285,-0.771428571428571,-0.757142857142856,
-0.742857142857142,-0.728571428571428,-0.714285714285714,-0.699999999999999,
-0.685714285714285,-0.671428571428571,-0.657142857142857,-0.642857142857142,
-0.628571428571428,-0.614285714285714,-0.6,-0.585714285714286,-0.571428571428571,
-0.557142857142857,-0.542857142857143,-0.528571428571429,-0.514285714285714,
-0.5,-0.485714285714286,-0.471428571428572,-0.457142857142857,-0.442857142857143,
-0.428571428571429,-0.414285714285714,-0.4,-0.385714285714286,-0.371428571428571,
-0.357142857142857,-0.342857142857143,-0.328571428571429,-0.314285714285714,
-0.3,-0.285714285714286,-0.271428571428571,-0.257142857142857,-0.242857142857143,
-0.228571428571429,-0.214285714285714,-0.2,-0.185714285714286,-0.171428571428571,
-0.157142857142857,-0.142857142857143,-0.128571428571429,-0.114285714285714,
-0.1,-0.0857142857142857,-0.0714285714285714,-0.0571428571428571,-0.0428571428571429,
-0.0285714285714286,-0.0142857142857143,0.),(0.,1.8),.UNSPECIFIED.);
#960=B_SPLINE_SURFACE_WITH_KNOTS('',5,1,((#23349,#23350),(#23351,#23352),
(#23353,#23354),(#23355,#23356),(#23357,#23358),(#23359,#23360),(#23361,
#23362),(#23363,#23364),(#23365,#23366),(#23367,#23368),(#23369,#23370),
(#23371,#23372),(#23373,#23374),(#23375,#23376),(#23377,#23378),(#23379,
#23380),(#23381,#23382),(#23383,#23384),(#23385,#23386),(#23387,#23388),
(#23389,#23390),(#23391,#23392),(#23393,#23394),(#23395,#23396),(#23397,
#23398),(#23399,#23400),(#23401,#23402),(#23403,#23404),(#23405,#23406),
(#23407,#23408),(#23409,#23410),(#23411,#23412),(#23413,#23414),(#23415,
#23416),(#23417,#23418),(#23419,#23420),(#23421,#23422),(#23423,#23424),
(#23425,#23426),(#23427,#23428),(#23429,#23430),(#23431,#23432),(#23433,
#23434),(#23435,#23436),(#23437,#23438),(#23439,#23440),(#23441,#23442),
(#23443,#23444),(#23445,#23446),(#23447,#23448),(#23449,#23450),(#23451,
#23452),(#23453,#23454),(#23455,#23456),(#23457,#23458),(#23459,#23460),
(#23461,#23462),(#23463,#23464),(#23465,#23466),(#23467,#23468),(#23469,
#23470),(#23471,#23472),(#23473,#23474),(#23475,#23476),(#23477,#23478),
(#23479,#23480),(#23481,#23482),(#23483,#23484),(#23485,#23486),(#23487,
#23488),(#23489,#23490),(#23491,#23492),(#23493,#23494),(#23495,#23496),
(#23497,#23498)),.UNSPECIFIED.,.F.,.F.,.F.,(6,1,1,1,1,1,1,1,1,1,1,1,1,1,
1,1,1,1,1,1,1,1,1,1,1,1,1,1,1,1,1,1,1,1,1,1,1,1,1,1,1,1,1,1,1,1,1,1,1,1,
1,1,1,1,1,1,1,1,1,1,1,1,1,1,1,1,1,1,1,1,6),(2,2),(0.,0.0142857142857143,
0.0285714285714286,0.0428571428571429,0.0571428571428571,0.0714285714285714,
0.0857142857142857,0.1,0.114285714285714,0.128571428571429,0.142857142857143,
0.157142857142857,0.171428571428571,0.185714285714286,0.2,0.214285714285714,
0.228571428571429,0.242857142857143,0.257142857142857,0.271428571428571,
0.285714285714286,0.3,0.314285714285714,0.328571428571429,0.342857142857143,
0.357142857142857,0.371428571428571,0.385714285714286,0.4,0.414285714285714,
0.428571428571429,0.442857142857143,0.457142857142857,0.471428571428572,
0.485714285714286,0.5,0.514285714285714,0.528571428571429,0.542857142857143,
0.557142857142857,0.571428571428571,0.585714285714286,0.6,0.614285714285714,
0.628571428571428,0.642857142857142,0.657142857142857,0.671428571428571,
0.685714285714285,0.699999999999999,0.714285714285714,0.728571428571428,
0.742857142857142,0.757142857142856,0.771428571428571,0.785714285714285,
0.799999999999999,0.814285714285713,0.828571428571428,0.842857142857142,
0.857142857142856,0.87142857142857,0.885714285714284,0.899999999999999,
0.914285714285713,0.928571428571427,0.942857142857141,0.957142857142856,
0.97142857142857,0.985714285714284,1.),(0.,1.8),.UNSPECIFIED.);
#961=B_SPLINE_SURFACE_WITH_KNOTS('',5,1,((#23647,#23648),(#23649,#23650),
(#23651,#23652),(#23653,#23654),(#23655,#23656),(#23657,#23658),(#23659,
#23660),(#23661,#23662),(#23663,#23664),(#23665,#23666),(#23667,#23668),
(#23669,#23670),(#23671,#23672),(#23673,#23674),(#23675,#23676),(#23677,
#23678),(#23679,#23680),(#23681,#23682),(#23683,#23684),(#23685,#23686),
(#23687,#23688),(#23689,#23690),(#23691,#23692),(#23693,#23694),(#23695,
#23696),(#23697,#23698),(#23699,#23700),(#23701,#23702),(#23703,#23704),
(#23705,#23706),(#23707,#23708),(#23709,#23710),(#23711,#23712),(#23713,
#23714),(#23715,#23716),(#23717,#23718),(#23719,#23720),(#23721,#23722),
(#23723,#23724),(#23725,#23726),(#23727,#23728),(#23729,#23730),(#23731,
#23732),(#23733,#23734),(#23735,#23736),(#23737,#23738),(#23739,#23740),
(#23741,#23742),(#23743,#23744),(#23745,#23746),(#23747,#23748),(#23749,
#23750),(#23751,#23752),(#23753,#23754),(#23755,#23756),(#23757,#23758),
(#23759,#23760),(#23761,#23762),(#23763,#23764),(#23765,#23766),(#23767,
#23768),(#23769,#23770),(#23771,#23772),(#23773,#23774),(#23775,#23776),
(#23777,#23778),(#23779,#23780),(#23781,#23782),(#23783,#23784),(#23785,
#23786),(#23787,#23788),(#23789,#23790),(#23791,#23792),(#23793,#23794),
(#23795,#23796)),.UNSPECIFIED.,.F.,.F.,.F.,(6,1,1,1,1,1,1,1,1,1,1,1,1,1,
1,1,1,1,1,1,1,1,1,1,1,1,1,1,1,1,1,1,1,1,1,1,1,1,1,1,1,1,1,1,1,1,1,1,1,1,
1,1,1,1,1,1,1,1,1,1,1,1,1,1,1,1,1,1,1,1,6),(2,2),(-1.,-0.985714285714284,
-0.97142857142857,-0.957142857142856,-0.942857142857141,-0.928571428571427,
-0.914285714285713,-0.899999999999999,-0.885714285714284,-0.87142857142857,
-0.857142857142856,-0.842857142857142,-0.828571428571428,-0.814285714285713,
-0.799999999999999,-0.785714285714285,-0.771428571428571,-0.757142857142856,
-0.742857142857142,-0.728571428571428,-0.714285714285714,-0.699999999999999,
-0.685714285714285,-0.671428571428571,-0.657142857142857,-0.642857142857142,
-0.628571428571428,-0.614285714285714,-0.6,-0.585714285714286,-0.571428571428571,
-0.557142857142857,-0.542857142857143,-0.528571428571429,-0.514285714285714,
-0.5,-0.485714285714286,-0.471428571428572,-0.457142857142857,-0.442857142857143,
-0.428571428571429,-0.414285714285714,-0.4,-0.385714285714286,-0.371428571428571,
-0.357142857142857,-0.342857142857143,-0.328571428571429,-0.314285714285714,
-0.3,-0.285714285714286,-0.271428571428571,-0.257142857142857,-0.242857142857143,
-0.228571428571429,-0.214285714285714,-0.2,-0.185714285714286,-0.171428571428571,
-0.157142857142857,-0.142857142857143,-0.128571428571429,-0.114285714285714,
-0.1,-0.0857142857142857,-0.0714285714285714,-0.0571428571428571,-0.0428571428571429,
-0.0285714285714286,-0.0142857142857143,0.),(0.,1.8),.UNSPECIFIED.);
#962=B_SPLINE_SURFACE_WITH_KNOTS('',5,1,((#23955,#23956),(#23957,#23958),
(#23959,#23960),(#23961,#23962),(#23963,#23964),(#23965,#23966),(#23967,
#23968),(#23969,#23970),(#23971,#23972),(#23973,#23974),(#23975,#23976),
(#23977,#23978),(#23979,#23980),(#23981,#23982),(#23983,#23984),(#23985,
#23986),(#23987,#23988),(#23989,#23990),(#23991,#23992),(#23993,#23994),
(#23995,#23996),(#23997,#23998),(#23999,#24000),(#24001,#24002),(#24003,
#24004),(#24005,#24006),(#24007,#24008),(#24009,#24010),(#24011,#24012),
(#24013,#24014),(#24015,#24016),(#24017,#24018),(#24019,#24020),(#24021,
#24022),(#24023,#24024),(#24025,#24026),(#24027,#24028),(#24029,#24030),
(#24031,#24032),(#24033,#24034),(#24035,#24036),(#24037,#24038),(#24039,
#24040),(#24041,#24042),(#24043,#24044),(#24045,#24046),(#24047,#24048),
(#24049,#24050),(#24051,#24052),(#24053,#24054),(#24055,#24056),(#24057,
#24058),(#24059,#24060),(#24061,#24062),(#24063,#24064),(#24065,#24066),
(#24067,#24068),(#24069,#24070),(#24071,#24072),(#24073,#24074),(#24075,
#24076),(#24077,#24078),(#24079,#24080),(#24081,#24082),(#24083,#24084),
(#24085,#24086),(#24087,#24088),(#24089,#24090),(#24091,#24092),(#24093,
#24094),(#24095,#24096),(#24097,#24098),(#24099,#24100),(#24101,#24102),
(#24103,#24104)),.UNSPECIFIED.,.F.,.F.,.F.,(6,1,1,1,1,1,1,1,1,1,1,1,1,1,
1,1,1,1,1,1,1,1,1,1,1,1,1,1,1,1,1,1,1,1,1,1,1,1,1,1,1,1,1,1,1,1,1,1,1,1,
1,1,1,1,1,1,1,1,1,1,1,1,1,1,1,1,1,1,1,1,6),(2,2),(0.,0.0142857142857143,
0.0285714285714286,0.0428571428571429,0.0571428571428571,0.0714285714285714,
0.0857142857142857,0.1,0.114285714285714,0.128571428571429,0.142857142857143,
0.157142857142857,0.171428571428571,0.185714285714286,0.2,0.214285714285714,
0.228571428571429,0.242857142857143,0.257142857142857,0.271428571428571,
0.285714285714286,0.3,0.314285714285714,0.328571428571429,0.342857142857143,
0.357142857142857,0.371428571428571,0.385714285714286,0.4,0.414285714285714,
0.428571428571429,0.442857142857143,0.457142857142857,0.471428571428572,
0.485714285714286,0.5,0.514285714285714,0.528571428571429,0.542857142857143,
0.557142857142857,0.571428571428571,0.585714285714286,0.6,0.614285714285714,
0.628571428571428,0.642857142857142,0.657142857142857,0.671428571428571,
0.685714285714285,0.699999999999999,0.714285714285714,0.728571428571428,
0.742857142857142,0.757142857142856,0.771428571428571,0.785714285714285,
0.799999999999999,0.814285714285713,0.828571428571428,0.842857142857142,
0.857142857142856,0.87142857142857,0.885714285714284,0.899999999999999,
0.914285714285713,0.928571428571427,0.942857142857141,0.957142857142856,
0.97142857142857,0.985714285714284,1.),(0.,1.8),.UNSPECIFIED.);
#963=B_SPLINE_SURFACE_WITH_KNOTS('',5,1,((#24253,#24254),(#24255,#24256),
(#24257,#24258),(#24259,#24260),(#24261,#24262),(#24263,#24264),(#24265,
#24266),(#24267,#24268),(#24269,#24270),(#24271,#24272),(#24273,#24274),
(#24275,#24276),(#24277,#24278),(#24279,#24280),(#24281,#24282),(#24283,
#24284),(#24285,#24286),(#24287,#24288),(#24289,#24290),(#24291,#24292),
(#24293,#24294),(#24295,#24296),(#24297,#24298),(#24299,#24300),(#24301,
#24302),(#24303,#24304),(#24305,#24306),(#24307,#24308),(#24309,#24310),
(#24311,#24312),(#24313,#24314),(#24315,#24316),(#24317,#24318),(#24319,
#24320),(#24321,#24322),(#24323,#24324),(#24325,#24326),(#24327,#24328),
(#24329,#24330),(#24331,#24332),(#24333,#24334),(#24335,#24336),(#24337,
#24338),(#24339,#24340),(#24341,#24342),(#24343,#24344),(#24345,#24346),
(#24347,#24348),(#24349,#24350),(#24351,#24352),(#24353,#24354),(#24355,
#24356),(#24357,#24358),(#24359,#24360),(#24361,#24362),(#24363,#24364),
(#24365,#24366),(#24367,#24368),(#24369,#24370),(#24371,#24372),(#24373,
#24374),(#24375,#24376),(#24377,#24378),(#24379,#24380),(#24381,#24382),
(#24383,#24384),(#24385,#24386),(#24387,#24388),(#24389,#24390),(#24391,
#24392),(#24393,#24394),(#24395,#24396),(#24397,#24398),(#24399,#24400),
(#24401,#24402)),.UNSPECIFIED.,.F.,.F.,.F.,(6,1,1,1,1,1,1,1,1,1,1,1,1,1,
1,1,1,1,1,1,1,1,1,1,1,1,1,1,1,1,1,1,1,1,1,1,1,1,1,1,1,1,1,1,1,1,1,1,1,1,
1,1,1,1,1,1,1,1,1,1,1,1,1,1,1,1,1,1,1,1,6),(2,2),(-1.,-0.985714285714284,
-0.97142857142857,-0.957142857142856,-0.942857142857141,-0.928571428571427,
-0.914285714285713,-0.899999999999999,-0.885714285714284,-0.87142857142857,
-0.857142857142856,-0.842857142857142,-0.828571428571428,-0.814285714285713,
-0.799999999999999,-0.785714285714285,-0.771428571428571,-0.757142857142856,
-0.742857142857142,-0.728571428571428,-0.714285714285714,-0.699999999999999,
-0.685714285714285,-0.671428571428571,-0.657142857142857,-0.642857142857142,
-0.628571428571428,-0.614285714285714,-0.6,-0.585714285714286,-0.571428571428571,
-0.557142857142857,-0.542857142857143,-0.528571428571429,-0.514285714285714,
-0.5,-0.485714285714286,-0.471428571428572,-0.457142857142857,-0.442857142857143,
-0.428571428571429,-0.414285714285714,-0.4,-0.385714285714286,-0.371428571428571,
-0.357142857142857,-0.342857142857143,-0.328571428571429,-0.314285714285714,
-0.3,-0.285714285714286,-0.271428571428571,-0.257142857142857,-0.242857142857143,
-0.228571428571429,-0.214285714285714,-0.2,-0.185714285714286,-0.171428571428571,
-0.157142857142857,-0.142857142857143,-0.128571428571429,-0.114285714285714,
-0.1,-0.0857142857142857,-0.0714285714285714,-0.0571428571428571,-0.0428571428571429,
-0.0285714285714286,-0.0142857142857143,0.),(0.,1.8),.UNSPECIFIED.);
#964=B_SPLINE_SURFACE_WITH_KNOTS('',5,1,((#24561,#24562),(#24563,#24564),
(#24565,#24566),(#24567,#24568),(#24569,#24570),(#24571,#24572),(#24573,
#24574),(#24575,#24576),(#24577,#24578),(#24579,#24580),(#24581,#24582),
(#24583,#24584),(#24585,#24586),(#24587,#24588),(#24589,#24590),(#24591,
#24592),(#24593,#24594),(#24595,#24596),(#24597,#24598),(#24599,#24600),
(#24601,#24602),(#24603,#24604),(#24605,#24606),(#24607,#24608),(#24609,
#24610),(#24611,#24612),(#24613,#24614),(#24615,#24616),(#24617,#24618),
(#24619,#24620),(#24621,#24622),(#24623,#24624),(#24625,#24626),(#24627,
#24628),(#24629,#24630),(#24631,#24632),(#24633,#24634),(#24635,#24636),
(#24637,#24638),(#24639,#24640),(#24641,#24642),(#24643,#24644),(#24645,
#24646),(#24647,#24648),(#24649,#24650),(#24651,#24652),(#24653,#24654),
(#24655,#24656),(#24657,#24658),(#24659,#24660),(#24661,#24662),(#24663,
#24664),(#24665,#24666),(#24667,#24668),(#24669,#24670),(#24671,#24672),
(#24673,#24674),(#24675,#24676),(#24677,#24678),(#24679,#24680),(#24681,
#24682),(#24683,#24684),(#24685,#24686),(#24687,#24688),(#24689,#24690),
(#24691,#24692),(#24693,#24694),(#24695,#24696),(#24697,#24698),(#24699,
#24700),(#24701,#24702),(#24703,#24704),(#24705,#24706),(#24707,#24708),
(#24709,#24710)),.UNSPECIFIED.,.F.,.F.,.F.,(6,1,1,1,1,1,1,1,1,1,1,1,1,1,
1,1,1,1,1,1,1,1,1,1,1,1,1,1,1,1,1,1,1,1,1,1,1,1,1,1,1,1,1,1,1,1,1,1,1,1,
1,1,1,1,1,1,1,1,1,1,1,1,1,1,1,1,1,1,1,1,6),(2,2),(0.,0.0142857142857143,
0.0285714285714286,0.0428571428571429,0.0571428571428571,0.0714285714285714,
0.0857142857142857,0.1,0.114285714285714,0.128571428571429,0.142857142857143,
0.157142857142857,0.171428571428571,0.185714285714286,0.2,0.214285714285714,
0.228571428571429,0.242857142857143,0.257142857142857,0.271428571428571,
0.285714285714286,0.3,0.314285714285714,0.328571428571429,0.342857142857143,
0.357142857142857,0.371428571428571,0.385714285714286,0.4,0.414285714285714,
0.428571428571429,0.442857142857143,0.457142857142857,0.471428571428572,
0.485714285714286,0.5,0.514285714285714,0.528571428571429,0.542857142857143,
0.557142857142857,0.571428571428571,0.585714285714286,0.6,0.614285714285714,
0.628571428571428,0.642857142857142,0.657142857142857,0.671428571428571,
0.685714285714285,0.699999999999999,0.714285714285714,0.728571428571428,
0.742857142857142,0.757142857142856,0.771428571428571,0.785714285714285,
0.799999999999999,0.814285714285713,0.828571428571428,0.842857142857142,
0.857142857142856,0.87142857142857,0.885714285714284,0.899999999999999,
0.914285714285713,0.928571428571427,0.942857142857141,0.957142857142856,
0.97142857142857,0.985714285714284,1.),(0.,1.8),.UNSPECIFIED.);
#965=B_SPLINE_SURFACE_WITH_KNOTS('',5,1,((#24859,#24860),(#24861,#24862),
(#24863,#24864),(#24865,#24866),(#24867,#24868),(#24869,#24870),(#24871,
#24872),(#24873,#24874),(#24875,#24876),(#24877,#24878),(#24879,#24880),
(#24881,#24882),(#24883,#24884),(#24885,#24886),(#24887,#24888),(#24889,
#24890),(#24891,#24892),(#24893,#24894),(#24895,#24896),(#24897,#24898),
(#24899,#24900),(#24901,#24902),(#24903,#24904),(#24905,#24906),(#24907,
#24908),(#24909,#24910),(#24911,#24912),(#24913,#24914),(#24915,#24916),
(#24917,#24918),(#24919,#24920),(#24921,#24922),(#24923,#24924),(#24925,
#24926),(#24927,#24928),(#24929,#24930),(#24931,#24932),(#24933,#24934),
(#24935,#24936),(#24937,#24938),(#24939,#24940),(#24941,#24942),(#24943,
#24944),(#24945,#24946),(#24947,#24948),(#24949,#24950),(#24951,#24952),
(#24953,#24954),(#24955,#24956),(#24957,#24958),(#24959,#24960),(#24961,
#24962),(#24963,#24964),(#24965,#24966),(#24967,#24968),(#24969,#24970),
(#24971,#24972),(#24973,#24974),(#24975,#24976),(#24977,#24978),(#24979,
#24980),(#24981,#24982),(#24983,#24984),(#24985,#24986),(#24987,#24988),
(#24989,#24990),(#24991,#24992),(#24993,#24994),(#24995,#24996),(#24997,
#24998),(#24999,#25000),(#25001,#25002),(#25003,#25004),(#25005,#25006),
(#25007,#25008)),.UNSPECIFIED.,.F.,.F.,.F.,(6,1,1,1,1,1,1,1,1,1,1,1,1,1,
1,1,1,1,1,1,1,1,1,1,1,1,1,1,1,1,1,1,1,1,1,1,1,1,1,1,1,1,1,1,1,1,1,1,1,1,
1,1,1,1,1,1,1,1,1,1,1,1,1,1,1,1,1,1,1,1,6),(2,2),(-1.,-0.985714285714284,
-0.97142857142857,-0.957142857142856,-0.942857142857141,-0.928571428571427,
-0.914285714285713,-0.899999999999999,-0.885714285714284,-0.87142857142857,
-0.857142857142856,-0.842857142857142,-0.828571428571428,-0.814285714285713,
-0.799999999999999,-0.785714285714285,-0.771428571428571,-0.757142857142856,
-0.742857142857142,-0.728571428571428,-0.714285714285714,-0.699999999999999,
-0.685714285714285,-0.671428571428571,-0.657142857142857,-0.642857142857142,
-0.628571428571428,-0.614285714285714,-0.6,-0.585714285714286,-0.571428571428571,
-0.557142857142857,-0.542857142857143,-0.528571428571429,-0.514285714285714,
-0.5,-0.485714285714286,-0.471428571428572,-0.457142857142857,-0.442857142857143,
-0.428571428571429,-0.414285714285714,-0.4,-0.385714285714286,-0.371428571428571,
-0.357142857142857,-0.342857142857143,-0.328571428571429,-0.314285714285714,
-0.3,-0.285714285714286,-0.271428571428571,-0.257142857142857,-0.242857142857143,
-0.228571428571429,-0.214285714285714,-0.2,-0.185714285714286,-0.171428571428571,
-0.157142857142857,-0.142857142857143,-0.128571428571429,-0.114285714285714,
-0.1,-0.0857142857142857,-0.0714285714285714,-0.0571428571428571,-0.0428571428571429,
-0.0285714285714286,-0.0142857142857143,0.),(0.,1.8),.UNSPECIFIED.);
#966=B_SPLINE_SURFACE_WITH_KNOTS('',5,1,((#25167,#25168),(#25169,#25170),
(#25171,#25172),(#25173,#25174),(#25175,#25176),(#25177,#25178),(#25179,
#25180),(#25181,#25182),(#25183,#25184),(#25185,#25186),(#25187,#25188),
(#25189,#25190),(#25191,#25192),(#25193,#25194),(#25195,#25196),(#25197,
#25198),(#25199,#25200),(#25201,#25202),(#25203,#25204),(#25205,#25206),
(#25207,#25208),(#25209,#25210),(#25211,#25212),(#25213,#25214),(#25215,
#25216),(#25217,#25218),(#25219,#25220),(#25221,#25222),(#25223,#25224),
(#25225,#25226),(#25227,#25228),(#25229,#25230),(#25231,#25232),(#25233,
#25234),(#25235,#25236),(#25237,#25238),(#25239,#25240),(#25241,#25242),
(#25243,#25244),(#25245,#25246),(#25247,#25248),(#25249,#25250),(#25251,
#25252),(#25253,#25254),(#25255,#25256),(#25257,#25258),(#25259,#25260),
(#25261,#25262),(#25263,#25264),(#25265,#25266),(#25267,#25268),(#25269,
#25270),(#25271,#25272),(#25273,#25274),(#25275,#25276),(#25277,#25278),
(#25279,#25280),(#25281,#25282),(#25283,#25284),(#25285,#25286),(#25287,
#25288),(#25289,#25290),(#25291,#25292),(#25293,#25294),(#25295,#25296),
(#25297,#25298),(#25299,#25300),(#25301,#25302),(#25303,#25304),(#25305,
#25306),(#25307,#25308),(#25309,#25310),(#25311,#25312),(#25313,#25314),
(#25315,#25316)),.UNSPECIFIED.,.F.,.F.,.F.,(6,1,1,1,1,1,1,1,1,1,1,1,1,1,
1,1,1,1,1,1,1,1,1,1,1,1,1,1,1,1,1,1,1,1,1,1,1,1,1,1,1,1,1,1,1,1,1,1,1,1,
1,1,1,1,1,1,1,1,1,1,1,1,1,1,1,1,1,1,1,1,6),(2,2),(0.,0.0142857142857143,
0.0285714285714286,0.0428571428571429,0.0571428571428571,0.0714285714285714,
0.0857142857142857,0.1,0.114285714285714,0.128571428571429,0.142857142857143,
0.157142857142857,0.171428571428571,0.185714285714286,0.2,0.214285714285714,
0.228571428571429,0.242857142857143,0.257142857142857,0.271428571428571,
0.285714285714286,0.3,0.314285714285714,0.328571428571429,0.342857142857143,
0.357142857142857,0.371428571428571,0.385714285714286,0.4,0.414285714285714,
0.428571428571429,0.442857142857143,0.457142857142857,0.471428571428572,
0.485714285714286,0.5,0.514285714285714,0.528571428571429,0.542857142857143,
0.557142857142857,0.571428571428571,0.585714285714286,0.6,0.614285714285714,
0.628571428571428,0.642857142857142,0.657142857142857,0.671428571428571,
0.685714285714285,0.699999999999999,0.714285714285714,0.728571428571428,
0.742857142857142,0.757142857142856,0.771428571428571,0.785714285714285,
0.799999999999999,0.814285714285713,0.828571428571428,0.842857142857142,
0.857142857142856,0.87142857142857,0.885714285714284,0.899999999999999,
0.914285714285713,0.928571428571427,0.942857142857141,0.957142857142856,
0.97142857142857,0.985714285714284,1.),(0.,1.8),.UNSPECIFIED.);
#967=B_SPLINE_SURFACE_WITH_KNOTS('',5,1,((#25465,#25466),(#25467,#25468),
(#25469,#25470),(#25471,#25472),(#25473,#25474),(#25475,#25476),(#25477,
#25478),(#25479,#25480),(#25481,#25482),(#25483,#25484),(#25485,#25486),
(#25487,#25488),(#25489,#25490),(#25491,#25492),(#25493,#25494),(#25495,
#25496),(#25497,#25498),(#25499,#25500),(#25501,#25502),(#25503,#25504),
(#25505,#25506),(#25507,#25508),(#25509,#25510),(#25511,#25512),(#25513,
#25514),(#25515,#25516),(#25517,#25518),(#25519,#25520),(#25521,#25522),
(#25523,#25524),(#25525,#25526),(#25527,#25528),(#25529,#25530),(#25531,
#25532),(#25533,#25534),(#25535,#25536),(#25537,#25538),(#25539,#25540),
(#25541,#25542),(#25543,#25544),(#25545,#25546),(#25547,#25548),(#25549,
#25550),(#25551,#25552),(#25553,#25554),(#25555,#25556),(#25557,#25558),
(#25559,#25560),(#25561,#25562),(#25563,#25564),(#25565,#25566),(#25567,
#25568),(#25569,#25570),(#25571,#25572),(#25573,#25574),(#25575,#25576),
(#25577,#25578),(#25579,#25580),(#25581,#25582),(#25583,#25584),(#25585,
#25586),(#25587,#25588),(#25589,#25590),(#25591,#25592),(#25593,#25594),
(#25595,#25596),(#25597,#25598),(#25599,#25600),(#25601,#25602),(#25603,
#25604),(#25605,#25606),(#25607,#25608),(#25609,#25610),(#25611,#25612),
(#25613,#25614)),.UNSPECIFIED.,.F.,.F.,.F.,(6,1,1,1,1,1,1,1,1,1,1,1,1,1,
1,1,1,1,1,1,1,1,1,1,1,1,1,1,1,1,1,1,1,1,1,1,1,1,1,1,1,1,1,1,1,1,1,1,1,1,
1,1,1,1,1,1,1,1,1,1,1,1,1,1,1,1,1,1,1,1,6),(2,2),(-1.,-0.985714285714284,
-0.97142857142857,-0.957142857142856,-0.942857142857141,-0.928571428571427,
-0.914285714285713,-0.899999999999999,-0.885714285714284,-0.87142857142857,
-0.857142857142856,-0.842857142857142,-0.828571428571428,-0.814285714285713,
-0.799999999999999,-0.785714285714285,-0.771428571428571,-0.757142857142856,
-0.742857142857142,-0.728571428571428,-0.714285714285714,-0.699999999999999,
-0.685714285714285,-0.671428571428571,-0.657142857142857,-0.642857142857142,
-0.628571428571428,-0.614285714285714,-0.6,-0.585714285714286,-0.571428571428571,
-0.557142857142857,-0.542857142857143,-0.528571428571429,-0.514285714285714,
-0.5,-0.485714285714286,-0.471428571428572,-0.457142857142857,-0.442857142857143,
-0.428571428571429,-0.414285714285714,-0.4,-0.385714285714286,-0.371428571428571,
-0.357142857142857,-0.342857142857143,-0.328571428571429,-0.314285714285714,
-0.3,-0.285714285714286,-0.271428571428571,-0.257142857142857,-0.242857142857143,
-0.228571428571429,-0.214285714285714,-0.2,-0.185714285714286,-0.171428571428571,
-0.157142857142857,-0.142857142857143,-0.128571428571429,-0.114285714285714,
-0.1,-0.0857142857142857,-0.0714285714285714,-0.0571428571428571,-0.0428571428571429,
-0.0285714285714286,-0.0142857142857143,0.),(0.,1.8),.UNSPECIFIED.);
#968=B_SPLINE_SURFACE_WITH_KNOTS('',5,1,((#25773,#25774),(#25775,#25776),
(#25777,#25778),(#25779,#25780),(#25781,#25782),(#25783,#25784),(#25785,
#25786),(#25787,#25788),(#25789,#25790),(#25791,#25792),(#25793,#25794),
(#25795,#25796),(#25797,#25798),(#25799,#25800),(#25801,#25802),(#25803,
#25804),(#25805,#25806),(#25807,#25808),(#25809,#25810),(#25811,#25812),
(#25813,#25814),(#25815,#25816),(#25817,#25818),(#25819,#25820),(#25821,
#25822),(#25823,#25824),(#25825,#25826),(#25827,#25828),(#25829,#25830),
(#25831,#25832),(#25833,#25834),(#25835,#25836),(#25837,#25838),(#25839,
#25840),(#25841,#25842),(#25843,#25844),(#25845,#25846),(#25847,#25848),
(#25849,#25850),(#25851,#25852),(#25853,#25854),(#25855,#25856),(#25857,
#25858),(#25859,#25860),(#25861,#25862),(#25863,#25864),(#25865,#25866),
(#25867,#25868),(#25869,#25870),(#25871,#25872),(#25873,#25874),(#25875,
#25876),(#25877,#25878),(#25879,#25880),(#25881,#25882),(#25883,#25884),
(#25885,#25886),(#25887,#25888),(#25889,#25890),(#25891,#25892),(#25893,
#25894),(#25895,#25896),(#25897,#25898),(#25899,#25900),(#25901,#25902),
(#25903,#25904),(#25905,#25906),(#25907,#25908),(#25909,#25910),(#25911,
#25912),(#25913,#25914),(#25915,#25916),(#25917,#25918),(#25919,#25920),
(#25921,#25922)),.UNSPECIFIED.,.F.,.F.,.F.,(6,1,1,1,1,1,1,1,1,1,1,1,1,1,
1,1,1,1,1,1,1,1,1,1,1,1,1,1,1,1,1,1,1,1,1,1,1,1,1,1,1,1,1,1,1,1,1,1,1,1,
1,1,1,1,1,1,1,1,1,1,1,1,1,1,1,1,1,1,1,1,6),(2,2),(0.,0.0142857142857143,
0.0285714285714286,0.0428571428571429,0.0571428571428571,0.0714285714285714,
0.0857142857142857,0.1,0.114285714285714,0.128571428571429,0.142857142857143,
0.157142857142857,0.171428571428571,0.185714285714286,0.2,0.214285714285714,
0.228571428571429,0.242857142857143,0.257142857142857,0.271428571428571,
0.285714285714286,0.3,0.314285714285714,0.328571428571429,0.342857142857143,
0.357142857142857,0.371428571428571,0.385714285714286,0.4,0.414285714285714,
0.428571428571429,0.442857142857143,0.457142857142857,0.471428571428572,
0.485714285714286,0.5,0.514285714285714,0.528571428571429,0.542857142857143,
0.557142857142857,0.571428571428571,0.585714285714286,0.6,0.614285714285714,
0.628571428571428,0.642857142857142,0.657142857142857,0.671428571428571,
0.685714285714285,0.699999999999999,0.714285714285714,0.728571428571428,
0.742857142857142,0.757142857142856,0.771428571428571,0.785714285714285,
0.799999999999999,0.814285714285713,0.828571428571428,0.842857142857142,
0.857142857142856,0.87142857142857,0.885714285714284,0.899999999999999,
0.914285714285713,0.928571428571427,0.942857142857141,0.957142857142856,
0.97142857142857,0.985714285714284,1.),(0.,1.8),.UNSPECIFIED.);
#969=B_SPLINE_SURFACE_WITH_KNOTS('',5,1,((#26071,#26072),(#26073,#26074),
(#26075,#26076),(#26077,#26078),(#26079,#26080),(#26081,#26082),(#26083,
#26084),(#26085,#26086),(#26087,#26088),(#26089,#26090),(#26091,#26092),
(#26093,#26094),(#26095,#26096),(#26097,#26098),(#26099,#26100),(#26101,
#26102),(#26103,#26104),(#26105,#26106),(#26107,#26108),(#26109,#26110),
(#26111,#26112),(#26113,#26114),(#26115,#26116),(#26117,#26118),(#26119,
#26120),(#26121,#26122),(#26123,#26124),(#26125,#26126),(#26127,#26128),
(#26129,#26130),(#26131,#26132),(#26133,#26134),(#26135,#26136),(#26137,
#26138),(#26139,#26140),(#26141,#26142),(#26143,#26144),(#26145,#26146),
(#26147,#26148),(#26149,#26150),(#26151,#26152),(#26153,#26154),(#26155,
#26156),(#26157,#26158),(#26159,#26160),(#26161,#26162),(#26163,#26164),
(#26165,#26166),(#26167,#26168),(#26169,#26170),(#26171,#26172),(#26173,
#26174),(#26175,#26176),(#26177,#26178),(#26179,#26180),(#26181,#26182),
(#26183,#26184),(#26185,#26186),(#26187,#26188),(#26189,#26190),(#26191,
#26192),(#26193,#26194),(#26195,#26196),(#26197,#26198),(#26199,#26200),
(#26201,#26202),(#26203,#26204),(#26205,#26206),(#26207,#26208),(#26209,
#26210),(#26211,#26212),(#26213,#26214),(#26215,#26216),(#26217,#26218),
(#26219,#26220)),.UNSPECIFIED.,.F.,.F.,.F.,(6,1,1,1,1,1,1,1,1,1,1,1,1,1,
1,1,1,1,1,1,1,1,1,1,1,1,1,1,1,1,1,1,1,1,1,1,1,1,1,1,1,1,1,1,1,1,1,1,1,1,
1,1,1,1,1,1,1,1,1,1,1,1,1,1,1,1,1,1,1,1,6),(2,2),(-1.,-0.985714285714284,
-0.97142857142857,-0.957142857142856,-0.942857142857141,-0.928571428571427,
-0.914285714285713,-0.899999999999999,-0.885714285714284,-0.87142857142857,
-0.857142857142856,-0.842857142857142,-0.828571428571428,-0.814285714285713,
-0.799999999999999,-0.785714285714285,-0.771428571428571,-0.757142857142856,
-0.742857142857142,-0.728571428571428,-0.714285714285714,-0.699999999999999,
-0.685714285714285,-0.671428571428571,-0.657142857142857,-0.642857142857142,
-0.628571428571428,-0.614285714285714,-0.6,-0.585714285714286,-0.571428571428571,
-0.557142857142857,-0.542857142857143,-0.528571428571429,-0.514285714285714,
-0.5,-0.485714285714286,-0.471428571428572,-0.457142857142857,-0.442857142857143,
-0.428571428571429,-0.414285714285714,-0.4,-0.385714285714286,-0.371428571428571,
-0.357142857142857,-0.342857142857143,-0.328571428571429,-0.314285714285714,
-0.3,-0.285714285714286,-0.271428571428571,-0.257142857142857,-0.242857142857143,
-0.228571428571429,-0.214285714285714,-0.2,-0.185714285714286,-0.171428571428571,
-0.157142857142857,-0.142857142857143,-0.128571428571429,-0.114285714285714,
-0.1,-0.0857142857142857,-0.0714285714285714,-0.0571428571428571,-0.0428571428571429,
-0.0285714285714286,-0.0142857142857143,0.),(0.,1.8),.UNSPECIFIED.);
#970=B_SPLINE_SURFACE_WITH_KNOTS('',5,1,((#26379,#26380),(#26381,#26382),
(#26383,#26384),(#26385,#26386),(#26387,#26388),(#26389,#26390),(#26391,
#26392),(#26393,#26394),(#26395,#26396),(#26397,#26398),(#26399,#26400),
(#26401,#26402),(#26403,#26404),(#26405,#26406),(#26407,#26408),(#26409,
#26410),(#26411,#26412),(#26413,#26414),(#26415,#26416),(#26417,#26418),
(#26419,#26420),(#26421,#26422),(#26423,#26424),(#26425,#26426),(#26427,
#26428),(#26429,#26430),(#26431,#26432),(#26433,#26434),(#26435,#26436),
(#26437,#26438),(#26439,#26440),(#26441,#26442),(#26443,#26444),(#26445,
#26446),(#26447,#26448),(#26449,#26450),(#26451,#26452),(#26453,#26454),
(#26455,#26456),(#26457,#26458),(#26459,#26460),(#26461,#26462),(#26463,
#26464),(#26465,#26466),(#26467,#26468),(#26469,#26470),(#26471,#26472),
(#26473,#26474),(#26475,#26476),(#26477,#26478),(#26479,#26480),(#26481,
#26482),(#26483,#26484),(#26485,#26486),(#26487,#26488),(#26489,#26490),
(#26491,#26492),(#26493,#26494),(#26495,#26496),(#26497,#26498),(#26499,
#26500),(#26501,#26502),(#26503,#26504),(#26505,#26506),(#26507,#26508),
(#26509,#26510),(#26511,#26512),(#26513,#26514),(#26515,#26516),(#26517,
#26518),(#26519,#26520),(#26521,#26522),(#26523,#26524),(#26525,#26526),
(#26527,#26528)),.UNSPECIFIED.,.F.,.F.,.F.,(6,1,1,1,1,1,1,1,1,1,1,1,1,1,
1,1,1,1,1,1,1,1,1,1,1,1,1,1,1,1,1,1,1,1,1,1,1,1,1,1,1,1,1,1,1,1,1,1,1,1,
1,1,1,1,1,1,1,1,1,1,1,1,1,1,1,1,1,1,1,1,6),(2,2),(0.,0.0142857142857143,
0.0285714285714286,0.0428571428571429,0.0571428571428571,0.0714285714285714,
0.0857142857142857,0.1,0.114285714285714,0.128571428571429,0.142857142857143,
0.157142857142857,0.171428571428571,0.185714285714286,0.2,0.214285714285714,
0.228571428571429,0.242857142857143,0.257142857142857,0.271428571428571,
0.285714285714286,0.3,0.314285714285714,0.328571428571429,0.342857142857143,
0.357142857142857,0.371428571428571,0.385714285714286,0.4,0.414285714285714,
0.428571428571429,0.442857142857143,0.457142857142857,0.471428571428572,
0.485714285714286,0.5,0.514285714285714,0.528571428571429,0.542857142857143,
0.557142857142857,0.571428571428571,0.585714285714286,0.6,0.614285714285714,
0.628571428571428,0.642857142857142,0.657142857142857,0.671428571428571,
0.685714285714285,0.699999999999999,0.714285714285714,0.728571428571428,
0.742857142857142,0.757142857142856,0.771428571428571,0.785714285714285,
0.799999999999999,0.814285714285713,0.828571428571428,0.842857142857142,
0.857142857142856,0.87142857142857,0.885714285714284,0.899999999999999,
0.914285714285713,0.928571428571427,0.942857142857141,0.957142857142856,
0.97142857142857,0.985714285714284,1.),(0.,1.8),.UNSPECIFIED.);
#971=B_SPLINE_SURFACE_WITH_KNOTS('',5,1,((#26677,#26678),(#26679,#26680),
(#26681,#26682),(#26683,#26684),(#26685,#26686),(#26687,#26688),(#26689,
#26690),(#26691,#26692),(#26693,#26694),(#26695,#26696),(#26697,#26698),
(#26699,#26700),(#26701,#26702),(#26703,#26704),(#26705,#26706),(#26707,
#26708),(#26709,#26710),(#26711,#26712),(#26713,#26714),(#26715,#26716),
(#26717,#26718),(#26719,#26720),(#26721,#26722),(#26723,#26724),(#26725,
#26726),(#26727,#26728),(#26729,#26730),(#26731,#26732),(#26733,#26734),
(#26735,#26736),(#26737,#26738),(#26739,#26740),(#26741,#26742),(#26743,
#26744),(#26745,#26746),(#26747,#26748),(#26749,#26750),(#26751,#26752),
(#26753,#26754),(#26755,#26756),(#26757,#26758),(#26759,#26760),(#26761,
#26762),(#26763,#26764),(#26765,#26766),(#26767,#26768),(#26769,#26770),
(#26771,#26772),(#26773,#26774),(#26775,#26776),(#26777,#26778),(#26779,
#26780),(#26781,#26782),(#26783,#26784),(#26785,#26786),(#26787,#26788),
(#26789,#26790),(#26791,#26792),(#26793,#26794),(#26795,#26796),(#26797,
#26798),(#26799,#26800),(#26801,#26802),(#26803,#26804),(#26805,#26806),
(#26807,#26808),(#26809,#26810),(#26811,#26812),(#26813,#26814),(#26815,
#26816),(#26817,#26818),(#26819,#26820),(#26821,#26822),(#26823,#26824),
(#26825,#26826)),.UNSPECIFIED.,.F.,.F.,.F.,(6,1,1,1,1,1,1,1,1,1,1,1,1,1,
1,1,1,1,1,1,1,1,1,1,1,1,1,1,1,1,1,1,1,1,1,1,1,1,1,1,1,1,1,1,1,1,1,1,1,1,
1,1,1,1,1,1,1,1,1,1,1,1,1,1,1,1,1,1,1,1,6),(2,2),(-1.,-0.985714285714284,
-0.97142857142857,-0.957142857142856,-0.942857142857141,-0.928571428571427,
-0.914285714285713,-0.899999999999999,-0.885714285714284,-0.87142857142857,
-0.857142857142856,-0.842857142857142,-0.828571428571428,-0.814285714285713,
-0.799999999999999,-0.785714285714285,-0.771428571428571,-0.757142857142856,
-0.742857142857142,-0.728571428571428,-0.714285714285714,-0.699999999999999,
-0.685714285714285,-0.671428571428571,-0.657142857142857,-0.642857142857142,
-0.628571428571428,-0.614285714285714,-0.6,-0.585714285714286,-0.571428571428571,
-0.557142857142857,-0.542857142857143,-0.528571428571429,-0.514285714285714,
-0.5,-0.485714285714286,-0.471428571428572,-0.457142857142857,-0.442857142857143,
-0.428571428571429,-0.414285714285714,-0.4,-0.385714285714286,-0.371428571428571,
-0.357142857142857,-0.342857142857143,-0.328571428571429,-0.314285714285714,
-0.3,-0.285714285714286,-0.271428571428571,-0.257142857142857,-0.242857142857143,
-0.228571428571429,-0.214285714285714,-0.2,-0.185714285714286,-0.171428571428571,
-0.157142857142857,-0.142857142857143,-0.128571428571429,-0.114285714285714,
-0.1,-0.0857142857142857,-0.0714285714285714,-0.0571428571428571,-0.0428571428571429,
-0.0285714285714286,-0.0142857142857143,0.),(0.,1.8),.UNSPECIFIED.);
#972=B_SPLINE_SURFACE_WITH_KNOTS('',5,1,((#26985,#26986),(#26987,#26988),
(#26989,#26990),(#26991,#26992),(#26993,#26994),(#26995,#26996),(#26997,
#26998),(#26999,#27000),(#27001,#27002),(#27003,#27004),(#27005,#27006),
(#27007,#27008),(#27009,#27010),(#27011,#27012),(#27013,#27014),(#27015,
#27016),(#27017,#27018),(#27019,#27020),(#27021,#27022),(#27023,#27024),
(#27025,#27026),(#27027,#27028),(#27029,#27030),(#27031,#27032),(#27033,
#27034),(#27035,#27036),(#27037,#27038),(#27039,#27040),(#27041,#27042),
(#27043,#27044),(#27045,#27046),(#27047,#27048),(#27049,#27050),(#27051,
#27052),(#27053,#27054),(#27055,#27056),(#27057,#27058),(#27059,#27060),
(#27061,#27062),(#27063,#27064),(#27065,#27066),(#27067,#27068),(#27069,
#27070),(#27071,#27072),(#27073,#27074),(#27075,#27076),(#27077,#27078),
(#27079,#27080),(#27081,#27082),(#27083,#27084),(#27085,#27086),(#27087,
#27088),(#27089,#27090),(#27091,#27092),(#27093,#27094),(#27095,#27096),
(#27097,#27098),(#27099,#27100),(#27101,#27102),(#27103,#27104),(#27105,
#27106),(#27107,#27108),(#27109,#27110),(#27111,#27112),(#27113,#27114),
(#27115,#27116),(#27117,#27118),(#27119,#27120),(#27121,#27122),(#27123,
#27124),(#27125,#27126),(#27127,#27128),(#27129,#27130),(#27131,#27132),
(#27133,#27134)),.UNSPECIFIED.,.F.,.F.,.F.,(6,1,1,1,1,1,1,1,1,1,1,1,1,1,
1,1,1,1,1,1,1,1,1,1,1,1,1,1,1,1,1,1,1,1,1,1,1,1,1,1,1,1,1,1,1,1,1,1,1,1,
1,1,1,1,1,1,1,1,1,1,1,1,1,1,1,1,1,1,1,1,6),(2,2),(0.,0.0142857142857143,
0.0285714285714286,0.0428571428571429,0.0571428571428571,0.0714285714285714,
0.0857142857142857,0.1,0.114285714285714,0.128571428571429,0.142857142857143,
0.157142857142857,0.171428571428571,0.185714285714286,0.2,0.214285714285714,
0.228571428571429,0.242857142857143,0.257142857142857,0.271428571428571,
0.285714285714286,0.3,0.314285714285714,0.328571428571429,0.342857142857143,
0.357142857142857,0.371428571428571,0.385714285714286,0.4,0.414285714285714,
0.428571428571429,0.442857142857143,0.457142857142857,0.471428571428572,
0.485714285714286,0.5,0.514285714285714,0.528571428571429,0.542857142857143,
0.557142857142857,0.571428571428571,0.585714285714286,0.6,0.614285714285714,
0.628571428571428,0.642857142857142,0.657142857142857,0.671428571428571,
0.685714285714285,0.699999999999999,0.714285714285714,0.728571428571428,
0.742857142857142,0.757142857142856,0.771428571428571,0.785714285714285,
0.799999999999999,0.814285714285713,0.828571428571428,0.842857142857142,
0.857142857142856,0.87142857142857,0.885714285714284,0.899999999999999,
0.914285714285713,0.928571428571427,0.942857142857141,0.957142857142856,
0.97142857142857,0.985714285714284,1.),(0.,1.8),.UNSPECIFIED.);
#973=B_SPLINE_SURFACE_WITH_KNOTS('',5,1,((#27283,#27284),(#27285,#27286),
(#27287,#27288),(#27289,#27290),(#27291,#27292),(#27293,#27294),(#27295,
#27296),(#27297,#27298),(#27299,#27300),(#27301,#27302),(#27303,#27304),
(#27305,#27306),(#27307,#27308),(#27309,#27310),(#27311,#27312),(#27313,
#27314),(#27315,#27316),(#27317,#27318),(#27319,#27320),(#27321,#27322),
(#27323,#27324),(#27325,#27326),(#27327,#27328),(#27329,#27330),(#27331,
#27332),(#27333,#27334),(#27335,#27336),(#27337,#27338),(#27339,#27340),
(#27341,#27342),(#27343,#27344),(#27345,#27346),(#27347,#27348),(#27349,
#27350),(#27351,#27352),(#27353,#27354),(#27355,#27356),(#27357,#27358),
(#27359,#27360),(#27361,#27362),(#27363,#27364),(#27365,#27366),(#27367,
#27368),(#27369,#27370),(#27371,#27372),(#27373,#27374),(#27375,#27376),
(#27377,#27378),(#27379,#27380),(#27381,#27382),(#27383,#27384),(#27385,
#27386),(#27387,#27388),(#27389,#27390),(#27391,#27392),(#27393,#27394),
(#27395,#27396),(#27397,#27398),(#27399,#27400),(#27401,#27402),(#27403,
#27404),(#27405,#27406),(#27407,#27408),(#27409,#27410),(#27411,#27412),
(#27413,#27414),(#27415,#27416),(#27417,#27418),(#27419,#27420),(#27421,
#27422),(#27423,#27424),(#27425,#27426),(#27427,#27428),(#27429,#27430),
(#27431,#27432)),.UNSPECIFIED.,.F.,.F.,.F.,(6,1,1,1,1,1,1,1,1,1,1,1,1,1,
1,1,1,1,1,1,1,1,1,1,1,1,1,1,1,1,1,1,1,1,1,1,1,1,1,1,1,1,1,1,1,1,1,1,1,1,
1,1,1,1,1,1,1,1,1,1,1,1,1,1,1,1,1,1,1,1,6),(2,2),(-1.,-0.985714285714284,
-0.97142857142857,-0.957142857142856,-0.942857142857141,-0.928571428571427,
-0.914285714285713,-0.899999999999999,-0.885714285714284,-0.87142857142857,
-0.857142857142856,-0.842857142857142,-0.828571428571428,-0.814285714285713,
-0.799999999999999,-0.785714285714285,-0.771428571428571,-0.757142857142856,
-0.742857142857142,-0.728571428571428,-0.714285714285714,-0.699999999999999,
-0.685714285714285,-0.671428571428571,-0.657142857142857,-0.642857142857142,
-0.628571428571428,-0.614285714285714,-0.6,-0.585714285714286,-0.571428571428571,
-0.557142857142857,-0.542857142857143,-0.528571428571429,-0.514285714285714,
-0.5,-0.485714285714286,-0.471428571428572,-0.457142857142857,-0.442857142857143,
-0.428571428571429,-0.414285714285714,-0.4,-0.385714285714286,-0.371428571428571,
-0.357142857142857,-0.342857142857143,-0.328571428571429,-0.314285714285714,
-0.3,-0.285714285714286,-0.271428571428571,-0.257142857142857,-0.242857142857143,
-0.228571428571429,-0.214285714285714,-0.2,-0.185714285714286,-0.171428571428571,
-0.157142857142857,-0.142857142857143,-0.128571428571429,-0.114285714285714,
-0.1,-0.0857142857142857,-0.0714285714285714,-0.0571428571428571,-0.0428571428571429,
-0.0285714285714286,-0.0142857142857143,0.),(0.,1.8),.UNSPECIFIED.);
#974=B_SPLINE_SURFACE_WITH_KNOTS('',5,1,((#27591,#27592),(#27593,#27594),
(#27595,#27596),(#27597,#27598),(#27599,#27600),(#27601,#27602),(#27603,
#27604),(#27605,#27606),(#27607,#27608),(#27609,#27610),(#27611,#27612),
(#27613,#27614),(#27615,#27616),(#27617,#27618),(#27619,#27620),(#27621,
#27622),(#27623,#27624),(#27625,#27626),(#27627,#27628),(#27629,#27630),
(#27631,#27632),(#27633,#27634),(#27635,#27636),(#27637,#27638),(#27639,
#27640),(#27641,#27642),(#27643,#27644),(#27645,#27646),(#27647,#27648),
(#27649,#27650),(#27651,#27652),(#27653,#27654),(#27655,#27656),(#27657,
#27658),(#27659,#27660),(#27661,#27662),(#27663,#27664),(#27665,#27666),
(#27667,#27668),(#27669,#27670),(#27671,#27672),(#27673,#27674),(#27675,
#27676),(#27677,#27678),(#27679,#27680),(#27681,#27682),(#27683,#27684),
(#27685,#27686),(#27687,#27688),(#27689,#27690),(#27691,#27692),(#27693,
#27694),(#27695,#27696),(#27697,#27698),(#27699,#27700),(#27701,#27702),
(#27703,#27704),(#27705,#27706),(#27707,#27708),(#27709,#27710),(#27711,
#27712),(#27713,#27714),(#27715,#27716),(#27717,#27718),(#27719,#27720),
(#27721,#27722),(#27723,#27724),(#27725,#27726),(#27727,#27728),(#27729,
#27730),(#27731,#27732),(#27733,#27734),(#27735,#27736),(#27737,#27738),
(#27739,#27740)),.UNSPECIFIED.,.F.,.F.,.F.,(6,1,1,1,1,1,1,1,1,1,1,1,1,1,
1,1,1,1,1,1,1,1,1,1,1,1,1,1,1,1,1,1,1,1,1,1,1,1,1,1,1,1,1,1,1,1,1,1,1,1,
1,1,1,1,1,1,1,1,1,1,1,1,1,1,1,1,1,1,1,1,6),(2,2),(0.,0.0142857142857143,
0.0285714285714286,0.0428571428571429,0.0571428571428571,0.0714285714285714,
0.0857142857142857,0.1,0.114285714285714,0.128571428571429,0.142857142857143,
0.157142857142857,0.171428571428571,0.185714285714286,0.2,0.214285714285714,
0.228571428571429,0.242857142857143,0.257142857142857,0.271428571428571,
0.285714285714286,0.3,0.314285714285714,0.328571428571429,0.342857142857143,
0.357142857142857,0.371428571428571,0.385714285714286,0.4,0.414285714285714,
0.428571428571429,0.442857142857143,0.457142857142857,0.471428571428572,
0.485714285714286,0.5,0.514285714285714,0.528571428571429,0.542857142857143,
0.557142857142857,0.571428571428571,0.585714285714286,0.6,0.614285714285714,
0.628571428571428,0.642857142857142,0.657142857142857,0.671428571428571,
0.685714285714285,0.699999999999999,0.714285714285714,0.728571428571428,
0.742857142857142,0.757142857142856,0.771428571428571,0.785714285714285,
0.799999999999999,0.814285714285713,0.828571428571428,0.842857142857142,
0.857142857142856,0.87142857142857,0.885714285714284,0.899999999999999,
0.914285714285713,0.928571428571427,0.942857142857141,0.957142857142856,
0.97142857142857,0.985714285714284,1.),(0.,1.8),.UNSPECIFIED.);
#975=B_SPLINE_SURFACE_WITH_KNOTS('',5,1,((#27889,#27890),(#27891,#27892),
(#27893,#27894),(#27895,#27896),(#27897,#27898),(#27899,#27900),(#27901,
#27902),(#27903,#27904),(#27905,#27906),(#27907,#27908),(#27909,#27910),
(#27911,#27912),(#27913,#27914),(#27915,#27916),(#27917,#27918),(#27919,
#27920),(#27921,#27922),(#27923,#27924),(#27925,#27926),(#27927,#27928),
(#27929,#27930),(#27931,#27932),(#27933,#27934),(#27935,#27936),(#27937,
#27938),(#27939,#27940),(#27941,#27942),(#27943,#27944),(#27945,#27946),
(#27947,#27948),(#27949,#27950),(#27951,#27952),(#27953,#27954),(#27955,
#27956),(#27957,#27958),(#27959,#27960),(#27961,#27962),(#27963,#27964),
(#27965,#27966),(#27967,#27968),(#27969,#27970),(#27971,#27972),(#27973,
#27974),(#27975,#27976),(#27977,#27978),(#27979,#27980),(#27981,#27982),
(#27983,#27984),(#27985,#27986),(#27987,#27988),(#27989,#27990),(#27991,
#27992),(#27993,#27994),(#27995,#27996),(#27997,#27998),(#27999,#28000),
(#28001,#28002),(#28003,#28004),(#28005,#28006),(#28007,#28008),(#28009,
#28010),(#28011,#28012),(#28013,#28014),(#28015,#28016),(#28017,#28018),
(#28019,#28020),(#28021,#28022),(#28023,#28024),(#28025,#28026),(#28027,
#28028),(#28029,#28030),(#28031,#28032),(#28033,#28034),(#28035,#28036),
(#28037,#28038)),.UNSPECIFIED.,.F.,.F.,.F.,(6,1,1,1,1,1,1,1,1,1,1,1,1,1,
1,1,1,1,1,1,1,1,1,1,1,1,1,1,1,1,1,1,1,1,1,1,1,1,1,1,1,1,1,1,1,1,1,1,1,1,
1,1,1,1,1,1,1,1,1,1,1,1,1,1,1,1,1,1,1,1,6),(2,2),(-1.,-0.985714285714284,
-0.97142857142857,-0.957142857142856,-0.942857142857141,-0.928571428571427,
-0.914285714285713,-0.899999999999999,-0.885714285714284,-0.87142857142857,
-0.857142857142856,-0.842857142857142,-0.828571428571428,-0.814285714285713,
-0.799999999999999,-0.785714285714285,-0.771428571428571,-0.757142857142856,
-0.742857142857142,-0.728571428571428,-0.714285714285714,-0.699999999999999,
-0.685714285714285,-0.671428571428571,-0.657142857142857,-0.642857142857142,
-0.628571428571428,-0.614285714285714,-0.6,-0.585714285714286,-0.571428571428571,
-0.557142857142857,-0.542857142857143,-0.528571428571429,-0.514285714285714,
-0.5,-0.485714285714286,-0.471428571428572,-0.457142857142857,-0.442857142857143,
-0.428571428571429,-0.414285714285714,-0.4,-0.385714285714286,-0.371428571428571,
-0.357142857142857,-0.342857142857143,-0.328571428571429,-0.314285714285714,
-0.3,-0.285714285714286,-0.271428571428571,-0.257142857142857,-0.242857142857143,
-0.228571428571429,-0.214285714285714,-0.2,-0.185714285714286,-0.171428571428571,
-0.157142857142857,-0.142857142857143,-0.128571428571429,-0.114285714285714,
-0.1,-0.0857142857142857,-0.0714285714285714,-0.0571428571428571,-0.0428571428571429,
-0.0285714285714286,-0.0142857142857143,0.),(0.,1.8),.UNSPECIFIED.);
#976=B_SPLINE_SURFACE_WITH_KNOTS('',5,1,((#28197,#28198),(#28199,#28200),
(#28201,#28202),(#28203,#28204),(#28205,#28206),(#28207,#28208),(#28209,
#28210),(#28211,#28212),(#28213,#28214),(#28215,#28216),(#28217,#28218),
(#28219,#28220),(#28221,#28222),(#28223,#28224),(#28225,#28226),(#28227,
#28228),(#28229,#28230),(#28231,#28232),(#28233,#28234),(#28235,#28236),
(#28237,#28238),(#28239,#28240),(#28241,#28242),(#28243,#28244),(#28245,
#28246),(#28247,#28248),(#28249,#28250),(#28251,#28252),(#28253,#28254),
(#28255,#28256),(#28257,#28258),(#28259,#28260),(#28261,#28262),(#28263,
#28264),(#28265,#28266),(#28267,#28268),(#28269,#28270),(#28271,#28272),
(#28273,#28274),(#28275,#28276),(#28277,#28278),(#28279,#28280),(#28281,
#28282),(#28283,#28284),(#28285,#28286),(#28287,#28288),(#28289,#28290),
(#28291,#28292),(#28293,#28294),(#28295,#28296),(#28297,#28298),(#28299,
#28300),(#28301,#28302),(#28303,#28304),(#28305,#28306),(#28307,#28308),
(#28309,#28310),(#28311,#28312),(#28313,#28314),(#28315,#28316),(#28317,
#28318),(#28319,#28320),(#28321,#28322),(#28323,#28324),(#28325,#28326),
(#28327,#28328),(#28329,#28330),(#28331,#28332),(#28333,#28334),(#28335,
#28336),(#28337,#28338),(#28339,#28340),(#28341,#28342),(#28343,#28344),
(#28345,#28346)),.UNSPECIFIED.,.F.,.F.,.F.,(6,1,1,1,1,1,1,1,1,1,1,1,1,1,
1,1,1,1,1,1,1,1,1,1,1,1,1,1,1,1,1,1,1,1,1,1,1,1,1,1,1,1,1,1,1,1,1,1,1,1,
1,1,1,1,1,1,1,1,1,1,1,1,1,1,1,1,1,1,1,1,6),(2,2),(0.,0.0142857142857143,
0.0285714285714286,0.0428571428571429,0.0571428571428571,0.0714285714285714,
0.0857142857142857,0.1,0.114285714285714,0.128571428571429,0.142857142857143,
0.157142857142857,0.171428571428571,0.185714285714286,0.2,0.214285714285714,
0.228571428571429,0.242857142857143,0.257142857142857,0.271428571428571,
0.285714285714286,0.3,0.314285714285714,0.328571428571429,0.342857142857143,
0.357142857142857,0.371428571428571,0.385714285714286,0.4,0.414285714285714,
0.428571428571429,0.442857142857143,0.457142857142857,0.471428571428572,
0.485714285714286,0.5,0.514285714285714,0.528571428571429,0.542857142857143,
0.557142857142857,0.571428571428571,0.585714285714286,0.6,0.614285714285714,
0.628571428571428,0.642857142857142,0.657142857142857,0.671428571428571,
0.685714285714285,0.699999999999999,0.714285714285714,0.728571428571428,
0.742857142857142,0.757142857142856,0.771428571428571,0.785714285714285,
0.799999999999999,0.814285714285713,0.828571428571428,0.842857142857142,
0.857142857142856,0.87142857142857,0.885714285714284,0.899999999999999,
0.914285714285713,0.928571428571427,0.942857142857141,0.957142857142856,
0.97142857142857,0.985714285714284,1.),(0.,1.8),.UNSPECIFIED.);
#977=B_SPLINE_SURFACE_WITH_KNOTS('',5,1,((#28495,#28496),(#28497,#28498),
(#28499,#28500),(#28501,#28502),(#28503,#28504),(#28505,#28506),(#28507,
#28508),(#28509,#28510),(#28511,#28512),(#28513,#28514),(#28515,#28516),
(#28517,#28518),(#28519,#28520),(#28521,#28522),(#28523,#28524),(#28525,
#28526),(#28527,#28528),(#28529,#28530),(#28531,#28532),(#28533,#28534),
(#28535,#28536),(#28537,#28538),(#28539,#28540),(#28541,#28542),(#28543,
#28544),(#28545,#28546),(#28547,#28548),(#28549,#28550),(#28551,#28552),
(#28553,#28554),(#28555,#28556),(#28557,#28558),(#28559,#28560),(#28561,
#28562),(#28563,#28564),(#28565,#28566),(#28567,#28568),(#28569,#28570),
(#28571,#28572),(#28573,#28574),(#28575,#28576),(#28577,#28578),(#28579,
#28580),(#28581,#28582),(#28583,#28584),(#28585,#28586),(#28587,#28588),
(#28589,#28590),(#28591,#28592),(#28593,#28594),(#28595,#28596),(#28597,
#28598),(#28599,#28600),(#28601,#28602),(#28603,#28604),(#28605,#28606),
(#28607,#28608),(#28609,#28610),(#28611,#28612),(#28613,#28614),(#28615,
#28616),(#28617,#28618),(#28619,#28620),(#28621,#28622),(#28623,#28624),
(#28625,#28626),(#28627,#28628),(#28629,#28630),(#28631,#28632),(#28633,
#28634),(#28635,#28636),(#28637,#28638),(#28639,#28640),(#28641,#28642),
(#28643,#28644)),.UNSPECIFIED.,.F.,.F.,.F.,(6,1,1,1,1,1,1,1,1,1,1,1,1,1,
1,1,1,1,1,1,1,1,1,1,1,1,1,1,1,1,1,1,1,1,1,1,1,1,1,1,1,1,1,1,1,1,1,1,1,1,
1,1,1,1,1,1,1,1,1,1,1,1,1,1,1,1,1,1,1,1,6),(2,2),(-1.,-0.985714285714284,
-0.97142857142857,-0.957142857142856,-0.942857142857141,-0.928571428571427,
-0.914285714285713,-0.899999999999999,-0.885714285714284,-0.87142857142857,
-0.857142857142856,-0.842857142857142,-0.828571428571428,-0.814285714285713,
-0.799999999999999,-0.785714285714285,-0.771428571428571,-0.757142857142856,
-0.742857142857142,-0.728571428571428,-0.714285714285714,-0.699999999999999,
-0.685714285714285,-0.671428571428571,-0.657142857142857,-0.642857142857142,
-0.628571428571428,-0.614285714285714,-0.6,-0.585714285714286,-0.571428571428571,
-0.557142857142857,-0.542857142857143,-0.528571428571429,-0.514285714285714,
-0.5,-0.485714285714286,-0.471428571428572,-0.457142857142857,-0.442857142857143,
-0.428571428571429,-0.414285714285714,-0.4,-0.385714285714286,-0.371428571428571,
-0.357142857142857,-0.342857142857143,-0.328571428571429,-0.314285714285714,
-0.3,-0.285714285714286,-0.271428571428571,-0.257142857142857,-0.242857142857143,
-0.228571428571429,-0.214285714285714,-0.2,-0.185714285714286,-0.171428571428571,
-0.157142857142857,-0.142857142857143,-0.128571428571429,-0.114285714285714,
-0.1,-0.0857142857142857,-0.0714285714285714,-0.0571428571428571,-0.0428571428571429,
-0.0285714285714286,-0.0142857142857143,0.),(0.,1.8),.UNSPECIFIED.);
#978=B_SPLINE_SURFACE_WITH_KNOTS('',5,1,((#28803,#28804),(#28805,#28806),
(#28807,#28808),(#28809,#28810),(#28811,#28812),(#28813,#28814),(#28815,
#28816),(#28817,#28818),(#28819,#28820),(#28821,#28822),(#28823,#28824),
(#28825,#28826),(#28827,#28828),(#28829,#28830),(#28831,#28832),(#28833,
#28834),(#28835,#28836),(#28837,#28838),(#28839,#28840),(#28841,#28842),
(#28843,#28844),(#28845,#28846),(#28847,#28848),(#28849,#28850),(#28851,
#28852),(#28853,#28854),(#28855,#28856),(#28857,#28858),(#28859,#28860),
(#28861,#28862),(#28863,#28864),(#28865,#28866),(#28867,#28868),(#28869,
#28870),(#28871,#28872),(#28873,#28874),(#28875,#28876),(#28877,#28878),
(#28879,#28880),(#28881,#28882),(#28883,#28884),(#28885,#28886),(#28887,
#28888),(#28889,#28890),(#28891,#28892),(#28893,#28894),(#28895,#28896),
(#28897,#28898),(#28899,#28900),(#28901,#28902),(#28903,#28904),(#28905,
#28906),(#28907,#28908),(#28909,#28910),(#28911,#28912),(#28913,#28914),
(#28915,#28916),(#28917,#28918),(#28919,#28920),(#28921,#28922),(#28923,
#28924),(#28925,#28926),(#28927,#28928),(#28929,#28930),(#28931,#28932),
(#28933,#28934),(#28935,#28936),(#28937,#28938),(#28939,#28940),(#28941,
#28942),(#28943,#28944),(#28945,#28946),(#28947,#28948),(#28949,#28950),
(#28951,#28952)),.UNSPECIFIED.,.F.,.F.,.F.,(6,1,1,1,1,1,1,1,1,1,1,1,1,1,
1,1,1,1,1,1,1,1,1,1,1,1,1,1,1,1,1,1,1,1,1,1,1,1,1,1,1,1,1,1,1,1,1,1,1,1,
1,1,1,1,1,1,1,1,1,1,1,1,1,1,1,1,1,1,1,1,6),(2,2),(0.,0.0142857142857143,
0.0285714285714286,0.0428571428571429,0.0571428571428571,0.0714285714285714,
0.0857142857142857,0.1,0.114285714285714,0.128571428571429,0.142857142857143,
0.157142857142857,0.171428571428571,0.185714285714286,0.2,0.214285714285714,
0.228571428571429,0.242857142857143,0.257142857142857,0.271428571428571,
0.285714285714286,0.3,0.314285714285714,0.328571428571429,0.342857142857143,
0.357142857142857,0.371428571428571,0.385714285714286,0.4,0.414285714285714,
0.428571428571429,0.442857142857143,0.457142857142857,0.471428571428572,
0.485714285714286,0.5,0.514285714285714,0.528571428571429,0.542857142857143,
0.557142857142857,0.571428571428571,0.585714285714286,0.6,0.614285714285714,
0.628571428571428,0.642857142857142,0.657142857142857,0.671428571428571,
0.685714285714285,0.699999999999999,0.714285714285714,0.728571428571428,
0.742857142857142,0.757142857142856,0.771428571428571,0.785714285714285,
0.799999999999999,0.814285714285713,0.828571428571428,0.842857142857142,
0.857142857142856,0.87142857142857,0.885714285714284,0.899999999999999,
0.914285714285713,0.928571428571427,0.942857142857141,0.957142857142856,
0.97142857142857,0.985714285714284,1.),(0.,1.8),.UNSPECIFIED.);
#979=B_SPLINE_SURFACE_WITH_KNOTS('',5,1,((#29101,#29102),(#29103,#29104),
(#29105,#29106),(#29107,#29108),(#29109,#29110),(#29111,#29112),(#29113,
#29114),(#29115,#29116),(#29117,#29118),(#29119,#29120),(#29121,#29122),
(#29123,#29124),(#29125,#29126),(#29127,#29128),(#29129,#29130),(#29131,
#29132),(#29133,#29134),(#29135,#29136),(#29137,#29138),(#29139,#29140),
(#29141,#29142),(#29143,#29144),(#29145,#29146),(#29147,#29148),(#29149,
#29150),(#29151,#29152),(#29153,#29154),(#29155,#29156),(#29157,#29158),
(#29159,#29160),(#29161,#29162),(#29163,#29164),(#29165,#29166),(#29167,
#29168),(#29169,#29170),(#29171,#29172),(#29173,#29174),(#29175,#29176),
(#29177,#29178),(#29179,#29180),(#29181,#29182),(#29183,#29184),(#29185,
#29186),(#29187,#29188),(#29189,#29190),(#29191,#29192),(#29193,#29194),
(#29195,#29196),(#29197,#29198),(#29199,#29200),(#29201,#29202),(#29203,
#29204),(#29205,#29206),(#29207,#29208),(#29209,#29210),(#29211,#29212),
(#29213,#29214),(#29215,#29216),(#29217,#29218),(#29219,#29220),(#29221,
#29222),(#29223,#29224),(#29225,#29226),(#29227,#29228),(#29229,#29230),
(#29231,#29232),(#29233,#29234),(#29235,#29236),(#29237,#29238),(#29239,
#29240),(#29241,#29242),(#29243,#29244),(#29245,#29246),(#29247,#29248),
(#29249,#29250)),.UNSPECIFIED.,.F.,.F.,.F.,(6,1,1,1,1,1,1,1,1,1,1,1,1,1,
1,1,1,1,1,1,1,1,1,1,1,1,1,1,1,1,1,1,1,1,1,1,1,1,1,1,1,1,1,1,1,1,1,1,1,1,
1,1,1,1,1,1,1,1,1,1,1,1,1,1,1,1,1,1,1,1,6),(2,2),(-1.,-0.985714285714284,
-0.97142857142857,-0.957142857142856,-0.942857142857141,-0.928571428571427,
-0.914285714285713,-0.899999999999999,-0.885714285714284,-0.87142857142857,
-0.857142857142856,-0.842857142857142,-0.828571428571428,-0.814285714285713,
-0.799999999999999,-0.785714285714285,-0.771428571428571,-0.757142857142856,
-0.742857142857142,-0.728571428571428,-0.714285714285714,-0.699999999999999,
-0.685714285714285,-0.671428571428571,-0.657142857142857,-0.642857142857142,
-0.628571428571428,-0.614285714285714,-0.6,-0.585714285714286,-0.571428571428571,
-0.557142857142857,-0.542857142857143,-0.528571428571429,-0.514285714285714,
-0.5,-0.485714285714286,-0.471428571428572,-0.457142857142857,-0.442857142857143,
-0.428571428571429,-0.414285714285714,-0.4,-0.385714285714286,-0.371428571428571,
-0.357142857142857,-0.342857142857143,-0.328571428571429,-0.314285714285714,
-0.3,-0.285714285714286,-0.271428571428571,-0.257142857142857,-0.242857142857143,
-0.228571428571429,-0.214285714285714,-0.2,-0.185714285714286,-0.171428571428571,
-0.157142857142857,-0.142857142857143,-0.128571428571429,-0.114285714285714,
-0.1,-0.0857142857142857,-0.0714285714285714,-0.0571428571428571,-0.0428571428571429,
-0.0285714285714286,-0.0142857142857143,0.),(0.,1.8),.UNSPECIFIED.);
#980=B_SPLINE_SURFACE_WITH_KNOTS('',5,1,((#29409,#29410),(#29411,#29412),
(#29413,#29414),(#29415,#29416),(#29417,#29418),(#29419,#29420),(#29421,
#29422),(#29423,#29424),(#29425,#29426),(#29427,#29428),(#29429,#29430),
(#29431,#29432),(#29433,#29434),(#29435,#29436),(#29437,#29438),(#29439,
#29440),(#29441,#29442),(#29443,#29444),(#29445,#29446),(#29447,#29448),
(#29449,#29450),(#29451,#29452),(#29453,#29454),(#29455,#29456),(#29457,
#29458),(#29459,#29460),(#29461,#29462),(#29463,#29464),(#29465,#29466),
(#29467,#29468),(#29469,#29470),(#29471,#29472),(#29473,#29474),(#29475,
#29476),(#29477,#29478),(#29479,#29480),(#29481,#29482),(#29483,#29484),
(#29485,#29486),(#29487,#29488),(#29489,#29490),(#29491,#29492),(#29493,
#29494),(#29495,#29496),(#29497,#29498),(#29499,#29500),(#29501,#29502),
(#29503,#29504),(#29505,#29506),(#29507,#29508),(#29509,#29510),(#29511,
#29512),(#29513,#29514),(#29515,#29516),(#29517,#29518),(#29519,#29520),
(#29521,#29522),(#29523,#29524),(#29525,#29526),(#29527,#29528),(#29529,
#29530),(#29531,#29532),(#29533,#29534),(#29535,#29536),(#29537,#29538),
(#29539,#29540),(#29541,#29542),(#29543,#29544),(#29545,#29546),(#29547,
#29548),(#29549,#29550),(#29551,#29552),(#29553,#29554),(#29555,#29556),
(#29557,#29558)),.UNSPECIFIED.,.F.,.F.,.F.,(6,1,1,1,1,1,1,1,1,1,1,1,1,1,
1,1,1,1,1,1,1,1,1,1,1,1,1,1,1,1,1,1,1,1,1,1,1,1,1,1,1,1,1,1,1,1,1,1,1,1,
1,1,1,1,1,1,1,1,1,1,1,1,1,1,1,1,1,1,1,1,6),(2,2),(0.,0.0142857142857143,
0.0285714285714286,0.0428571428571429,0.0571428571428571,0.0714285714285714,
0.0857142857142857,0.1,0.114285714285714,0.128571428571429,0.142857142857143,
0.157142857142857,0.171428571428571,0.185714285714286,0.2,0.214285714285714,
0.228571428571429,0.242857142857143,0.257142857142857,0.271428571428571,
0.285714285714286,0.3,0.314285714285714,0.328571428571429,0.342857142857143,
0.357142857142857,0.371428571428571,0.385714285714286,0.4,0.414285714285714,
0.428571428571429,0.442857142857143,0.457142857142857,0.471428571428572,
0.485714285714286,0.5,0.514285714285714,0.528571428571429,0.542857142857143,
0.557142857142857,0.571428571428571,0.585714285714286,0.6,0.614285714285714,
0.628571428571428,0.642857142857142,0.657142857142857,0.671428571428571,
0.685714285714285,0.699999999999999,0.714285714285714,0.728571428571428,
0.742857142857142,0.757142857142856,0.771428571428571,0.785714285714285,
0.799999999999999,0.814285714285713,0.828571428571428,0.842857142857142,
0.857142857142856,0.87142857142857,0.885714285714284,0.899999999999999,
0.914285714285713,0.928571428571427,0.942857142857141,0.957142857142856,
0.97142857142857,0.985714285714284,1.),(0.,1.8),.UNSPECIFIED.);
#981=B_SPLINE_SURFACE_WITH_KNOTS('',5,1,((#29707,#29708),(#29709,#29710),
(#29711,#29712),(#29713,#29714),(#29715,#29716),(#29717,#29718),(#29719,
#29720),(#29721,#29722),(#29723,#29724),(#29725,#29726),(#29727,#29728),
(#29729,#29730),(#29731,#29732),(#29733,#29734),(#29735,#29736),(#29737,
#29738),(#29739,#29740),(#29741,#29742),(#29743,#29744),(#29745,#29746),
(#29747,#29748),(#29749,#29750),(#29751,#29752),(#29753,#29754),(#29755,
#29756),(#29757,#29758),(#29759,#29760),(#29761,#29762),(#29763,#29764),
(#29765,#29766),(#29767,#29768),(#29769,#29770),(#29771,#29772),(#29773,
#29774),(#29775,#29776),(#29777,#29778),(#29779,#29780),(#29781,#29782),
(#29783,#29784),(#29785,#29786),(#29787,#29788),(#29789,#29790),(#29791,
#29792),(#29793,#29794),(#29795,#29796),(#29797,#29798),(#29799,#29800),
(#29801,#29802),(#29803,#29804),(#29805,#29806),(#29807,#29808),(#29809,
#29810),(#29811,#29812),(#29813,#29814),(#29815,#29816),(#29817,#29818),
(#29819,#29820),(#29821,#29822),(#29823,#29824),(#29825,#29826),(#29827,
#29828),(#29829,#29830),(#29831,#29832),(#29833,#29834),(#29835,#29836),
(#29837,#29838),(#29839,#29840),(#29841,#29842),(#29843,#29844),(#29845,
#29846),(#29847,#29848),(#29849,#29850),(#29851,#29852),(#29853,#29854),
(#29855,#29856)),.UNSPECIFIED.,.F.,.F.,.F.,(6,1,1,1,1,1,1,1,1,1,1,1,1,1,
1,1,1,1,1,1,1,1,1,1,1,1,1,1,1,1,1,1,1,1,1,1,1,1,1,1,1,1,1,1,1,1,1,1,1,1,
1,1,1,1,1,1,1,1,1,1,1,1,1,1,1,1,1,1,1,1,6),(2,2),(-1.,-0.985714285714284,
-0.97142857142857,-0.957142857142856,-0.942857142857141,-0.928571428571427,
-0.914285714285713,-0.899999999999999,-0.885714285714284,-0.87142857142857,
-0.857142857142856,-0.842857142857142,-0.828571428571428,-0.814285714285713,
-0.799999999999999,-0.785714285714285,-0.771428571428571,-0.757142857142856,
-0.742857142857142,-0.728571428571428,-0.714285714285714,-0.699999999999999,
-0.685714285714285,-0.671428571428571,-0.657142857142857,-0.642857142857142,
-0.628571428571428,-0.614285714285714,-0.6,-0.585714285714286,-0.571428571428571,
-0.557142857142857,-0.542857142857143,-0.528571428571429,-0.514285714285714,
-0.5,-0.485714285714286,-0.471428571428572,-0.457142857142857,-0.442857142857143,
-0.428571428571429,-0.414285714285714,-0.4,-0.385714285714286,-0.371428571428571,
-0.357142857142857,-0.342857142857143,-0.328571428571429,-0.314285714285714,
-0.3,-0.285714285714286,-0.271428571428571,-0.257142857142857,-0.242857142857143,
-0.228571428571429,-0.214285714285714,-0.2,-0.185714285714286,-0.171428571428571,
-0.157142857142857,-0.142857142857143,-0.128571428571429,-0.114285714285714,
-0.1,-0.0857142857142857,-0.0714285714285714,-0.0571428571428571,-0.0428571428571429,
-0.0285714285714286,-0.0142857142857143,0.),(0.,1.8),.UNSPECIFIED.);
#982=B_SPLINE_SURFACE_WITH_KNOTS('',5,1,((#30015,#30016),(#30017,#30018),
(#30019,#30020),(#30021,#30022),(#30023,#30024),(#30025,#30026),(#30027,
#30028),(#30029,#30030),(#30031,#30032),(#30033,#30034),(#30035,#30036),
(#30037,#30038),(#30039,#30040),(#30041,#30042),(#30043,#30044),(#30045,
#30046),(#30047,#30048),(#30049,#30050),(#30051,#30052),(#30053,#30054),
(#30055,#30056),(#30057,#30058),(#30059,#30060),(#30061,#30062),(#30063,
#30064),(#30065,#30066),(#30067,#30068),(#30069,#30070),(#30071,#30072),
(#30073,#30074),(#30075,#30076),(#30077,#30078),(#30079,#30080),(#30081,
#30082),(#30083,#30084),(#30085,#30086),(#30087,#30088),(#30089,#30090),
(#30091,#30092),(#30093,#30094),(#30095,#30096),(#30097,#30098),(#30099,
#30100),(#30101,#30102),(#30103,#30104),(#30105,#30106),(#30107,#30108),
(#30109,#30110),(#30111,#30112),(#30113,#30114),(#30115,#30116),(#30117,
#30118),(#30119,#30120),(#30121,#30122),(#30123,#30124),(#30125,#30126),
(#30127,#30128),(#30129,#30130),(#30131,#30132),(#30133,#30134),(#30135,
#30136),(#30137,#30138),(#30139,#30140),(#30141,#30142),(#30143,#30144),
(#30145,#30146),(#30147,#30148),(#30149,#30150),(#30151,#30152),(#30153,
#30154),(#30155,#30156),(#30157,#30158),(#30159,#30160),(#30161,#30162),
(#30163,#30164)),.UNSPECIFIED.,.F.,.F.,.F.,(6,1,1,1,1,1,1,1,1,1,1,1,1,1,
1,1,1,1,1,1,1,1,1,1,1,1,1,1,1,1,1,1,1,1,1,1,1,1,1,1,1,1,1,1,1,1,1,1,1,1,
1,1,1,1,1,1,1,1,1,1,1,1,1,1,1,1,1,1,1,1,6),(2,2),(0.,0.0142857142857143,
0.0285714285714286,0.0428571428571429,0.0571428571428571,0.0714285714285714,
0.0857142857142857,0.1,0.114285714285714,0.128571428571429,0.142857142857143,
0.157142857142857,0.171428571428571,0.185714285714286,0.2,0.214285714285714,
0.228571428571429,0.242857142857143,0.257142857142857,0.271428571428571,
0.285714285714286,0.3,0.314285714285714,0.328571428571429,0.342857142857143,
0.357142857142857,0.371428571428571,0.385714285714286,0.4,0.414285714285714,
0.428571428571429,0.442857142857143,0.457142857142857,0.471428571428572,
0.485714285714286,0.5,0.514285714285714,0.528571428571429,0.542857142857143,
0.557142857142857,0.571428571428571,0.585714285714286,0.6,0.614285714285714,
0.628571428571428,0.642857142857142,0.657142857142857,0.671428571428571,
0.685714285714285,0.699999999999999,0.714285714285714,0.728571428571428,
0.742857142857142,0.757142857142856,0.771428571428571,0.785714285714285,
0.799999999999999,0.814285714285713,0.828571428571428,0.842857142857142,
0.857142857142856,0.87142857142857,0.885714285714284,0.899999999999999,
0.914285714285713,0.928571428571427,0.942857142857141,0.957142857142856,
0.97142857142857,0.985714285714284,1.),(0.,1.8),.UNSPECIFIED.);
#983=B_SPLINE_SURFACE_WITH_KNOTS('',5,1,((#30313,#30314),(#30315,#30316),
(#30317,#30318),(#30319,#30320),(#30321,#30322),(#30323,#30324),(#30325,
#30326),(#30327,#30328),(#30329,#30330),(#30331,#30332),(#30333,#30334),
(#30335,#30336),(#30337,#30338),(#30339,#30340),(#30341,#30342),(#30343,
#30344),(#30345,#30346),(#30347,#30348),(#30349,#30350),(#30351,#30352),
(#30353,#30354),(#30355,#30356),(#30357,#30358),(#30359,#30360),(#30361,
#30362),(#30363,#30364),(#30365,#30366),(#30367,#30368),(#30369,#30370),
(#30371,#30372),(#30373,#30374),(#30375,#30376),(#30377,#30378),(#30379,
#30380),(#30381,#30382),(#30383,#30384),(#30385,#30386),(#30387,#30388),
(#30389,#30390),(#30391,#30392),(#30393,#30394),(#30395,#30396),(#30397,
#30398),(#30399,#30400),(#30401,#30402),(#30403,#30404),(#30405,#30406),
(#30407,#30408),(#30409,#30410),(#30411,#30412),(#30413,#30414),(#30415,
#30416),(#30417,#30418),(#30419,#30420),(#30421,#30422),(#30423,#30424),
(#30425,#30426),(#30427,#30428),(#30429,#30430),(#30431,#30432),(#30433,
#30434),(#30435,#30436),(#30437,#30438),(#30439,#30440),(#30441,#30442),
(#30443,#30444),(#30445,#30446),(#30447,#30448),(#30449,#30450),(#30451,
#30452),(#30453,#30454),(#30455,#30456),(#30457,#30458),(#30459,#30460),
(#30461,#30462)),.UNSPECIFIED.,.F.,.F.,.F.,(6,1,1,1,1,1,1,1,1,1,1,1,1,1,
1,1,1,1,1,1,1,1,1,1,1,1,1,1,1,1,1,1,1,1,1,1,1,1,1,1,1,1,1,1,1,1,1,1,1,1,
1,1,1,1,1,1,1,1,1,1,1,1,1,1,1,1,1,1,1,1,6),(2,2),(-1.,-0.985714285714284,
-0.97142857142857,-0.957142857142856,-0.942857142857141,-0.928571428571427,
-0.914285714285713,-0.899999999999999,-0.885714285714284,-0.87142857142857,
-0.857142857142856,-0.842857142857142,-0.828571428571428,-0.814285714285713,
-0.799999999999999,-0.785714285714285,-0.771428571428571,-0.757142857142856,
-0.742857142857142,-0.728571428571428,-0.714285714285714,-0.699999999999999,
-0.685714285714285,-0.671428571428571,-0.657142857142857,-0.642857142857142,
-0.628571428571428,-0.614285714285714,-0.6,-0.585714285714286,-0.571428571428571,
-0.557142857142857,-0.542857142857143,-0.528571428571429,-0.514285714285714,
-0.5,-0.485714285714286,-0.471428571428572,-0.457142857142857,-0.442857142857143,
-0.428571428571429,-0.414285714285714,-0.4,-0.385714285714286,-0.371428571428571,
-0.357142857142857,-0.342857142857143,-0.328571428571429,-0.314285714285714,
-0.3,-0.285714285714286,-0.271428571428571,-0.257142857142857,-0.242857142857143,
-0.228571428571429,-0.214285714285714,-0.2,-0.185714285714286,-0.171428571428571,
-0.157142857142857,-0.142857142857143,-0.128571428571429,-0.114285714285714,
-0.1,-0.0857142857142857,-0.0714285714285714,-0.0571428571428571,-0.0428571428571429,
-0.0285714285714286,-0.0142857142857143,0.),(0.,1.8),.UNSPECIFIED.);
#984=B_SPLINE_SURFACE_WITH_KNOTS('',5,1,((#30621,#30622),(#30623,#30624),
(#30625,#30626),(#30627,#30628),(#30629,#30630),(#30631,#30632),(#30633,
#30634),(#30635,#30636),(#30637,#30638),(#30639,#30640),(#30641,#30642),
(#30643,#30644),(#30645,#30646),(#30647,#30648),(#30649,#30650),(#30651,
#30652),(#30653,#30654),(#30655,#30656),(#30657,#30658),(#30659,#30660),
(#30661,#30662),(#30663,#30664),(#30665,#30666),(#30667,#30668),(#30669,
#30670),(#30671,#30672),(#30673,#30674),(#30675,#30676),(#30677,#30678),
(#30679,#30680),(#30681,#30682),(#30683,#30684),(#30685,#30686),(#30687,
#30688),(#30689,#30690),(#30691,#30692),(#30693,#30694),(#30695,#30696),
(#30697,#30698),(#30699,#30700),(#30701,#30702),(#30703,#30704),(#30705,
#30706),(#30707,#30708),(#30709,#30710),(#30711,#30712),(#30713,#30714),
(#30715,#30716),(#30717,#30718),(#30719,#30720),(#30721,#30722),(#30723,
#30724),(#30725,#30726),(#30727,#30728),(#30729,#30730),(#30731,#30732),
(#30733,#30734),(#30735,#30736),(#30737,#30738),(#30739,#30740),(#30741,
#30742),(#30743,#30744),(#30745,#30746),(#30747,#30748),(#30749,#30750),
(#30751,#30752),(#30753,#30754),(#30755,#30756),(#30757,#30758),(#30759,
#30760),(#30761,#30762),(#30763,#30764),(#30765,#30766),(#30767,#30768),
(#30769,#30770)),.UNSPECIFIED.,.F.,.F.,.F.,(6,1,1,1,1,1,1,1,1,1,1,1,1,1,
1,1,1,1,1,1,1,1,1,1,1,1,1,1,1,1,1,1,1,1,1,1,1,1,1,1,1,1,1,1,1,1,1,1,1,1,
1,1,1,1,1,1,1,1,1,1,1,1,1,1,1,1,1,1,1,1,6),(2,2),(0.,0.0142857142857143,
0.0285714285714286,0.0428571428571429,0.0571428571428571,0.0714285714285714,
0.0857142857142857,0.1,0.114285714285714,0.128571428571429,0.142857142857143,
0.157142857142857,0.171428571428571,0.185714285714286,0.2,0.214285714285714,
0.228571428571429,0.242857142857143,0.257142857142857,0.271428571428571,
0.285714285714286,0.3,0.314285714285714,0.328571428571429,0.342857142857143,
0.357142857142857,0.371428571428571,0.385714285714286,0.4,0.414285714285714,
0.428571428571429,0.442857142857143,0.457142857142857,0.471428571428572,
0.485714285714286,0.5,0.514285714285714,0.528571428571429,0.542857142857143,
0.557142857142857,0.571428571428571,0.585714285714286,0.6,0.614285714285714,
0.628571428571428,0.642857142857142,0.657142857142857,0.671428571428571,
0.685714285714285,0.699999999999999,0.714285714285714,0.728571428571428,
0.742857142857142,0.757142857142856,0.771428571428571,0.785714285714285,
0.799999999999999,0.814285714285713,0.828571428571428,0.842857142857142,
0.857142857142856,0.87142857142857,0.885714285714284,0.899999999999999,
0.914285714285713,0.928571428571427,0.942857142857141,0.957142857142856,
0.97142857142857,0.985714285714284,1.),(0.,1.8),.UNSPECIFIED.);
#985=B_SPLINE_SURFACE_WITH_KNOTS('',5,1,((#31313,#31314),(#31315,#31316),
(#31317,#31318),(#31319,#31320),(#31321,#31322),(#31323,#31324),(#31325,
#31326),(#31327,#31328),(#31329,#31330),(#31331,#31332),(#31333,#31334),
(#31335,#31336),(#31337,#31338),(#31339,#31340),(#31341,#31342),(#31343,
#31344),(#31345,#31346),(#31347,#31348),(#31349,#31350),(#31351,#31352),
(#31353,#31354),(#31355,#31356),(#31357,#31358),(#31359,#31360),(#31361,
#31362),(#31363,#31364),(#31365,#31366),(#31367,#31368),(#31369,#31370),
(#31371,#31372),(#31373,#31374),(#31375,#31376),(#31377,#31378),(#31379,
#31380),(#31381,#31382),(#31383,#31384),(#31385,#31386),(#31387,#31388),
(#31389,#31390),(#31391,#31392),(#31393,#31394),(#31395,#31396),(#31397,
#31398),(#31399,#31400),(#31401,#31402),(#31403,#31404),(#31405,#31406),
(#31407,#31408),(#31409,#31410),(#31411,#31412),(#31413,#31414),(#31415,
#31416),(#31417,#31418),(#31419,#31420),(#31421,#31422),(#31423,#31424),
(#31425,#31426),(#31427,#31428),(#31429,#31430),(#31431,#31432),(#31433,
#31434),(#31435,#31436),(#31437,#31438),(#31439,#31440),(#31441,#31442),
(#31443,#31444),(#31445,#31446),(#31447,#31448),(#31449,#31450),(#31451,
#31452),(#31453,#31454),(#31455,#31456),(#31457,#31458),(#31459,#31460),
(#31461,#31462)),.UNSPECIFIED.,.F.,.F.,.F.,(6,1,1,1,1,1,1,1,1,1,1,1,1,1,
1,1,1,1,1,1,1,1,1,1,1,1,1,1,1,1,1,1,1,1,1,1,1,1,1,1,1,1,1,1,1,1,1,1,1,1,
1,1,1,1,1,1,1,1,1,1,1,1,1,1,1,1,1,1,1,1,6),(2,2),(-1.,-0.985714285714284,
-0.97142857142857,-0.957142857142856,-0.942857142857141,-0.928571428571427,
-0.914285714285713,-0.899999999999999,-0.885714285714284,-0.87142857142857,
-0.857142857142856,-0.842857142857142,-0.828571428571428,-0.814285714285713,
-0.799999999999999,-0.785714285714285,-0.771428571428571,-0.757142857142856,
-0.742857142857142,-0.728571428571428,-0.714285714285714,-0.699999999999999,
-0.685714285714285,-0.671428571428571,-0.657142857142857,-0.642857142857142,
-0.628571428571428,-0.614285714285714,-0.6,-0.585714285714286,-0.571428571428571,
-0.557142857142857,-0.542857142857143,-0.528571428571429,-0.514285714285714,
-0.5,-0.485714285714286,-0.471428571428572,-0.457142857142857,-0.442857142857143,
-0.428571428571429,-0.414285714285714,-0.4,-0.385714285714286,-0.371428571428571,
-0.357142857142857,-0.342857142857143,-0.328571428571429,-0.314285714285714,
-0.3,-0.285714285714286,-0.271428571428571,-0.257142857142857,-0.242857142857143,
-0.228571428571429,-0.214285714285714,-0.2,-0.185714285714286,-0.171428571428571,
-0.157142857142857,-0.142857142857143,-0.128571428571429,-0.114285714285714,
-0.1,-0.0857142857142857,-0.0714285714285714,-0.0571428571428571,-0.0428571428571429,
-0.0285714285714286,-0.0142857142857143,0.),(0.,1.8),.UNSPECIFIED.);
#986=B_SPLINE_SURFACE_WITH_KNOTS('',5,1,((#31466,#31467),(#31468,#31469),
(#31470,#31471),(#31472,#31473),(#31474,#31475),(#31476,#31477),(#31478,
#31479),(#31480,#31481),(#31482,#31483),(#31484,#31485),(#31486,#31487),
(#31488,#31489),(#31490,#31491),(#31492,#31493),(#31494,#31495),(#31496,
#31497),(#31498,#31499),(#31500,#31501),(#31502,#31503),(#31504,#31505),
(#31506,#31507),(#31508,#31509),(#31510,#31511),(#31512,#31513),(#31514,
#31515),(#31516,#31517),(#31518,#31519),(#31520,#31521),(#31522,#31523),
(#31524,#31525),(#31526,#31527),(#31528,#31529),(#31530,#31531),(#31532,
#31533),(#31534,#31535),(#31536,#31537),(#31538,#31539),(#31540,#31541),
(#31542,#31543),(#31544,#31545),(#31546,#31547),(#31548,#31549),(#31550,
#31551),(#31552,#31553),(#31554,#31555),(#31556,#31557),(#31558,#31559),
(#31560,#31561),(#31562,#31563),(#31564,#31565),(#31566,#31567),(#31568,
#31569),(#31570,#31571),(#31572,#31573),(#31574,#31575),(#31576,#31577),
(#31578,#31579),(#31580,#31581),(#31582,#31583),(#31584,#31585),(#31586,
#31587),(#31588,#31589),(#31590,#31591),(#31592,#31593),(#31594,#31595),
(#31596,#31597),(#31598,#31599),(#31600,#31601),(#31602,#31603),(#31604,
#31605),(#31606,#31607),(#31608,#31609),(#31610,#31611),(#31612,#31613),
(#31614,#31615)),.UNSPECIFIED.,.F.,.F.,.F.,(6,1,1,1,1,1,1,1,1,1,1,1,1,1,
1,1,1,1,1,1,1,1,1,1,1,1,1,1,1,1,1,1,1,1,1,1,1,1,1,1,1,1,1,1,1,1,1,1,1,1,
1,1,1,1,1,1,1,1,1,1,1,1,1,1,1,1,1,1,1,1,6),(2,2),(0.,0.0142857142857143,
0.0285714285714286,0.0428571428571429,0.0571428571428571,0.0714285714285714,
0.0857142857142857,0.1,0.114285714285714,0.128571428571429,0.142857142857143,
0.157142857142857,0.171428571428571,0.185714285714286,0.2,0.214285714285714,
0.228571428571429,0.242857142857143,0.257142857142857,0.271428571428571,
0.285714285714286,0.3,0.314285714285714,0.328571428571429,0.342857142857143,
0.357142857142857,0.371428571428571,0.385714285714286,0.4,0.414285714285714,
0.428571428571429,0.442857142857143,0.457142857142857,0.471428571428572,
0.485714285714286,0.5,0.514285714285714,0.528571428571429,0.542857142857143,
0.557142857142857,0.571428571428571,0.585714285714286,0.6,0.614285714285714,
0.628571428571428,0.642857142857142,0.657142857142857,0.671428571428571,
0.685714285714285,0.699999999999999,0.714285714285714,0.728571428571428,
0.742857142857142,0.757142857142856,0.771428571428571,0.785714285714285,
0.799999999999999,0.814285714285713,0.828571428571428,0.842857142857142,
0.857142857142856,0.87142857142857,0.885714285714284,0.899999999999999,
0.914285714285713,0.928571428571427,0.942857142857141,0.957142857142856,
0.97142857142857,0.985714285714284,1.),(0.,1.8),.UNSPECIFIED.);
#1007=PLANE('',#13192);
#1008=PLANE('',#13193);
#1009=PLANE('',#13197);
#1010=PLANE('',#13201);
#1011=PLANE('',#13205);
#1012=PLANE('',#13209);
#1013=PLANE('',#13213);
#1014=PLANE('',#13217);
#1015=PLANE('',#13221);
#1016=PLANE('',#13225);
#1017=PLANE('',#13229);
#1018=PLANE('',#13233);
#1019=PLANE('',#13237);
#1020=PLANE('',#13241);
#1021=PLANE('',#13245);
#1022=PLANE('',#13249);
#1023=PLANE('',#13253);
#1024=PLANE('',#13257);
#1025=PLANE('',#13261);
#1026=PLANE('',#13265);
#1027=PLANE('',#13269);
#1028=PLANE('',#13273);
#1029=PLANE('',#13277);
#1030=PLANE('',#13281);
#1031=PLANE('',#13285);
#1032=PLANE('',#13289);
#1033=PLANE('',#13293);
#1034=PLANE('',#13297);
#1035=PLANE('',#13301);
#1036=PLANE('',#13305);
#1037=PLANE('',#13309);
#1038=PLANE('',#13313);
#1039=PLANE('',#13317);
#1040=PLANE('',#13321);
#1041=PLANE('',#13325);
#1042=PLANE('',#13329);
#1043=PLANE('',#13333);
#1044=PLANE('',#13337);
#1045=PLANE('',#13341);
#1046=PLANE('',#13345);
#1047=PLANE('',#13403);
#1048=PLANE('',#13427);
#1049=PLANE('',#13471);
#1050=PLANE('',#13473);
#1287=FACE_OUTER_BOUND('',#2039,.T.);
#1288=FACE_OUTER_BOUND('',#2040,.T.);
#1289=FACE_OUTER_BOUND('',#2041,.T.);
#1290=FACE_OUTER_BOUND('',#2042,.T.);
#1291=FACE_OUTER_BOUND('',#2043,.T.);
#1292=FACE_OUTER_BOUND('',#2044,.T.);
#1293=FACE_OUTER_BOUND('',#2045,.T.);
#1294=FACE_OUTER_BOUND('',#2046,.T.);
#1295=FACE_OUTER_BOUND('',#2047,.T.);
#1296=FACE_OUTER_BOUND('',#2048,.T.);
#1297=FACE_OUTER_BOUND('',#2049,.T.);
#1298=FACE_OUTER_BOUND('',#2050,.T.);
#1299=FACE_OUTER_BOUND('',#2051,.T.);
#1300=FACE_OUTER_BOUND('',#2052,.T.);
#1301=FACE_OUTER_BOUND('',#2053,.T.);
#1302=FACE_OUTER_BOUND('',#2054,.T.);
#1303=FACE_OUTER_BOUND('',#2055,.T.);
#1304=FACE_OUTER_BOUND('',#2056,.T.);
#1305=FACE_OUTER_BOUND('',#2057,.T.);
#1306=FACE_OUTER_BOUND('',#2058,.T.);
#1307=FACE_OUTER_BOUND('',#2059,.T.);
#1308=FACE_OUTER_BOUND('',#2060,.T.);
#1309=FACE_OUTER_BOUND('',#2061,.T.);
#1310=FACE_OUTER_BOUND('',#2062,.T.);
#1311=FACE_OUTER_BOUND('',#2063,.T.);
#1312=FACE_OUTER_BOUND('',#2064,.T.);
#1313=FACE_OUTER_BOUND('',#2065,.T.);
#1314=FACE_OUTER_BOUND('',#2066,.T.);
#1315=FACE_OUTER_BOUND('',#2067,.T.);
#1316=FACE_OUTER_BOUND('',#2068,.T.);
#1317=FACE_OUTER_BOUND('',#2069,.T.);
#1318=FACE_OUTER_BOUND('',#2070,.T.);
#1319=FACE_OUTER_BOUND('',#2071,.T.);
#1320=FACE_OUTER_BOUND('',#2072,.T.);
#1321=FACE_OUTER_BOUND('',#2073,.T.);
#1322=FACE_OUTER_BOUND('',#2074,.T.);
#1323=FACE_OUTER_BOUND('',#2075,.T.);
#1324=FACE_OUTER_BOUND('',#2076,.T.);
#1325=FACE_OUTER_BOUND('',#2077,.T.);
#1326=FACE_OUTER_BOUND('',#2078,.T.);
#1327=FACE_OUTER_BOUND('',#2079,.T.);
#1328=FACE_OUTER_BOUND('',#2080,.T.);
#1329=FACE_OUTER_BOUND('',#2081,.T.);
#1330=FACE_OUTER_BOUND('',#2082,.T.);
#1331=FACE_OUTER_BOUND('',#2083,.T.);
#1332=FACE_OUTER_BOUND('',#2084,.T.);
#1333=FACE_OUTER_BOUND('',#2085,.T.);
#1334=FACE_OUTER_BOUND('',#2086,.T.);
#1335=FACE_OUTER_BOUND('',#2087,.T.);
#1336=FACE_OUTER_BOUND('',#2088,.T.);
#1337=FACE_OUTER_BOUND('',#2089,.T.);
#1338=FACE_OUTER_BOUND('',#2090,.T.);
#1339=FACE_OUTER_BOUND('',#2091,.T.);
#1340=FACE_OUTER_BOUND('',#2092,.T.);
#1341=FACE_OUTER_BOUND('',#2093,.T.);
#1342=FACE_OUTER_BOUND('',#2094,.T.);
#1343=FACE_OUTER_BOUND('',#2095,.T.);
#1344=FACE_OUTER_BOUND('',#2096,.T.);
#1345=FACE_OUTER_BOUND('',#2097,.T.);
#1346=FACE_OUTER_BOUND('',#2098,.T.);
#1347=FACE_OUTER_BOUND('',#2099,.T.);
#1348=FACE_OUTER_BOUND('',#2100,.T.);
#1349=FACE_OUTER_BOUND('',#2101,.T.);
#1350=FACE_OUTER_BOUND('',#2102,.T.);
#1351=FACE_OUTER_BOUND('',#2103,.T.);
#1352=FACE_OUTER_BOUND('',#2104,.T.);
#1353=FACE_OUTER_BOUND('',#2105,.T.);
#1354=FACE_OUTER_BOUND('',#2106,.T.);
#1355=FACE_OUTER_BOUND('',#2107,.T.);
#1356=FACE_OUTER_BOUND('',#2108,.T.);
#1357=FACE_OUTER_BOUND('',#2109,.T.);
#1358=FACE_OUTER_BOUND('',#2110,.T.);
#1359=FACE_OUTER_BOUND('',#2111,.T.);
#1360=FACE_OUTER_BOUND('',#2112,.T.);
#1361=FACE_OUTER_BOUND('',#2113,.T.);
#1362=FACE_OUTER_BOUND('',#2114,.T.);
#1363=FACE_OUTER_BOUND('',#2115,.T.);
#1364=FACE_OUTER_BOUND('',#2116,.T.);
#1365=FACE_OUTER_BOUND('',#2117,.T.);
#1366=FACE_OUTER_BOUND('',#2118,.T.);
#1367=FACE_OUTER_BOUND('',#2119,.T.);
#1368=FACE_OUTER_BOUND('',#2120,.T.);
#1369=FACE_OUTER_BOUND('',#2121,.T.);
#1370=FACE_OUTER_BOUND('',#2122,.T.);
#1371=FACE_OUTER_BOUND('',#2123,.T.);
#1372=FACE_OUTER_BOUND('',#2124,.T.);
#1373=FACE_OUTER_BOUND('',#2125,.T.);
#1374=FACE_OUTER_BOUND('',#2126,.T.);
#1375=FACE_OUTER_BOUND('',#2127,.T.);
#1376=FACE_OUTER_BOUND('',#2128,.T.);
#1377=FACE_OUTER_BOUND('',#2129,.T.);
#1378=FACE_OUTER_BOUND('',#2130,.T.);
#1379=FACE_OUTER_BOUND('',#2131,.T.);
#1380=FACE_OUTER_BOUND('',#2132,.T.);
#1381=FACE_OUTER_BOUND('',#2133,.T.);
#1382=FACE_OUTER_BOUND('',#2134,.T.);
#1383=FACE_OUTER_BOUND('',#2135,.T.);
#1384=FACE_OUTER_BOUND('',#2136,.T.);
#1385=FACE_OUTER_BOUND('',#2137,.T.);
#1386=FACE_OUTER_BOUND('',#2138,.T.);
#1387=FACE_OUTER_BOUND('',#2139,.T.);
#1388=FACE_OUTER_BOUND('',#2140,.T.);
#1389=FACE_OUTER_BOUND('',#2141,.T.);
#1390=FACE_OUTER_BOUND('',#2142,.T.);
#1391=FACE_OUTER_BOUND('',#2143,.T.);
#1392=FACE_OUTER_BOUND('',#2144,.T.);
#1393=FACE_OUTER_BOUND('',#2145,.T.);
#1394=FACE_OUTER_BOUND('',#2146,.T.);
#1395=FACE_OUTER_BOUND('',#2147,.T.);
#1396=FACE_OUTER_BOUND('',#2148,.T.);
#1397=FACE_OUTER_BOUND('',#2149,.T.);
#1398=FACE_OUTER_BOUND('',#2150,.T.);
#1399=FACE_OUTER_BOUND('',#2151,.T.);
#1400=FACE_OUTER_BOUND('',#2152,.T.);
#1401=FACE_OUTER_BOUND('',#2153,.T.);
#1402=FACE_OUTER_BOUND('',#2154,.T.);
#1403=FACE_OUTER_BOUND('',#2155,.T.);
#1404=FACE_OUTER_BOUND('',#2156,.T.);
#1405=FACE_OUTER_BOUND('',#2157,.T.);
#1406=FACE_OUTER_BOUND('',#2158,.T.);
#1407=FACE_OUTER_BOUND('',#2159,.T.);
#1408=FACE_OUTER_BOUND('',#2160,.T.);
#1409=FACE_OUTER_BOUND('',#2161,.T.);
#1410=FACE_OUTER_BOUND('',#2162,.T.);
#1411=FACE_OUTER_BOUND('',#2163,.T.);
#1412=FACE_OUTER_BOUND('',#2164,.T.);
#1413=FACE_OUTER_BOUND('',#2165,.T.);
#1414=FACE_OUTER_BOUND('',#2166,.T.);
#1415=FACE_OUTER_BOUND('',#2167,.T.);
#1416=FACE_OUTER_BOUND('',#2168,.T.);
#1417=FACE_OUTER_BOUND('',#2169,.T.);
#1418=FACE_OUTER_BOUND('',#2170,.T.);
#1419=FACE_OUTER_BOUND('',#2171,.T.);
#1420=FACE_OUTER_BOUND('',#2172,.T.);
#1421=FACE_OUTER_BOUND('',#2173,.T.);
#1422=FACE_OUTER_BOUND('',#2174,.T.);
#1423=FACE_OUTER_BOUND('',#2175,.T.);
#1424=FACE_OUTER_BOUND('',#2176,.T.);
#1425=FACE_OUTER_BOUND('',#2178,.T.);
#1426=FACE_OUTER_BOUND('',#2180,.T.);
#1427=FACE_OUTER_BOUND('',#2181,.T.);
#1428=FACE_OUTER_BOUND('',#2182,.T.);
#1429=FACE_OUTER_BOUND('',#2183,.T.);
#1430=FACE_OUTER_BOUND('',#2184,.T.);
#1431=FACE_OUTER_BOUND('',#2185,.T.);
#1432=FACE_OUTER_BOUND('',#2186,.T.);
#1433=FACE_OUTER_BOUND('',#2187,.T.);
#1434=FACE_OUTER_BOUND('',#2188,.T.);
#1435=FACE_OUTER_BOUND('',#2189,.T.);
#1436=FACE_OUTER_BOUND('',#2190,.T.);
#1437=FACE_OUTER_BOUND('',#2191,.T.);
#1438=FACE_OUTER_BOUND('',#2192,.T.);
#1439=FACE_OUTER_BOUND('',#2193,.T.);
#1440=FACE_OUTER_BOUND('',#2194,.T.);
#1441=FACE_OUTER_BOUND('',#2195,.T.);
#1442=FACE_OUTER_BOUND('',#2196,.T.);
#1443=FACE_OUTER_BOUND('',#2197,.T.);
#1444=FACE_OUTER_BOUND('',#2198,.T.);
#1445=FACE_OUTER_BOUND('',#2199,.T.);
#1446=FACE_OUTER_BOUND('',#2200,.T.);
#1447=FACE_OUTER_BOUND('',#2201,.T.);
#1448=FACE_OUTER_BOUND('',#2202,.T.);
#1449=FACE_OUTER_BOUND('',#2203,.T.);
#1450=FACE_OUTER_BOUND('',#2204,.T.);
#1451=FACE_OUTER_BOUND('',#2205,.T.);
#1452=FACE_OUTER_BOUND('',#2206,.T.);
#2039=EDGE_LOOP('',(#8171,#8172,#8173,#8174));
#2040=EDGE_LOOP('',(#8175,#8176,#8177,#8178));
#2041=EDGE_LOOP('',(#8179));
#2042=EDGE_LOOP('',(#8180));
#2043=EDGE_LOOP('',(#8181,#8182,#8183,#8184));
#2044=EDGE_LOOP('',(#8185,#8186,#8187,#8188));
#2045=EDGE_LOOP('',(#8189,#8190,#8191,#8192));
#2046=EDGE_LOOP('',(#8193,#8194,#8195,#8196));
#2047=EDGE_LOOP('',(#8197,#8198,#8199,#8200));
#2048=EDGE_LOOP('',(#8201,#8202,#8203,#8204));
#2049=EDGE_LOOP('',(#8205,#8206,#8207,#8208));
#2050=EDGE_LOOP('',(#8209,#8210,#8211,#8212));
#2051=EDGE_LOOP('',(#8213,#8214,#8215,#8216));
#2052=EDGE_LOOP('',(#8217,#8218,#8219,#8220));
#2053=EDGE_LOOP('',(#8221,#8222,#8223,#8224));
#2054=EDGE_LOOP('',(#8225,#8226,#8227,#8228));
#2055=EDGE_LOOP('',(#8229,#8230,#8231,#8232));
#2056=EDGE_LOOP('',(#8233,#8234,#8235,#8236));
#2057=EDGE_LOOP('',(#8237,#8238,#8239,#8240));
#2058=EDGE_LOOP('',(#8241,#8242,#8243,#8244));
#2059=EDGE_LOOP('',(#8245,#8246,#8247,#8248));
#2060=EDGE_LOOP('',(#8249,#8250,#8251,#8252));
#2061=EDGE_LOOP('',(#8253,#8254,#8255,#8256));
#2062=EDGE_LOOP('',(#8257,#8258,#8259,#8260));
#2063=EDGE_LOOP('',(#8261,#8262,#8263,#8264));
#2064=EDGE_LOOP('',(#8265,#8266,#8267,#8268));
#2065=EDGE_LOOP('',(#8269,#8270,#8271,#8272));
#2066=EDGE_LOOP('',(#8273,#8274,#8275,#8276));
#2067=EDGE_LOOP('',(#8277,#8278,#8279,#8280));
#2068=EDGE_LOOP('',(#8281,#8282,#8283,#8284));
#2069=EDGE_LOOP('',(#8285,#8286,#8287,#8288));
#2070=EDGE_LOOP('',(#8289,#8290,#8291,#8292));
#2071=EDGE_LOOP('',(#8293,#8294,#8295,#8296));
#2072=EDGE_LOOP('',(#8297,#8298,#8299,#8300));
#2073=EDGE_LOOP('',(#8301,#8302,#8303,#8304));
#2074=EDGE_LOOP('',(#8305,#8306,#8307,#8308));
#2075=EDGE_LOOP('',(#8309,#8310,#8311,#8312));
#2076=EDGE_LOOP('',(#8313,#8314,#8315,#8316));
#2077=EDGE_LOOP('',(#8317,#8318,#8319,#8320));
#2078=EDGE_LOOP('',(#8321,#8322,#8323,#8324));
#2079=EDGE_LOOP('',(#8325,#8326,#8327,#8328));
#2080=EDGE_LOOP('',(#8329,#8330,#8331,#8332));
#2081=EDGE_LOOP('',(#8333,#8334,#8335,#8336));
#2082=EDGE_LOOP('',(#8337,#8338,#8339,#8340));
#2083=EDGE_LOOP('',(#8341,#8342,#8343,#8344));
#2084=EDGE_LOOP('',(#8345,#8346,#8347,#8348));
#2085=EDGE_LOOP('',(#8349,#8350,#8351,#8352));
#2086=EDGE_LOOP('',(#8353,#8354,#8355,#8356));
#2087=EDGE_LOOP('',(#8357,#8358,#8359,#8360));
#2088=EDGE_LOOP('',(#8361,#8362,#8363,#8364));
#2089=EDGE_LOOP('',(#8365,#8366,#8367,#8368));
#2090=EDGE_LOOP('',(#8369,#8370,#8371,#8372));
#2091=EDGE_LOOP('',(#8373,#8374,#8375,#8376));
#2092=EDGE_LOOP('',(#8377,#8378,#8379,#8380));
#2093=EDGE_LOOP('',(#8381,#8382,#8383,#8384));
#2094=EDGE_LOOP('',(#8385,#8386,#8387,#8388));
#2095=EDGE_LOOP('',(#8389,#8390,#8391,#8392));
#2096=EDGE_LOOP('',(#8393,#8394,#8395,#8396));
#2097=EDGE_LOOP('',(#8397,#8398,#8399,#8400));
#2098=EDGE_LOOP('',(#8401,#8402,#8403,#8404));
#2099=EDGE_LOOP('',(#8405,#8406,#8407,#8408));
#2100=EDGE_LOOP('',(#8409,#8410,#8411,#8412));
#2101=EDGE_LOOP('',(#8413,#8414,#8415,#8416));
#2102=EDGE_LOOP('',(#8417,#8418,#8419,#8420));
#2103=EDGE_LOOP('',(#8421,#8422,#8423,#8424));
#2104=EDGE_LOOP('',(#8425,#8426,#8427,#8428));
#2105=EDGE_LOOP('',(#8429,#8430,#8431,#8432));
#2106=EDGE_LOOP('',(#8433,#8434,#8435,#8436));
#2107=EDGE_LOOP('',(#8437,#8438,#8439,#8440));
#2108=EDGE_LOOP('',(#8441,#8442,#8443,#8444));
#2109=EDGE_LOOP('',(#8445,#8446,#8447,#8448));
#2110=EDGE_LOOP('',(#8449,#8450,#8451,#8452));
#2111=EDGE_LOOP('',(#8453,#8454,#8455,#8456));
#2112=EDGE_LOOP('',(#8457,#8458,#8459,#8460));
#2113=EDGE_LOOP('',(#8461,#8462,#8463,#8464));
#2114=EDGE_LOOP('',(#8465,#8466,#8467,#8468));
#2115=EDGE_LOOP('',(#8469,#8470,#8471,#8472));
#2116=EDGE_LOOP('',(#8473,#8474,#8475,#8476));
#2117=EDGE_LOOP('',(#8477,#8478,#8479,#8480));
#2118=EDGE_LOOP('',(#8481,#8482,#8483,#8484));
#2119=EDGE_LOOP('',(#8485,#8486,#8487,#8488));
#2120=EDGE_LOOP('',(#8489,#8490,#8491,#8492));
#2121=EDGE_LOOP('',(#8493,#8494,#8495,#8496));
#2122=EDGE_LOOP('',(#8497,#8498,#8499,#8500));
#2123=EDGE_LOOP('',(#8501,#8502,#8503,#8504));
#2124=EDGE_LOOP('',(#8505,#8506,#8507,#8508));
#2125=EDGE_LOOP('',(#8509,#8510,#8511,#8512));
#2126=EDGE_LOOP('',(#8513,#8514,#8515,#8516));
#2127=EDGE_LOOP('',(#8517,#8518,#8519,#8520));
#2128=EDGE_LOOP('',(#8521,#8522,#8523,#8524));
#2129=EDGE_LOOP('',(#8525,#8526,#8527,#8528));
#2130=EDGE_LOOP('',(#8529,#8530,#8531,#8532));
#2131=EDGE_LOOP('',(#8533,#8534,#8535,#8536));
#2132=EDGE_LOOP('',(#8537,#8538,#8539,#8540));
#2133=EDGE_LOOP('',(#8541,#8542,#8543,#8544));
#2134=EDGE_LOOP('',(#8545,#8546,#8547,#8548));
#2135=EDGE_LOOP('',(#8549,#8550,#8551,#8552));
#2136=EDGE_LOOP('',(#8553,#8554,#8555,#8556));
#2137=EDGE_LOOP('',(#8557,#8558,#8559,#8560));
#2138=EDGE_LOOP('',(#8561,#8562,#8563,#8564));
#2139=EDGE_LOOP('',(#8565,#8566,#8567,#8568));
#2140=EDGE_LOOP('',(#8569,#8570,#8571,#8572));
#2141=EDGE_LOOP('',(#8573,#8574,#8575,#8576));
#2142=EDGE_LOOP('',(#8577,#8578,#8579,#8580));
#2143=EDGE_LOOP('',(#8581,#8582,#8583,#8584));
#2144=EDGE_LOOP('',(#8585,#8586,#8587,#8588));
#2145=EDGE_LOOP('',(#8589,#8590,#8591,#8592));
#2146=EDGE_LOOP('',(#8593,#8594,#8595,#8596));
#2147=EDGE_LOOP('',(#8597,#8598,#8599,#8600));
#2148=EDGE_LOOP('',(#8601,#8602,#8603,#8604));
#2149=EDGE_LOOP('',(#8605,#8606,#8607,#8608));
#2150=EDGE_LOOP('',(#8609,#8610,#8611,#8612));
#2151=EDGE_LOOP('',(#8613,#8614,#8615,#8616));
#2152=EDGE_LOOP('',(#8617,#8618,#8619,#8620));
#2153=EDGE_LOOP('',(#8621,#8622,#8623,#8624));
#2154=EDGE_LOOP('',(#8625,#8626,#8627,#8628));
#2155=EDGE_LOOP('',(#8629,#8630,#8631,#8632));
#2156=EDGE_LOOP('',(#8633,#8634,#8635,#8636));
#2157=EDGE_LOOP('',(#8637,#8638,#8639,#8640));
#2158=EDGE_LOOP('',(#8641,#8642,#8643,#8644));
#2159=EDGE_LOOP('',(#8645,#8646,#8647,#8648));
#2160=EDGE_LOOP('',(#8649,#8650,#8651,#8652));
#2161=EDGE_LOOP('',(#8653,#8654,#8655,#8656));
#2162=EDGE_LOOP('',(#8657,#8658,#8659,#8660));
#2163=EDGE_LOOP('',(#8661,#8662,#8663,#8664));
#2164=EDGE_LOOP('',(#8665,#8666,#8667,#8668));
#2165=EDGE_LOOP('',(#8669,#8670,#8671,#8672));
#2166=EDGE_LOOP('',(#8673,#8674,#8675,#8676));
#2167=EDGE_LOOP('',(#8677,#8678,#8679,#8680));
#2168=EDGE_LOOP('',(#8681,#8682,#8683,#8684));
#2169=EDGE_LOOP('',(#8685,#8686,#8687,#8688));
#2170=EDGE_LOOP('',(#8689,#8690,#8691,#8692));
#2171=EDGE_LOOP('',(#8693,#8694,#8695,#8696));
#2172=EDGE_LOOP('',(#8697,#8698,#8699,#8700));
#2173=EDGE_LOOP('',(#8701,#8702,#8703,#8704));
#2174=EDGE_LOOP('',(#8705,#8706,#8707,#8708));
#2175=EDGE_LOOP('',(#8709,#8710,#8711,#8712));
#2176=EDGE_LOOP('',(#8713,#8714,#8715,#8716,#8717,#8718,#8719,#8720,#8721,
#8722,#8723,#8724,#8725,#8726,#8727,#8728,#8729,#8730,#8731,#8732,#8733,
#8734,#8735,#8736,#8737,#8738,#8739,#8740,#8741,#8742,#8743,#8744,#8745,
#8746,#8747,#8748,#8749,#8750,#8751,#8752,#8753,#8754,#8755,#8756,#8757,
#8758,#8759,#8760,#8761,#8762,#8763,#8764,#8765,#8766,#8767,#8768,#8769,
#8770,#8771,#8772,#8773,#8774,#8775,#8776,#8777,#8778,#8779,#8780,#8781,
#8782,#8783,#8784,#8785,#8786,#8787,#8788,#8789,#8790,#8791,#8792,#8793,
#8794,#8795,#8796,#8797,#8798,#8799,#8800,#8801,#8802,#8803,#8804,#8805,
#8806,#8807,#8808,#8809,#8810,#8811,#8812,#8813,#8814,#8815,#8816,#8817,
#8818,#8819,#8820,#8821,#8822,#8823,#8824,#8825,#8826,#8827,#8828,#8829,
#8830,#8831,#8832,#8833,#8834,#8835,#8836,#8837,#8838,#8839,#8840,#8841,
#8842,#8843,#8844,#8845,#8846,#8847,#8848,#8849,#8850,#8851,#8852,#8853,
#8854,#8855,#8856,#8857,#8858,#8859,#8860,#8861,#8862,#8863,#8864,#8865,
#8866,#8867,#8868,#8869,#8870,#8871,#8872));
#2177=EDGE_LOOP('',(#8873));
#2178=EDGE_LOOP('',(#8874,#8875,#8876,#8877,#8878,#8879,#8880,#8881,#8882,
#8883,#8884,#8885,#8886,#8887,#8888,#8889,#8890,#8891,#8892,#8893,#8894,
#8895,#8896,#8897,#8898,#8899,#8900,#8901,#8902,#8903,#8904,#8905,#8906,
#8907,#8908,#8909,#8910,#8911,#8912,#8913,#8914,#8915,#8916,#8917,#8918,
#8919,#8920,#8921,#8922,#8923,#8924,#8925,#8926,#8927,#8928,#8929,#8930,
#8931,#8932,#8933,#8934,#8935,#8936,#8937,#8938,#8939,#8940,#8941,#8942,
#8943,#8944,#8945,#8946,#8947,#8948,#8949,#8950,#8951,#8952,#8953,#8954,
#8955,#8956,#8957,#8958,#8959,#8960,#8961,#8962,#8963,#8964,#8965,#8966,
#8967,#8968,#8969,#8970,#8971,#8972,#8973,#8974,#8975,#8976,#8977,#8978,
#8979,#8980,#8981,#8982,#8983,#8984,#8985,#8986,#8987,#8988,#8989,#8990,
#8991,#8992,#8993,#8994,#8995,#8996,#8997,#8998,#8999,#9000,#9001,#9002,
#9003,#9004,#9005,#9006,#9007,#9008,#9009,#9010,#9011,#9012,#9013,#9014,
#9015,#9016,#9017,#9018,#9019,#9020,#9021,#9022,#9023,#9024,#9025,#9026,
#9027,#9028,#9029,#9030,#9031,#9032,#9033));
#2179=EDGE_LOOP('',(#9034));
#2180=EDGE_LOOP('',(#9035,#9036,#9037,#9038));
#2181=EDGE_LOOP('',(#9039,#9040,#9041,#9042));
#2182=EDGE_LOOP('',(#9043,#9044,#9045,#9046));
#2183=EDGE_LOOP('',(#9047,#9048,#9049,#9050));
#2184=EDGE_LOOP('',(#9051,#9052,#9053,#9054));
#2185=EDGE_LOOP('',(#9055,#9056,#9057,#9058));
#2186=EDGE_LOOP('',(#9059,#9060,#9061,#9062));
#2187=EDGE_LOOP('',(#9063,#9064,#9065,#9066));
#2188=EDGE_LOOP('',(#9067,#9068,#9069,#9070));
#2189=EDGE_LOOP('',(#9071,#9072,#9073,#9074));
#2190=EDGE_LOOP('',(#9075,#9076,#9077,#9078));
#2191=EDGE_LOOP('',(#9079,#9080,#9081,#9082));
#2192=EDGE_LOOP('',(#9083,#9084,#9085,#9086));
#2193=EDGE_LOOP('',(#9087,#9088,#9089,#9090));
#2194=EDGE_LOOP('',(#9091,#9092,#9093,#9094));
#2195=EDGE_LOOP('',(#9095,#9096,#9097,#9098));
#2196=EDGE_LOOP('',(#9099,#9100,#9101,#9102));
#2197=EDGE_LOOP('',(#9103,#9104,#9105,#9106));
#2198=EDGE_LOOP('',(#9107,#9108,#9109,#9110));
#2199=EDGE_LOOP('',(#9111,#9112,#9113,#9114));
#2200=EDGE_LOOP('',(#9115,#9116,#9117,#9118));
#2201=EDGE_LOOP('',(#9119,#9120,#9121,#9122));
#2202=EDGE_LOOP('',(#9123,#9124,#9125,#9126));
#2203=EDGE_LOOP('',(#9127,#9128,#9129,#9130));
#2204=EDGE_LOOP('',(#9131,#9132,#9133,#9134));
#2205=EDGE_LOOP('',(#9135,#9136,#9137,#9138));
#2206=EDGE_LOOP('',(#9139,#9140,#9141,#9142));
#3003=LINE('',#18825,#3451);
#3004=LINE('',#18831,#3452);
#3005=LINE('',#18840,#3453);
#3006=LINE('',#18843,#3454);
#3007=LINE('',#18846,#3455);
#3008=LINE('',#18848,#3456);
#3009=LINE('',#18849,#3457);
#3010=LINE('',#18855,#3458);
#3011=LINE('',#18858,#3459);
#3012=LINE('',#18861,#3460);
#3013=LINE('',#18863,#3461);
#3014=LINE('',#18864,#3462);
#3015=LINE('',#18870,#3463);
#3016=LINE('',#18873,#3464);
#3017=LINE('',#18876,#3465);
#3018=LINE('',#18878,#3466);
#3019=LINE('',#18879,#3467);
#3020=LINE('',#18885,#3468);
#3021=LINE('',#18888,#3469);
#3022=LINE('',#18891,#3470);
#3023=LINE('',#18893,#3471);
#3024=LINE('',#18894,#3472);
#3025=LINE('',#18900,#3473);
#3026=LINE('',#18903,#3474);
#3027=LINE('',#18906,#3475);
#3028=LINE('',#18908,#3476);
#3029=LINE('',#18909,#3477);
#3030=LINE('',#18915,#3478);
#3031=LINE('',#18918,#3479);
#3032=LINE('',#18921,#3480);
#3033=LINE('',#18923,#3481);
#3034=LINE('',#18924,#3482);
#3035=LINE('',#18930,#3483);
#3036=LINE('',#18933,#3484);
#3037=LINE('',#18936,#3485);
#3038=LINE('',#18938,#3486);
#3039=LINE('',#18939,#3487);
#3040=LINE('',#18945,#3488);
#3041=LINE('',#18948,#3489);
#3042=LINE('',#18951,#3490);
#3043=LINE('',#18953,#3491);
#3044=LINE('',#18954,#3492);
#3045=LINE('',#18960,#3493);
#3046=LINE('',#18963,#3494);
#3047=LINE('',#18966,#3495);
#3048=LINE('',#18968,#3496);
#3049=LINE('',#18969,#3497);
#3050=LINE('',#18975,#3498);
#3051=LINE('',#18978,#3499);
#3052=LINE('',#18981,#3500);
#3053=LINE('',#18983,#3501);
#3054=LINE('',#18984,#3502);
#3055=LINE('',#18990,#3503);
#3056=LINE('',#18993,#3504);
#3057=LINE('',#18996,#3505);
#3058=LINE('',#18998,#3506);
#3059=LINE('',#18999,#3507);
#3060=LINE('',#19005,#3508);
#3061=LINE('',#19008,#3509);
#3062=LINE('',#19011,#3510);
#3063=LINE('',#19013,#3511);
#3064=LINE('',#19014,#3512);
#3065=LINE('',#19020,#3513);
#3066=LINE('',#19023,#3514);
#3067=LINE('',#19026,#3515);
#3068=LINE('',#19028,#3516);
#3069=LINE('',#19029,#3517);
#3070=LINE('',#19035,#3518);
#3071=LINE('',#19038,#3519);
#3072=LINE('',#19041,#3520);
#3073=LINE('',#19043,#3521);
#3074=LINE('',#19044,#3522);
#3075=LINE('',#19050,#3523);
#3076=LINE('',#19053,#3524);
#3077=LINE('',#19056,#3525);
#3078=LINE('',#19058,#3526);
#3079=LINE('',#19059,#3527);
#3080=LINE('',#19065,#3528);
#3081=LINE('',#19068,#3529);
#3082=LINE('',#19071,#3530);
#3083=LINE('',#19073,#3531);
#3084=LINE('',#19074,#3532);
#3085=LINE('',#19080,#3533);
#3086=LINE('',#19083,#3534);
#3087=LINE('',#19086,#3535);
#3088=LINE('',#19088,#3536);
#3089=LINE('',#19089,#3537);
#3090=LINE('',#19095,#3538);
#3091=LINE('',#19098,#3539);
#3092=LINE('',#19101,#3540);
#3093=LINE('',#19103,#3541);
#3094=LINE('',#19104,#3542);
#3095=LINE('',#19110,#3543);
#3096=LINE('',#19113,#3544);
#3097=LINE('',#19116,#3545);
#3098=LINE('',#19118,#3546);
#3099=LINE('',#19119,#3547);
#3100=LINE('',#19125,#3548);
#3101=LINE('',#19128,#3549);
#3102=LINE('',#19131,#3550);
#3103=LINE('',#19133,#3551);
#3104=LINE('',#19134,#3552);
#3105=LINE('',#19140,#3553);
#3106=LINE('',#19143,#3554);
#3107=LINE('',#19146,#3555);
#3108=LINE('',#19148,#3556);
#3109=LINE('',#19149,#3557);
#3110=LINE('',#19155,#3558);
#3111=LINE('',#19158,#3559);
#3112=LINE('',#19161,#3560);
#3113=LINE('',#19163,#3561);
#3114=LINE('',#19164,#3562);
#3115=LINE('',#19170,#3563);
#3116=LINE('',#19173,#3564);
#3117=LINE('',#19176,#3565);
#3118=LINE('',#19178,#3566);
#3119=LINE('',#19179,#3567);
#3120=LINE('',#19185,#3568);
#3121=LINE('',#19188,#3569);
#3122=LINE('',#19191,#3570);
#3123=LINE('',#19193,#3571);
#3124=LINE('',#19194,#3572);
#3125=LINE('',#19200,#3573);
#3126=LINE('',#19203,#3574);
#3127=LINE('',#19206,#3575);
#3128=LINE('',#19208,#3576);
#3129=LINE('',#19209,#3577);
#3130=LINE('',#19215,#3578);
#3131=LINE('',#19218,#3579);
#3132=LINE('',#19221,#3580);
#3133=LINE('',#19223,#3581);
#3134=LINE('',#19224,#3582);
#3135=LINE('',#19230,#3583);
#3136=LINE('',#19233,#3584);
#3137=LINE('',#19236,#3585);
#3138=LINE('',#19238,#3586);
#3139=LINE('',#19239,#3587);
#3140=LINE('',#19245,#3588);
#3141=LINE('',#19248,#3589);
#3142=LINE('',#19251,#3590);
#3143=LINE('',#19253,#3591);
#3144=LINE('',#19254,#3592);
#3145=LINE('',#19260,#3593);
#3146=LINE('',#19263,#3594);
#3147=LINE('',#19266,#3595);
#3148=LINE('',#19268,#3596);
#3149=LINE('',#19269,#3597);
#3150=LINE('',#19275,#3598);
#3151=LINE('',#19278,#3599);
#3152=LINE('',#19281,#3600);
#3153=LINE('',#19283,#3601);
#3154=LINE('',#19284,#3602);
#3155=LINE('',#19290,#3603);
#3156=LINE('',#19293,#3604);
#3157=LINE('',#19296,#3605);
#3158=LINE('',#19298,#3606);
#3159=LINE('',#19299,#3607);
#3160=LINE('',#19305,#3608);
#3161=LINE('',#19308,#3609);
#3162=LINE('',#19311,#3610);
#3163=LINE('',#19313,#3611);
#3164=LINE('',#19314,#3612);
#3165=LINE('',#19320,#3613);
#3166=LINE('',#19323,#3614);
#3167=LINE('',#19326,#3615);
#3168=LINE('',#19328,#3616);
#3169=LINE('',#19329,#3617);
#3170=LINE('',#19335,#3618);
#3171=LINE('',#19338,#3619);
#3172=LINE('',#19341,#3620);
#3173=LINE('',#19343,#3621);
#3174=LINE('',#19344,#3622);
#3175=LINE('',#19350,#3623);
#3176=LINE('',#19353,#3624);
#3177=LINE('',#19356,#3625);
#3178=LINE('',#19358,#3626);
#3179=LINE('',#19359,#3627);
#3180=LINE('',#19365,#3628);
#3181=LINE('',#19368,#3629);
#3182=LINE('',#19371,#3630);
#3183=LINE('',#19373,#3631);
#3184=LINE('',#19374,#3632);
#3185=LINE('',#19380,#3633);
#3186=LINE('',#19383,#3634);
#3187=LINE('',#19386,#3635);
#3188=LINE('',#19388,#3636);
#3189=LINE('',#19389,#3637);
#3190=LINE('',#19395,#3638);
#3191=LINE('',#19398,#3639);
#3192=LINE('',#19401,#3640);
#3193=LINE('',#19403,#3641);
#3194=LINE('',#19404,#3642);
#3195=LINE('',#19706,#3643);
#3196=LINE('',#19712,#3644);
#3197=LINE('',#20312,#3645);
#3198=LINE('',#20318,#3646);
#3199=LINE('',#20918,#3647);
#3200=LINE('',#20924,#3648);
#3201=LINE('',#21524,#3649);
#3202=LINE('',#21530,#3650);
#3203=LINE('',#22130,#3651);
#3204=LINE('',#22136,#3652);
#3205=LINE('',#22736,#3653);
#3206=LINE('',#22742,#3654);
#3207=LINE('',#23342,#3655);
#3208=LINE('',#23348,#3656);
#3209=LINE('',#23948,#3657);
#3210=LINE('',#23954,#3658);
#3211=LINE('',#24554,#3659);
#3212=LINE('',#24560,#3660);
#3213=LINE('',#25160,#3661);
#3214=LINE('',#25166,#3662);
#3215=LINE('',#25766,#3663);
#3216=LINE('',#25772,#3664);
#3217=LINE('',#26372,#3665);
#3218=LINE('',#26378,#3666);
#3219=LINE('',#26978,#3667);
#3220=LINE('',#26984,#3668);
#3221=LINE('',#27584,#3669);
#3222=LINE('',#27590,#3670);
#3223=LINE('',#28190,#3671);
#3224=LINE('',#28196,#3672);
#3225=LINE('',#28796,#3673);
#3226=LINE('',#28802,#3674);
#3227=LINE('',#29402,#3675);
#3228=LINE('',#29408,#3676);
#3229=LINE('',#30008,#3677);
#3230=LINE('',#30014,#3678);
#3231=LINE('',#30614,#3679);
#3232=LINE('',#30620,#3680);
#3233=LINE('',#30942,#3681);
#3234=LINE('',#31096,#3682);
#3235=LINE('',#31107,#3683);
#3236=LINE('',#31262,#3684);
#3237=LINE('',#31285,#3685);
#3238=LINE('',#31305,#3686);
#3239=LINE('',#31307,#3687);
#3240=LINE('',#31309,#3688);
#3241=LINE('',#31310,#3689);
#3242=LINE('',#31312,#3690);
#3243=LINE('',#31463,#3691);
#3244=LINE('',#31465,#3692);
#3451=VECTOR('',#14921,7.5);
#3452=VECTOR('',#14928,7.5);
#3453=VECTOR('',#14939,10.);
#3454=VECTOR('',#14942,10.);
#3455=VECTOR('',#14945,10.);
#3456=VECTOR('',#14946,10.);
#3457=VECTOR('',#14947,10.);
#3458=VECTOR('',#14952,10.);
#3459=VECTOR('',#14955,10.);
#3460=VECTOR('',#14958,10.);
#3461=VECTOR('',#14959,10.);
#3462=VECTOR('',#14960,10.);
#3463=VECTOR('',#14965,10.);
#3464=VECTOR('',#14968,10.);
#3465=VECTOR('',#14971,10.);
#3466=VECTOR('',#14972,10.);
#3467=VECTOR('',#14973,10.);
#3468=VECTOR('',#14978,10.);
#3469=VECTOR('',#14981,10.);
#3470=VECTOR('',#14984,10.);
#3471=VECTOR('',#14985,10.);
#3472=VECTOR('',#14986,10.);
#3473=VECTOR('',#14991,10.);
#3474=VECTOR('',#14994,10.);
#3475=VECTOR('',#14997,10.);
#3476=VECTOR('',#14998,10.);
#3477=VECTOR('',#14999,10.);
#3478=VECTOR('',#15004,10.);
#3479=VECTOR('',#15007,10.);
#3480=VECTOR('',#15010,10.);
#3481=VECTOR('',#15011,10.);
#3482=VECTOR('',#15012,10.);
#3483=VECTOR('',#15017,10.);
#3484=VECTOR('',#15020,10.);
#3485=VECTOR('',#15023,10.);
#3486=VECTOR('',#15024,10.);
#3487=VECTOR('',#15025,10.);
#3488=VECTOR('',#15030,10.);
#3489=VECTOR('',#15033,10.);
#3490=VECTOR('',#15036,10.);
#3491=VECTOR('',#15037,10.);
#3492=VECTOR('',#15038,10.);
#3493=VECTOR('',#15043,10.);
#3494=VECTOR('',#15046,10.);
#3495=VECTOR('',#15049,10.);
#3496=VECTOR('',#15050,10.);
#3497=VECTOR('',#15051,10.);
#3498=VECTOR('',#15056,10.);
#3499=VECTOR('',#15059,10.);
#3500=VECTOR('',#15062,10.);
#3501=VECTOR('',#15063,10.);
#3502=VECTOR('',#15064,10.);
#3503=VECTOR('',#15069,10.);
#3504=VECTOR('',#15072,10.);
#3505=VECTOR('',#15075,10.);
#3506=VECTOR('',#15076,10.);
#3507=VECTOR('',#15077,10.);
#3508=VECTOR('',#15082,10.);
#3509=VECTOR('',#15085,10.);
#3510=VECTOR('',#15088,10.);
#3511=VECTOR('',#15089,10.);
#3512=VECTOR('',#15090,10.);
#3513=VECTOR('',#15095,10.);
#3514=VECTOR('',#15098,10.);
#3515=VECTOR('',#15101,10.);
#3516=VECTOR('',#15102,10.);
#3517=VECTOR('',#15103,10.);
#3518=VECTOR('',#15108,10.);
#3519=VECTOR('',#15111,10.);
#3520=VECTOR('',#15114,10.);
#3521=VECTOR('',#15115,10.);
#3522=VECTOR('',#15116,10.);
#3523=VECTOR('',#15121,10.);
#3524=VECTOR('',#15124,10.);
#3525=VECTOR('',#15127,10.);
#3526=VECTOR('',#15128,10.);
#3527=VECTOR('',#15129,10.);
#3528=VECTOR('',#15134,10.);
#3529=VECTOR('',#15137,10.);
#3530=VECTOR('',#15140,10.);
#3531=VECTOR('',#15141,10.);
#3532=VECTOR('',#15142,10.);
#3533=VECTOR('',#15147,10.);
#3534=VECTOR('',#15150,10.);
#3535=VECTOR('',#15153,10.);
#3536=VECTOR('',#15154,10.);
#3537=VECTOR('',#15155,10.);
#3538=VECTOR('',#15160,10.);
#3539=VECTOR('',#15163,10.);
#3540=VECTOR('',#15166,10.);
#3541=VECTOR('',#15167,10.);
#3542=VECTOR('',#15168,10.);
#3543=VECTOR('',#15173,10.);
#3544=VECTOR('',#15176,10.);
#3545=VECTOR('',#15179,10.);
#3546=VECTOR('',#15180,10.);
#3547=VECTOR('',#15181,10.);
#3548=VECTOR('',#15186,10.);
#3549=VECTOR('',#15189,10.);
#3550=VECTOR('',#15192,10.);
#3551=VECTOR('',#15193,10.);
#3552=VECTOR('',#15194,10.);
#3553=VECTOR('',#15199,10.);
#3554=VECTOR('',#15202,10.);
#3555=VECTOR('',#15205,10.);
#3556=VECTOR('',#15206,10.);
#3557=VECTOR('',#15207,10.);
#3558=VECTOR('',#15212,10.);
#3559=VECTOR('',#15215,10.);
#3560=VECTOR('',#15218,10.);
#3561=VECTOR('',#15219,10.);
#3562=VECTOR('',#15220,10.);
#3563=VECTOR('',#15225,10.);
#3564=VECTOR('',#15228,10.);
#3565=VECTOR('',#15231,10.);
#3566=VECTOR('',#15232,10.);
#3567=VECTOR('',#15233,10.);
#3568=VECTOR('',#15238,10.);
#3569=VECTOR('',#15241,10.);
#3570=VECTOR('',#15244,10.);
#3571=VECTOR('',#15245,10.);
#3572=VECTOR('',#15246,10.);
#3573=VECTOR('',#15251,10.);
#3574=VECTOR('',#15254,10.);
#3575=VECTOR('',#15257,10.);
#3576=VECTOR('',#15258,10.);
#3577=VECTOR('',#15259,10.);
#3578=VECTOR('',#15264,10.);
#3579=VECTOR('',#15267,10.);
#3580=VECTOR('',#15270,10.);
#3581=VECTOR('',#15271,10.);
#3582=VECTOR('',#15272,10.);
#3583=VECTOR('',#15277,10.);
#3584=VECTOR('',#15280,10.);
#3585=VECTOR('',#15283,10.);
#3586=VECTOR('',#15284,10.);
#3587=VECTOR('',#15285,10.);
#3588=VECTOR('',#15290,10.);
#3589=VECTOR('',#15293,10.);
#3590=VECTOR('',#15296,10.);
#3591=VECTOR('',#15297,10.);
#3592=VECTOR('',#15298,10.);
#3593=VECTOR('',#15303,10.);
#3594=VECTOR('',#15306,10.);
#3595=VECTOR('',#15309,10.);
#3596=VECTOR('',#15310,10.);
#3597=VECTOR('',#15311,10.);
#3598=VECTOR('',#15316,10.);
#3599=VECTOR('',#15319,10.);
#3600=VECTOR('',#15322,10.);
#3601=VECTOR('',#15323,10.);
#3602=VECTOR('',#15324,10.);
#3603=VECTOR('',#15329,10.);
#3604=VECTOR('',#15332,10.);
#3605=VECTOR('',#15335,10.);
#3606=VECTOR('',#15336,10.);
#3607=VECTOR('',#15337,10.);
#3608=VECTOR('',#15342,10.);
#3609=VECTOR('',#15345,10.);
#3610=VECTOR('',#15348,10.);
#3611=VECTOR('',#15349,10.);
#3612=VECTOR('',#15350,10.);
#3613=VECTOR('',#15355,10.);
#3614=VECTOR('',#15358,10.);
#3615=VECTOR('',#15361,10.);
#3616=VECTOR('',#15362,10.);
#3617=VECTOR('',#15363,10.);
#3618=VECTOR('',#15368,10.);
#3619=VECTOR('',#15371,10.);
#3620=VECTOR('',#15374,10.);
#3621=VECTOR('',#15375,10.);
#3622=VECTOR('',#15376,10.);
#3623=VECTOR('',#15381,10.);
#3624=VECTOR('',#15384,10.);
#3625=VECTOR('',#15387,10.);
#3626=VECTOR('',#15388,10.);
#3627=VECTOR('',#15389,10.);
#3628=VECTOR('',#15394,10.);
#3629=VECTOR('',#15397,10.);
#3630=VECTOR('',#15400,10.);
#3631=VECTOR('',#15401,10.);
#3632=VECTOR('',#15402,10.);
#3633=VECTOR('',#15407,10.);
#3634=VECTOR('',#15410,10.);
#3635=VECTOR('',#15413,10.);
#3636=VECTOR('',#15414,10.);
#3637=VECTOR('',#15415,10.);
#3638=VECTOR('',#15420,10.);
#3639=VECTOR('',#15423,10.);
#3640=VECTOR('',#15426,10.);
#3641=VECTOR('',#15427,10.);
#3642=VECTOR('',#15428,10.);
#3643=VECTOR('',#15429,10.);
#3644=VECTOR('',#15436,10.);
#3645=VECTOR('',#15437,10.);
#3646=VECTOR('',#15444,10.);
#3647=VECTOR('',#15445,10.);
#3648=VECTOR('',#15452,10.);
#3649=VECTOR('',#15453,10.);
#3650=VECTOR('',#15460,10.);
#3651=VECTOR('',#15461,10.);
#3652=VECTOR('',#15468,10.);
#3653=VECTOR('',#15469,10.);
#3654=VECTOR('',#15476,10.);
#3655=VECTOR('',#15477,10.);
#3656=VECTOR('',#15484,10.);
#3657=VECTOR('',#15485,10.);
#3658=VECTOR('',#15492,10.);
#3659=VECTOR('',#15493,10.);
#3660=VECTOR('',#15500,10.);
#3661=VECTOR('',#15501,10.);
#3662=VECTOR('',#15508,10.);
#3663=VECTOR('',#15509,10.);
#3664=VECTOR('',#15516,10.);
#3665=VECTOR('',#15517,10.);
#3666=VECTOR('',#15524,10.);
#3667=VECTOR('',#15525,10.);
#3668=VECTOR('',#15532,10.);
#3669=VECTOR('',#15533,10.);
#3670=VECTOR('',#15540,10.);
#3671=VECTOR('',#15541,10.);
#3672=VECTOR('',#15548,10.);
#3673=VECTOR('',#15549,10.);
#3674=VECTOR('',#15556,10.);
#3675=VECTOR('',#15557,10.);
#3676=VECTOR('',#15564,10.);
#3677=VECTOR('',#15565,10.);
#3678=VECTOR('',#15572,10.);
#3679=VECTOR('',#15573,10.);
#3680=VECTOR('',#15580,10.);
#3681=VECTOR('',#15621,10.);
#3682=VECTOR('',#15624,10.);
#3683=VECTOR('',#15637,10.);
#3684=VECTOR('',#15640,10.);
#3685=VECTOR('',#15683,10.);
#3686=VECTOR('',#15722,10.);
#3687=VECTOR('',#15725,10.);
#3688=VECTOR('',#15728,10.);
#3689=VECTOR('',#15729,10.);
#3690=VECTOR('',#15732,10.);
#3691=VECTOR('',#15733,10.);
#3692=VECTOR('',#15736,10.);
#3899=CIRCLE('',#13187,7.5);
#3900=CIRCLE('',#13188,7.5);
#3901=CIRCLE('',#13190,7.5);
#3902=CIRCLE('',#13191,7.5);
#3903=CIRCLE('',#13195,1.);
#3904=CIRCLE('',#13196,1.);
#3905=CIRCLE('',#13199,1.);
#3906=CIRCLE('',#13200,1.);
#3907=CIRCLE('',#13203,1.);
#3908=CIRCLE('',#13204,1.);
#3909=CIRCLE('',#13207,1.);
#3910=CIRCLE('',#13208,1.);
#3911=CIRCLE('',#13211,1.);
#3912=CIRCLE('',#13212,1.);
#3913=CIRCLE('',#13215,1.);
#3914=CIRCLE('',#13216,1.);
#3915=CIRCLE('',#13219,1.);
#3916=CIRCLE('',#13220,1.);
#3917=CIRCLE('',#13223,1.);
#3918=CIRCLE('',#13224,1.);
#3919=CIRCLE('',#13227,1.);
#3920=CIRCLE('',#13228,1.);
#3921=CIRCLE('',#13231,1.);
#3922=CIRCLE('',#13232,1.);
#3923=CIRCLE('',#13235,1.);
#3924=CIRCLE('',#13236,1.);
#3925=CIRCLE('',#13239,1.);
#3926=CIRCLE('',#13240,1.);
#3927=CIRCLE('',#13243,1.);
#3928=CIRCLE('',#13244,1.);
#3929=CIRCLE('',#13247,1.);
#3930=CIRCLE('',#13248,1.);
#3931=CIRCLE('',#13251,1.);
#3932=CIRCLE('',#13252,1.);
#3933=CIRCLE('',#13255,1.);
#3934=CIRCLE('',#13256,1.);
#3935=CIRCLE('',#13259,1.);
#3936=CIRCLE('',#13260,1.);
#3937=CIRCLE('',#13263,1.);
#3938=CIRCLE('',#13264,1.);
#3939=CIRCLE('',#13267,1.);
#3940=CIRCLE('',#13268,1.);
#3941=CIRCLE('',#13271,1.);
#3942=CIRCLE('',#13272,1.);
#3943=CIRCLE('',#13275,1.);
#3944=CIRCLE('',#13276,1.);
#3945=CIRCLE('',#13279,1.);
#3946=CIRCLE('',#13280,1.);
#3947=CIRCLE('',#13283,1.);
#3948=CIRCLE('',#13284,1.);
#3949=CIRCLE('',#13287,1.);
#3950=CIRCLE('',#13288,1.);
#3951=CIRCLE('',#13291,1.);
#3952=CIRCLE('',#13292,1.);
#3953=CIRCLE('',#13295,1.);
#3954=CIRCLE('',#13296,1.);
#3955=CIRCLE('',#13299,1.);
#3956=CIRCLE('',#13300,1.);
#3957=CIRCLE('',#13303,1.);
#3958=CIRCLE('',#13304,1.);
#3959=CIRCLE('',#13307,1.);
#3960=CIRCLE('',#13308,1.);
#3961=CIRCLE('',#13311,1.);
#3962=CIRCLE('',#13312,1.);
#3963=CIRCLE('',#13315,1.);
#3964=CIRCLE('',#13316,1.);
#3965=CIRCLE('',#13319,1.);
#3966=CIRCLE('',#13320,1.);
#3967=CIRCLE('',#13323,1.);
#3968=CIRCLE('',#13324,1.);
#3969=CIRCLE('',#13327,1.);
#3970=CIRCLE('',#13328,1.);
#3971=CIRCLE('',#13331,1.);
#3972=CIRCLE('',#13332,1.);
#3973=CIRCLE('',#13335,1.);
#3974=CIRCLE('',#13336,1.);
#3975=CIRCLE('',#13339,1.);
#3976=CIRCLE('',#13340,1.);
#3977=CIRCLE('',#13343,1.);
#3978=CIRCLE('',#13344,1.);
#3979=CIRCLE('',#13347,43.9999999999887);
#3980=CIRCLE('',#13348,43.9999999999887);
#3981=CIRCLE('',#13350,43.9999999999887);
#3982=CIRCLE('',#13351,43.9999999999887);
#3983=CIRCLE('',#13353,43.9999999999887);
#3984=CIRCLE('',#13354,43.9999999999887);
#3985=CIRCLE('',#13356,43.9999999999887);
#3986=CIRCLE('',#13357,43.9999999999887);
#3987=CIRCLE('',#13359,43.9999999999887);
#3988=CIRCLE('',#13360,43.9999999999887);
#3989=CIRCLE('',#13362,43.9999999999887);
#3990=CIRCLE('',#13363,43.9999999999887);
#3991=CIRCLE('',#13365,43.9999999999887);
#3992=CIRCLE('',#13366,43.9999999999887);
#3993=CIRCLE('',#13368,43.9999999999887);
#3994=CIRCLE('',#13369,43.9999999999887);
#3995=CIRCLE('',#13371,43.9999999999887);
#3996=CIRCLE('',#13372,43.9999999999887);
#3997=CIRCLE('',#13374,43.9999999999887);
#3998=CIRCLE('',#13375,43.9999999999887);
#3999=CIRCLE('',#13377,43.9999999999887);
#4000=CIRCLE('',#13378,43.9999999999887);
#4001=CIRCLE('',#13380,43.9999999999887);
#4002=CIRCLE('',#13381,43.9999999999887);
#4003=CIRCLE('',#13383,43.9999999999887);
#4004=CIRCLE('',#13384,43.9999999999887);
#4005=CIRCLE('',#13386,43.9999999999887);
#4006=CIRCLE('',#13387,43.9999999999887);
#4007=CIRCLE('',#13389,43.9999999999887);
#4008=CIRCLE('',#13390,43.9999999999887);
#4009=CIRCLE('',#13392,43.9999999999887);
#4010=CIRCLE('',#13393,43.9999999999887);
#4011=CIRCLE('',#13395,43.9999999999887);
#4012=CIRCLE('',#13396,43.9999999999887);
#4013=CIRCLE('',#13398,43.9999999999887);
#4014=CIRCLE('',#13399,43.9999999999887);
#4015=CIRCLE('',#13401,43.9999999999887);
#4016=CIRCLE('',#13402,43.9999999999887);
#4017=CIRCLE('',#13404,35.372);
#4018=CIRCLE('',#13405,35.372);
#4019=CIRCLE('',#13406,35.372);
#4020=CIRCLE('',#13407,35.372);
#4021=CIRCLE('',#13408,35.372);
#4022=CIRCLE('',#13409,35.372);
#4023=CIRCLE('',#13410,35.372);
#4024=CIRCLE('',#13411,35.372);
#4025=CIRCLE('',#13412,35.372);
#4026=CIRCLE('',#13413,35.372);
#4027=CIRCLE('',#13414,35.372);
#4028=CIRCLE('',#13415,35.372);
#4029=CIRCLE('',#13416,35.372);
#4030=CIRCLE('',#13417,35.372);
#4031=CIRCLE('',#13418,35.372);
#4032=CIRCLE('',#13419,35.372);
#4033=CIRCLE('',#13420,35.372);
#4034=CIRCLE('',#13421,35.372);
#4035=CIRCLE('',#13422,1.);
#4036=CIRCLE('',#13423,43.9999999999887);
#4037=CIRCLE('',#13424,1.);
#4038=CIRCLE('',#13425,35.372);
#4039=CIRCLE('',#13426,35.372);
#4040=CIRCLE('',#13428,35.372);
#4041=CIRCLE('',#13429,1.);
#4042=CIRCLE('',#13430,43.9999999999887);
#4043=CIRCLE('',#13431,1.);
#4044=CIRCLE('',#13432,35.372);
#4045=CIRCLE('',#13433,35.372);
#4046=CIRCLE('',#13434,35.372);
#4047=CIRCLE('',#13435,35.372);
#4048=CIRCLE('',#13436,35.372);
#4049=CIRCLE('',#13437,35.372);
#4050=CIRCLE('',#13438,35.372);
#4051=CIRCLE('',#13439,35.372);
#4052=CIRCLE('',#13440,35.372);
#4053=CIRCLE('',#13441,35.372);
#4054=CIRCLE('',#13442,35.372);
#4055=CIRCLE('',#13443,35.372);
#4056=CIRCLE('',#13444,35.372);
#4057=CIRCLE('',#13445,35.372);
#4058=CIRCLE('',#13446,35.372);
#4059=CIRCLE('',#13447,35.372);
#4060=CIRCLE('',#13448,35.372);
#4061=CIRCLE('',#13449,35.372);
#4062=CIRCLE('',#13450,35.372);
#4919=VERTEX_POINT('',#18822);
#4920=VERTEX_POINT('',#18824);
#4921=VERTEX_POINT('',#18828);
#4922=VERTEX_POINT('',#18830);
#4923=VERTEX_POINT('',#18836);
#4924=VERTEX_POINT('',#18837);
#4925=VERTEX_POINT('',#18839);
#4926=VERTEX_POINT('',#18841);
#4927=VERTEX_POINT('',#18845);
#4928=VERTEX_POINT('',#18847);
#4929=VERTEX_POINT('',#18851);
#4930=VERTEX_POINT('',#18852);
#4931=VERTEX_POINT('',#18854);
#4932=VERTEX_POINT('',#18856);
#4933=VERTEX_POINT('',#18860);
#4934=VERTEX_POINT('',#18862);
#4935=VERTEX_POINT('',#18866);
#4936=VERTEX_POINT('',#18867);
#4937=VERTEX_POINT('',#18869);
#4938=VERTEX_POINT('',#18871);
#4939=VERTEX_POINT('',#18875);
#4940=VERTEX_POINT('',#18877);
#4941=VERTEX_POINT('',#18881);
#4942=VERTEX_POINT('',#18882);
#4943=VERTEX_POINT('',#18884);
#4944=VERTEX_POINT('',#18886);
#4945=VERTEX_POINT('',#18890);
#4946=VERTEX_POINT('',#18892);
#4947=VERTEX_POINT('',#18896);
#4948=VERTEX_POINT('',#18897);
#4949=VERTEX_POINT('',#18899);
#4950=VERTEX_POINT('',#18901);
#4951=VERTEX_POINT('',#18905);
#4952=VERTEX_POINT('',#18907);
#4953=VERTEX_POINT('',#18911);
#4954=VERTEX_POINT('',#18912);
#4955=VERTEX_POINT('',#18914);
#4956=VERTEX_POINT('',#18916);
#4957=VERTEX_POINT('',#18920);
#4958=VERTEX_POINT('',#18922);
#4959=VERTEX_POINT('',#18926);
#4960=VERTEX_POINT('',#18927);
#4961=VERTEX_POINT('',#18929);
#4962=VERTEX_POINT('',#18931);
#4963=VERTEX_POINT('',#18935);
#4964=VERTEX_POINT('',#18937);
#4965=VERTEX_POINT('',#18941);
#4966=VERTEX_POINT('',#18942);
#4967=VERTEX_POINT('',#18944);
#4968=VERTEX_POINT('',#18946);
#4969=VERTEX_POINT('',#18950);
#4970=VERTEX_POINT('',#18952);
#4971=VERTEX_POINT('',#18956);
#4972=VERTEX_POINT('',#18957);
#4973=VERTEX_POINT('',#18959);
#4974=VERTEX_POINT('',#18961);
#4975=VERTEX_POINT('',#18965);
#4976=VERTEX_POINT('',#18967);
#4977=VERTEX_POINT('',#18971);
#4978=VERTEX_POINT('',#18972);
#4979=VERTEX_POINT('',#18974);
#4980=VERTEX_POINT('',#18976);
#4981=VERTEX_POINT('',#18980);
#4982=VERTEX_POINT('',#18982);
#4983=VERTEX_POINT('',#18986);
#4984=VERTEX_POINT('',#18987);
#4985=VERTEX_POINT('',#18989);
#4986=VERTEX_POINT('',#18991);
#4987=VERTEX_POINT('',#18995);
#4988=VERTEX_POINT('',#18997);
#4989=VERTEX_POINT('',#19001);
#4990=VERTEX_POINT('',#19002);
#4991=VERTEX_POINT('',#19004);
#4992=VERTEX_POINT('',#19006);
#4993=VERTEX_POINT('',#19010);
#4994=VERTEX_POINT('',#19012);
#4995=VERTEX_POINT('',#19016);
#4996=VERTEX_POINT('',#19017);
#4997=VERTEX_POINT('',#19019);
#4998=VERTEX_POINT('',#19021);
#4999=VERTEX_POINT('',#19025);
#5000=VERTEX_POINT('',#19027);
#5001=VERTEX_POINT('',#19031);
#5002=VERTEX_POINT('',#19032);
#5003=VERTEX_POINT('',#19034);
#5004=VERTEX_POINT('',#19036);
#5005=VERTEX_POINT('',#19040);
#5006=VERTEX_POINT('',#19042);
#5007=VERTEX_POINT('',#19046);
#5008=VERTEX_POINT('',#19047);
#5009=VERTEX_POINT('',#19049);
#5010=VERTEX_POINT('',#19051);
#5011=VERTEX_POINT('',#19055);
#5012=VERTEX_POINT('',#19057);
#5013=VERTEX_POINT('',#19061);
#5014=VERTEX_POINT('',#19062);
#5015=VERTEX_POINT('',#19064);
#5016=VERTEX_POINT('',#19066);
#5017=VERTEX_POINT('',#19070);
#5018=VERTEX_POINT('',#19072);
#5019=VERTEX_POINT('',#19076);
#5020=VERTEX_POINT('',#19077);
#5021=VERTEX_POINT('',#19079);
#5022=VERTEX_POINT('',#19081);
#5023=VERTEX_POINT('',#19085);
#5024=VERTEX_POINT('',#19087);
#5025=VERTEX_POINT('',#19091);
#5026=VERTEX_POINT('',#19092);
#5027=VERTEX_POINT('',#19094);
#5028=VERTEX_POINT('',#19096);
#5029=VERTEX_POINT('',#19100);
#5030=VERTEX_POINT('',#19102);
#5031=VERTEX_POINT('',#19106);
#5032=VERTEX_POINT('',#19107);
#5033=VERTEX_POINT('',#19109);
#5034=VERTEX_POINT('',#19111);
#5035=VERTEX_POINT('',#19115);
#5036=VERTEX_POINT('',#19117);
#5037=VERTEX_POINT('',#19121);
#5038=VERTEX_POINT('',#19122);
#5039=VERTEX_POINT('',#19124);
#5040=VERTEX_POINT('',#19126);
#5041=VERTEX_POINT('',#19130);
#5042=VERTEX_POINT('',#19132);
#5043=VERTEX_POINT('',#19136);
#5044=VERTEX_POINT('',#19137);
#5045=VERTEX_POINT('',#19139);
#5046=VERTEX_POINT('',#19141);
#5047=VERTEX_POINT('',#19145);
#5048=VERTEX_POINT('',#19147);
#5049=VERTEX_POINT('',#19151);
#5050=VERTEX_POINT('',#19152);
#5051=VERTEX_POINT('',#19154);
#5052=VERTEX_POINT('',#19156);
#5053=VERTEX_POINT('',#19160);
#5054=VERTEX_POINT('',#19162);
#5055=VERTEX_POINT('',#19166);
#5056=VERTEX_POINT('',#19167);
#5057=VERTEX_POINT('',#19169);
#5058=VERTEX_POINT('',#19171);
#5059=VERTEX_POINT('',#19175);
#5060=VERTEX_POINT('',#19177);
#5061=VERTEX_POINT('',#19181);
#5062=VERTEX_POINT('',#19182);
#5063=VERTEX_POINT('',#19184);
#5064=VERTEX_POINT('',#19186);
#5065=VERTEX_POINT('',#19190);
#5066=VERTEX_POINT('',#19192);
#5067=VERTEX_POINT('',#19196);
#5068=VERTEX_POINT('',#19197);
#5069=VERTEX_POINT('',#19199);
#5070=VERTEX_POINT('',#19201);
#5071=VERTEX_POINT('',#19205);
#5072=VERTEX_POINT('',#19207);
#5073=VERTEX_POINT('',#19211);
#5074=VERTEX_POINT('',#19212);
#5075=VERTEX_POINT('',#19214);
#5076=VERTEX_POINT('',#19216);
#5077=VERTEX_POINT('',#19220);
#5078=VERTEX_POINT('',#19222);
#5079=VERTEX_POINT('',#19226);
#5080=VERTEX_POINT('',#19227);
#5081=VERTEX_POINT('',#19229);
#5082=VERTEX_POINT('',#19231);
#5083=VERTEX_POINT('',#19235);
#5084=VERTEX_POINT('',#19237);
#5085=VERTEX_POINT('',#19241);
#5086=VERTEX_POINT('',#19242);
#5087=VERTEX_POINT('',#19244);
#5088=VERTEX_POINT('',#19246);
#5089=VERTEX_POINT('',#19250);
#5090=VERTEX_POINT('',#19252);
#5091=VERTEX_POINT('',#19256);
#5092=VERTEX_POINT('',#19257);
#5093=VERTEX_POINT('',#19259);
#5094=VERTEX_POINT('',#19261);
#5095=VERTEX_POINT('',#19265);
#5096=VERTEX_POINT('',#19267);
#5097=VERTEX_POINT('',#19271);
#5098=VERTEX_POINT('',#19272);
#5099=VERTEX_POINT('',#19274);
#5100=VERTEX_POINT('',#19276);
#5101=VERTEX_POINT('',#19280);
#5102=VERTEX_POINT('',#19282);
#5103=VERTEX_POINT('',#19286);
#5104=VERTEX_POINT('',#19287);
#5105=VERTEX_POINT('',#19289);
#5106=VERTEX_POINT('',#19291);
#5107=VERTEX_POINT('',#19295);
#5108=VERTEX_POINT('',#19297);
#5109=VERTEX_POINT('',#19301);
#5110=VERTEX_POINT('',#19302);
#5111=VERTEX_POINT('',#19304);
#5112=VERTEX_POINT('',#19306);
#5113=VERTEX_POINT('',#19310);
#5114=VERTEX_POINT('',#19312);
#5115=VERTEX_POINT('',#19316);
#5116=VERTEX_POINT('',#19317);
#5117=VERTEX_POINT('',#19319);
#5118=VERTEX_POINT('',#19321);
#5119=VERTEX_POINT('',#19325);
#5120=VERTEX_POINT('',#19327);
#5121=VERTEX_POINT('',#19331);
#5122=VERTEX_POINT('',#19332);
#5123=VERTEX_POINT('',#19334);
#5124=VERTEX_POINT('',#19336);
#5125=VERTEX_POINT('',#19340);
#5126=VERTEX_POINT('',#19342);
#5127=VERTEX_POINT('',#19346);
#5128=VERTEX_POINT('',#19347);
#5129=VERTEX_POINT('',#19349);
#5130=VERTEX_POINT('',#19351);
#5131=VERTEX_POINT('',#19355);
#5132=VERTEX_POINT('',#19357);
#5133=VERTEX_POINT('',#19361);
#5134=VERTEX_POINT('',#19362);
#5135=VERTEX_POINT('',#19364);
#5136=VERTEX_POINT('',#19366);
#5137=VERTEX_POINT('',#19370);
#5138=VERTEX_POINT('',#19372);
#5139=VERTEX_POINT('',#19376);
#5140=VERTEX_POINT('',#19377);
#5141=VERTEX_POINT('',#19379);
#5142=VERTEX_POINT('',#19381);
#5143=VERTEX_POINT('',#19385);
#5144=VERTEX_POINT('',#19387);
#5145=VERTEX_POINT('',#19391);
#5146=VERTEX_POINT('',#19392);
#5147=VERTEX_POINT('',#19394);
#5148=VERTEX_POINT('',#19396);
#5149=VERTEX_POINT('',#19400);
#5150=VERTEX_POINT('',#19402);
#5151=VERTEX_POINT('',#19555);
#5152=VERTEX_POINT('',#19630);
#5153=VERTEX_POINT('',#19708);
#5154=VERTEX_POINT('',#19710);
#5155=VERTEX_POINT('',#20161);
#5156=VERTEX_POINT('',#20236);
#5157=VERTEX_POINT('',#20314);
#5158=VERTEX_POINT('',#20316);
#5159=VERTEX_POINT('',#20767);
#5160=VERTEX_POINT('',#20842);
#5161=VERTEX_POINT('',#20920);
#5162=VERTEX_POINT('',#20922);
#5163=VERTEX_POINT('',#21373);
#5164=VERTEX_POINT('',#21448);
#5165=VERTEX_POINT('',#21526);
#5166=VERTEX_POINT('',#21528);
#5167=VERTEX_POINT('',#21979);
#5168=VERTEX_POINT('',#22054);
#5169=VERTEX_POINT('',#22132);
#5170=VERTEX_POINT('',#22134);
#5171=VERTEX_POINT('',#22585);
#5172=VERTEX_POINT('',#22660);
#5173=VERTEX_POINT('',#22738);
#5174=VERTEX_POINT('',#22740);
#5175=VERTEX_POINT('',#23191);
#5176=VERTEX_POINT('',#23266);
#5177=VERTEX_POINT('',#23344);
#5178=VERTEX_POINT('',#23346);
#5179=VERTEX_POINT('',#23797);
#5180=VERTEX_POINT('',#23872);
#5181=VERTEX_POINT('',#23950);
#5182=VERTEX_POINT('',#23952);
#5183=VERTEX_POINT('',#24403);
#5184=VERTEX_POINT('',#24478);
#5185=VERTEX_POINT('',#24556);
#5186=VERTEX_POINT('',#24558);
#5187=VERTEX_POINT('',#25009);
#5188=VERTEX_POINT('',#25084);
#5189=VERTEX_POINT('',#25162);
#5190=VERTEX_POINT('',#25164);
#5191=VERTEX_POINT('',#25615);
#5192=VERTEX_POINT('',#25690);
#5193=VERTEX_POINT('',#25768);
#5194=VERTEX_POINT('',#25770);
#5195=VERTEX_POINT('',#26221);
#5196=VERTEX_POINT('',#26296);
#5197=VERTEX_POINT('',#26374);
#5198=VERTEX_POINT('',#26376);
#5199=VERTEX_POINT('',#26827);
#5200=VERTEX_POINT('',#26902);
#5201=VERTEX_POINT('',#26980);
#5202=VERTEX_POINT('',#26982);
#5203=VERTEX_POINT('',#27433);
#5204=VERTEX_POINT('',#27508);
#5205=VERTEX_POINT('',#27586);
#5206=VERTEX_POINT('',#27588);
#5207=VERTEX_POINT('',#28039);
#5208=VERTEX_POINT('',#28114);
#5209=VERTEX_POINT('',#28192);
#5210=VERTEX_POINT('',#28194);
#5211=VERTEX_POINT('',#28645);
#5212=VERTEX_POINT('',#28720);
#5213=VERTEX_POINT('',#28798);
#5214=VERTEX_POINT('',#28800);
#5215=VERTEX_POINT('',#29251);
#5216=VERTEX_POINT('',#29326);
#5217=VERTEX_POINT('',#29404);
#5218=VERTEX_POINT('',#29406);
#5219=VERTEX_POINT('',#29857);
#5220=VERTEX_POINT('',#29932);
#5221=VERTEX_POINT('',#30010);
#5222=VERTEX_POINT('',#30012);
#5223=VERTEX_POINT('',#30463);
#5224=VERTEX_POINT('',#30538);
#5225=VERTEX_POINT('',#30616);
#5226=VERTEX_POINT('',#30618);
#5227=VERTEX_POINT('',#30937);
#5228=VERTEX_POINT('',#30939);
#5229=VERTEX_POINT('',#30941);
#5230=VERTEX_POINT('',#30943);
#5231=VERTEX_POINT('',#31018);
#5232=VERTEX_POINT('',#31020);
#5233=VERTEX_POINT('',#31095);
#5234=VERTEX_POINT('',#31097);
#5235=VERTEX_POINT('',#31102);
#5236=VERTEX_POINT('',#31104);
#5237=VERTEX_POINT('',#31106);
#5238=VERTEX_POINT('',#31108);
#5239=VERTEX_POINT('',#31183);
#5240=VERTEX_POINT('',#31185);
#5241=VERTEX_POINT('',#31261);
#5242=VERTEX_POINT('',#31263);
#6247=EDGE_CURVE('',#4919,#4919,#3899,.T.);
#6248=EDGE_CURVE('',#4919,#4920,#3003,.T.);
#6249=EDGE_CURVE('',#4920,#4920,#3900,.F.);
#6250=EDGE_CURVE('',#4921,#4921,#3901,.T.);
#6251=EDGE_CURVE('',#4921,#4922,#3004,.T.);
#6252=EDGE_CURVE('',#4922,#4922,#3902,.T.);
#6253=EDGE_CURVE('',#4923,#4924,#3903,.T.);
#6254=EDGE_CURVE('',#4924,#4925,#3005,.T.);
#6255=EDGE_CURVE('',#4925,#4926,#3904,.T.);
#6256=EDGE_CURVE('',#4926,#4923,#3006,.T.);
#6257=EDGE_CURVE('',#4927,#4924,#3007,.T.);
#6258=EDGE_CURVE('',#4928,#4927,#3008,.T.);
#6259=EDGE_CURVE('',#4925,#4928,#3009,.T.);
#6260=EDGE_CURVE('',#4929,#4930,#3905,.T.);
#6261=EDGE_CURVE('',#4930,#4931,#3010,.T.);
#6262=EDGE_CURVE('',#4931,#4932,#3906,.T.);
#6263=EDGE_CURVE('',#4932,#4929,#3011,.T.);
#6264=EDGE_CURVE('',#4930,#4933,#3012,.T.);
#6265=EDGE_CURVE('',#4933,#4934,#3013,.T.);
#6266=EDGE_CURVE('',#4931,#4934,#3014,.T.);
#6267=EDGE_CURVE('',#4935,#4936,#3907,.T.);
#6268=EDGE_CURVE('',#4936,#4937,#3015,.T.);
#6269=EDGE_CURVE('',#4937,#4938,#3908,.T.);
#6270=EDGE_CURVE('',#4938,#4935,#3016,.T.);
#6271=EDGE_CURVE('',#4939,#4936,#3017,.T.);
#6272=EDGE_CURVE('',#4940,#4939,#3018,.T.);
#6273=EDGE_CURVE('',#4937,#4940,#3019,.T.);
#6274=EDGE_CURVE('',#4941,#4942,#3909,.T.);
#6275=EDGE_CURVE('',#4942,#4943,#3020,.T.);
#6276=EDGE_CURVE('',#4943,#4944,#3910,.T.);
#6277=EDGE_CURVE('',#4944,#4941,#3021,.T.);
#6278=EDGE_CURVE('',#4942,#4945,#3022,.T.);
#6279=EDGE_CURVE('',#4945,#4946,#3023,.T.);
#6280=EDGE_CURVE('',#4943,#4946,#3024,.T.);
#6281=EDGE_CURVE('',#4947,#4948,#3911,.T.);
#6282=EDGE_CURVE('',#4948,#4949,#3025,.T.);
#6283=EDGE_CURVE('',#4949,#4950,#3912,.T.);
#6284=EDGE_CURVE('',#4950,#4947,#3026,.T.);
#6285=EDGE_CURVE('',#4951,#4948,#3027,.T.);
#6286=EDGE_CURVE('',#4952,#4951,#3028,.T.);
#6287=EDGE_CURVE('',#4949,#4952,#3029,.T.);
#6288=EDGE_CURVE('',#4953,#4954,#3913,.T.);
#6289=EDGE_CURVE('',#4954,#4955,#3030,.T.);
#6290=EDGE_CURVE('',#4955,#4956,#3914,.T.);
#6291=EDGE_CURVE('',#4956,#4953,#3031,.T.);
#6292=EDGE_CURVE('',#4954,#4957,#3032,.T.);
#6293=EDGE_CURVE('',#4957,#4958,#3033,.T.);
#6294=EDGE_CURVE('',#4955,#4958,#3034,.T.);
#6295=EDGE_CURVE('',#4959,#4960,#3915,.T.);
#6296=EDGE_CURVE('',#4960,#4961,#3035,.T.);
#6297=EDGE_CURVE('',#4961,#4962,#3916,.T.);
#6298=EDGE_CURVE('',#4962,#4959,#3036,.T.);
#6299=EDGE_CURVE('',#4963,#4960,#3037,.T.);
#6300=EDGE_CURVE('',#4964,#4963,#3038,.T.);
#6301=EDGE_CURVE('',#4961,#4964,#3039,.T.);
#6302=EDGE_CURVE('',#4965,#4966,#3917,.T.);
#6303=EDGE_CURVE('',#4966,#4967,#3040,.T.);
#6304=EDGE_CURVE('',#4967,#4968,#3918,.T.);
#6305=EDGE_CURVE('',#4968,#4965,#3041,.T.);
#6306=EDGE_CURVE('',#4966,#4969,#3042,.T.);
#6307=EDGE_CURVE('',#4969,#4970,#3043,.T.);
#6308=EDGE_CURVE('',#4967,#4970,#3044,.T.);
#6309=EDGE_CURVE('',#4971,#4972,#3919,.T.);
#6310=EDGE_CURVE('',#4972,#4973,#3045,.T.);
#6311=EDGE_CURVE('',#4973,#4974,#3920,.T.);
#6312=EDGE_CURVE('',#4974,#4971,#3046,.T.);
#6313=EDGE_CURVE('',#4975,#4972,#3047,.T.);
#6314=EDGE_CURVE('',#4976,#4975,#3048,.T.);
#6315=EDGE_CURVE('',#4973,#4976,#3049,.T.);
#6316=EDGE_CURVE('',#4977,#4978,#3921,.T.);
#6317=EDGE_CURVE('',#4978,#4979,#3050,.T.);
#6318=EDGE_CURVE('',#4979,#4980,#3922,.T.);
#6319=EDGE_CURVE('',#4980,#4977,#3051,.T.);
#6320=EDGE_CURVE('',#4978,#4981,#3052,.T.);
#6321=EDGE_CURVE('',#4981,#4982,#3053,.T.);
#6322=EDGE_CURVE('',#4979,#4982,#3054,.T.);
#6323=EDGE_CURVE('',#4983,#4984,#3923,.T.);
#6324=EDGE_CURVE('',#4984,#4985,#3055,.T.);
#6325=EDGE_CURVE('',#4985,#4986,#3924,.T.);
#6326=EDGE_CURVE('',#4986,#4983,#3056,.T.);
#6327=EDGE_CURVE('',#4987,#4984,#3057,.T.);
#6328=EDGE_CURVE('',#4988,#4987,#3058,.T.);
#6329=EDGE_CURVE('',#4985,#4988,#3059,.T.);
#6330=EDGE_CURVE('',#4989,#4990,#3925,.T.);
#6331=EDGE_CURVE('',#4990,#4991,#3060,.T.);
#6332=EDGE_CURVE('',#4991,#4992,#3926,.T.);
#6333=EDGE_CURVE('',#4992,#4989,#3061,.T.);
#6334=EDGE_CURVE('',#4990,#4993,#3062,.T.);
#6335=EDGE_CURVE('',#4993,#4994,#3063,.T.);
#6336=EDGE_CURVE('',#4991,#4994,#3064,.T.);
#6337=EDGE_CURVE('',#4995,#4996,#3927,.T.);
#6338=EDGE_CURVE('',#4996,#4997,#3065,.T.);
#6339=EDGE_CURVE('',#4997,#4998,#3928,.T.);
#6340=EDGE_CURVE('',#4998,#4995,#3066,.T.);
#6341=EDGE_CURVE('',#4999,#4996,#3067,.T.);
#6342=EDGE_CURVE('',#5000,#4999,#3068,.T.);
#6343=EDGE_CURVE('',#4997,#5000,#3069,.T.);
#6344=EDGE_CURVE('',#5001,#5002,#3929,.T.);
#6345=EDGE_CURVE('',#5002,#5003,#3070,.T.);
#6346=EDGE_CURVE('',#5003,#5004,#3930,.T.);
#6347=EDGE_CURVE('',#5004,#5001,#3071,.T.);
#6348=EDGE_CURVE('',#5002,#5005,#3072,.T.);
#6349=EDGE_CURVE('',#5005,#5006,#3073,.T.);
#6350=EDGE_CURVE('',#5003,#5006,#3074,.T.);
#6351=EDGE_CURVE('',#5007,#5008,#3931,.T.);
#6352=EDGE_CURVE('',#5008,#5009,#3075,.T.);
#6353=EDGE_CURVE('',#5009,#5010,#3932,.T.);
#6354=EDGE_CURVE('',#5010,#5007,#3076,.T.);
#6355=EDGE_CURVE('',#5011,#5008,#3077,.T.);
#6356=EDGE_CURVE('',#5012,#5011,#3078,.T.);
#6357=EDGE_CURVE('',#5009,#5012,#3079,.T.);
#6358=EDGE_CURVE('',#5013,#5014,#3933,.T.);
#6359=EDGE_CURVE('',#5014,#5015,#3080,.T.);
#6360=EDGE_CURVE('',#5015,#5016,#3934,.T.);
#6361=EDGE_CURVE('',#5016,#5013,#3081,.T.);
#6362=EDGE_CURVE('',#5014,#5017,#3082,.T.);
#6363=EDGE_CURVE('',#5017,#5018,#3083,.T.);
#6364=EDGE_CURVE('',#5015,#5018,#3084,.T.);
#6365=EDGE_CURVE('',#5019,#5020,#3935,.T.);
#6366=EDGE_CURVE('',#5020,#5021,#3085,.T.);
#6367=EDGE_CURVE('',#5021,#5022,#3936,.T.);
#6368=EDGE_CURVE('',#5022,#5019,#3086,.T.);
#6369=EDGE_CURVE('',#5023,#5020,#3087,.T.);
#6370=EDGE_CURVE('',#5024,#5023,#3088,.T.);
#6371=EDGE_CURVE('',#5021,#5024,#3089,.T.);
#6372=EDGE_CURVE('',#5025,#5026,#3937,.T.);
#6373=EDGE_CURVE('',#5026,#5027,#3090,.T.);
#6374=EDGE_CURVE('',#5027,#5028,#3938,.T.);
#6375=EDGE_CURVE('',#5028,#5025,#3091,.T.);
#6376=EDGE_CURVE('',#5026,#5029,#3092,.T.);
#6377=EDGE_CURVE('',#5029,#5030,#3093,.T.);
#6378=EDGE_CURVE('',#5027,#5030,#3094,.T.);
#6379=EDGE_CURVE('',#5031,#5032,#3939,.T.);
#6380=EDGE_CURVE('',#5032,#5033,#3095,.T.);
#6381=EDGE_CURVE('',#5033,#5034,#3940,.T.);
#6382=EDGE_CURVE('',#5034,#5031,#3096,.T.);
#6383=EDGE_CURVE('',#5035,#5032,#3097,.T.);
#6384=EDGE_CURVE('',#5036,#5035,#3098,.T.);
#6385=EDGE_CURVE('',#5033,#5036,#3099,.T.);
#6386=EDGE_CURVE('',#5037,#5038,#3941,.T.);
#6387=EDGE_CURVE('',#5038,#5039,#3100,.T.);
#6388=EDGE_CURVE('',#5039,#5040,#3942,.T.);
#6389=EDGE_CURVE('',#5040,#5037,#3101,.T.);
#6390=EDGE_CURVE('',#5038,#5041,#3102,.T.);
#6391=EDGE_CURVE('',#5041,#5042,#3103,.T.);
#6392=EDGE_CURVE('',#5039,#5042,#3104,.T.);
#6393=EDGE_CURVE('',#5043,#5044,#3943,.T.);
#6394=EDGE_CURVE('',#5044,#5045,#3105,.T.);
#6395=EDGE_CURVE('',#5045,#5046,#3944,.T.);
#6396=EDGE_CURVE('',#5046,#5043,#3106,.T.);
#6397=EDGE_CURVE('',#5047,#5044,#3107,.T.);
#6398=EDGE_CURVE('',#5048,#5047,#3108,.T.);
#6399=EDGE_CURVE('',#5045,#5048,#3109,.T.);
#6400=EDGE_CURVE('',#5049,#5050,#3945,.T.);
#6401=EDGE_CURVE('',#5050,#5051,#3110,.T.);
#6402=EDGE_CURVE('',#5051,#5052,#3946,.T.);
#6403=EDGE_CURVE('',#5052,#5049,#3111,.T.);
#6404=EDGE_CURVE('',#5050,#5053,#3112,.T.);
#6405=EDGE_CURVE('',#5053,#5054,#3113,.T.);
#6406=EDGE_CURVE('',#5051,#5054,#3114,.T.);
#6407=EDGE_CURVE('',#5055,#5056,#3947,.T.);
#6408=EDGE_CURVE('',#5056,#5057,#3115,.T.);
#6409=EDGE_CURVE('',#5057,#5058,#3948,.T.);
#6410=EDGE_CURVE('',#5058,#5055,#3116,.T.);
#6411=EDGE_CURVE('',#5059,#5056,#3117,.T.);
#6412=EDGE_CURVE('',#5060,#5059,#3118,.T.);
#6413=EDGE_CURVE('',#5057,#5060,#3119,.T.);
#6414=EDGE_CURVE('',#5061,#5062,#3949,.T.);
#6415=EDGE_CURVE('',#5062,#5063,#3120,.T.);
#6416=EDGE_CURVE('',#5063,#5064,#3950,.T.);
#6417=EDGE_CURVE('',#5064,#5061,#3121,.T.);
#6418=EDGE_CURVE('',#5062,#5065,#3122,.T.);
#6419=EDGE_CURVE('',#5065,#5066,#3123,.T.);
#6420=EDGE_CURVE('',#5063,#5066,#3124,.T.);
#6421=EDGE_CURVE('',#5067,#5068,#3951,.T.);
#6422=EDGE_CURVE('',#5068,#5069,#3125,.T.);
#6423=EDGE_CURVE('',#5069,#5070,#3952,.T.);
#6424=EDGE_CURVE('',#5070,#5067,#3126,.T.);
#6425=EDGE_CURVE('',#5071,#5068,#3127,.T.);
#6426=EDGE_CURVE('',#5072,#5071,#3128,.T.);
#6427=EDGE_CURVE('',#5069,#5072,#3129,.T.);
#6428=EDGE_CURVE('',#5073,#5074,#3953,.T.);
#6429=EDGE_CURVE('',#5074,#5075,#3130,.T.);
#6430=EDGE_CURVE('',#5075,#5076,#3954,.T.);
#6431=EDGE_CURVE('',#5076,#5073,#3131,.T.);
#6432=EDGE_CURVE('',#5074,#5077,#3132,.T.);
#6433=EDGE_CURVE('',#5077,#5078,#3133,.T.);
#6434=EDGE_CURVE('',#5075,#5078,#3134,.T.);
#6435=EDGE_CURVE('',#5079,#5080,#3955,.T.);
#6436=EDGE_CURVE('',#5080,#5081,#3135,.T.);
#6437=EDGE_CURVE('',#5081,#5082,#3956,.T.);
#6438=EDGE_CURVE('',#5082,#5079,#3136,.T.);
#6439=EDGE_CURVE('',#5083,#5080,#3137,.T.);
#6440=EDGE_CURVE('',#5084,#5083,#3138,.T.);
#6441=EDGE_CURVE('',#5081,#5084,#3139,.T.);
#6442=EDGE_CURVE('',#5085,#5086,#3957,.T.);
#6443=EDGE_CURVE('',#5086,#5087,#3140,.T.);
#6444=EDGE_CURVE('',#5087,#5088,#3958,.T.);
#6445=EDGE_CURVE('',#5088,#5085,#3141,.T.);
#6446=EDGE_CURVE('',#5086,#5089,#3142,.T.);
#6447=EDGE_CURVE('',#5089,#5090,#3143,.T.);
#6448=EDGE_CURVE('',#5087,#5090,#3144,.T.);
#6449=EDGE_CURVE('',#5091,#5092,#3959,.T.);
#6450=EDGE_CURVE('',#5092,#5093,#3145,.T.);
#6451=EDGE_CURVE('',#5093,#5094,#3960,.T.);
#6452=EDGE_CURVE('',#5094,#5091,#3146,.T.);
#6453=EDGE_CURVE('',#5095,#5092,#3147,.T.);
#6454=EDGE_CURVE('',#5096,#5095,#3148,.T.);
#6455=EDGE_CURVE('',#5093,#5096,#3149,.T.);
#6456=EDGE_CURVE('',#5097,#5098,#3961,.T.);
#6457=EDGE_CURVE('',#5098,#5099,#3150,.T.);
#6458=EDGE_CURVE('',#5099,#5100,#3962,.T.);
#6459=EDGE_CURVE('',#5100,#5097,#3151,.T.);
#6460=EDGE_CURVE('',#5098,#5101,#3152,.T.);
#6461=EDGE_CURVE('',#5101,#5102,#3153,.T.);
#6462=EDGE_CURVE('',#5099,#5102,#3154,.T.);
#6463=EDGE_CURVE('',#5103,#5104,#3963,.T.);
#6464=EDGE_CURVE('',#5104,#5105,#3155,.T.);
#6465=EDGE_CURVE('',#5105,#5106,#3964,.T.);
#6466=EDGE_CURVE('',#5106,#5103,#3156,.T.);
#6467=EDGE_CURVE('',#5107,#5104,#3157,.T.);
#6468=EDGE_CURVE('',#5108,#5107,#3158,.T.);
#6469=EDGE_CURVE('',#5105,#5108,#3159,.T.);
#6470=EDGE_CURVE('',#5109,#5110,#3965,.T.);
#6471=EDGE_CURVE('',#5110,#5111,#3160,.T.);
#6472=EDGE_CURVE('',#5111,#5112,#3966,.T.);
#6473=EDGE_CURVE('',#5112,#5109,#3161,.T.);
#6474=EDGE_CURVE('',#5110,#5113,#3162,.T.);
#6475=EDGE_CURVE('',#5113,#5114,#3163,.T.);
#6476=EDGE_CURVE('',#5111,#5114,#3164,.T.);
#6477=EDGE_CURVE('',#5115,#5116,#3967,.T.);
#6478=EDGE_CURVE('',#5116,#5117,#3165,.T.);
#6479=EDGE_CURVE('',#5117,#5118,#3968,.T.);
#6480=EDGE_CURVE('',#5118,#5115,#3166,.T.);
#6481=EDGE_CURVE('',#5119,#5116,#3167,.T.);
#6482=EDGE_CURVE('',#5120,#5119,#3168,.T.);
#6483=EDGE_CURVE('',#5117,#5120,#3169,.T.);
#6484=EDGE_CURVE('',#5121,#5122,#3969,.T.);
#6485=EDGE_CURVE('',#5122,#5123,#3170,.T.);
#6486=EDGE_CURVE('',#5123,#5124,#3970,.T.);
#6487=EDGE_CURVE('',#5124,#5121,#3171,.T.);
#6488=EDGE_CURVE('',#5122,#5125,#3172,.T.);
#6489=EDGE_CURVE('',#5125,#5126,#3173,.T.);
#6490=EDGE_CURVE('',#5123,#5126,#3174,.T.);
#6491=EDGE_CURVE('',#5127,#5128,#3971,.T.);
#6492=EDGE_CURVE('',#5128,#5129,#3175,.T.);
#6493=EDGE_CURVE('',#5129,#5130,#3972,.T.);
#6494=EDGE_CURVE('',#5130,#5127,#3176,.T.);
#6495=EDGE_CURVE('',#5131,#5128,#3177,.T.);
#6496=EDGE_CURVE('',#5132,#5131,#3178,.T.);
#6497=EDGE_CURVE('',#5129,#5132,#3179,.T.);
#6498=EDGE_CURVE('',#5133,#5134,#3973,.T.);
#6499=EDGE_CURVE('',#5134,#5135,#3180,.T.);
#6500=EDGE_CURVE('',#5135,#5136,#3974,.T.);
#6501=EDGE_CURVE('',#5136,#5133,#3181,.T.);
#6502=EDGE_CURVE('',#5134,#5137,#3182,.T.);
#6503=EDGE_CURVE('',#5137,#5138,#3183,.T.);
#6504=EDGE_CURVE('',#5135,#5138,#3184,.T.);
#6505=EDGE_CURVE('',#5139,#5140,#3975,.T.);
#6506=EDGE_CURVE('',#5140,#5141,#3185,.T.);
#6507=EDGE_CURVE('',#5141,#5142,#3976,.T.);
#6508=EDGE_CURVE('',#5142,#5139,#3186,.T.);
#6509=EDGE_CURVE('',#5143,#5140,#3187,.T.);
#6510=EDGE_CURVE('',#5144,#5143,#3188,.T.);
#6511=EDGE_CURVE('',#5141,#5144,#3189,.T.);
#6512=EDGE_CURVE('',#5145,#5146,#3977,.T.);
#6513=EDGE_CURVE('',#5146,#5147,#3190,.T.);
#6514=EDGE_CURVE('',#5147,#5148,#3978,.T.);
#6515=EDGE_CURVE('',#5148,#5145,#3191,.T.);
#6516=EDGE_CURVE('',#5146,#5149,#3192,.T.);
#6517=EDGE_CURVE('',#5149,#5150,#3193,.T.);
#6518=EDGE_CURVE('',#5147,#5150,#3194,.T.);
#6519=EDGE_CURVE('',#4928,#5151,#491,.T.);
#6520=EDGE_CURVE('',#5152,#4927,#492,.T.);
#6521=EDGE_CURVE('',#5151,#5152,#3195,.T.);
#6522=EDGE_CURVE('',#5153,#5151,#3979,.T.);
#6523=EDGE_CURVE('',#5154,#5152,#3980,.T.);
#6524=EDGE_CURVE('',#5153,#5154,#3196,.T.);
#6525=EDGE_CURVE('',#4933,#5153,#493,.T.);
#6526=EDGE_CURVE('',#4934,#5154,#494,.T.);
#6527=EDGE_CURVE('',#4940,#5155,#495,.T.);
#6528=EDGE_CURVE('',#5156,#4939,#496,.T.);
#6529=EDGE_CURVE('',#5155,#5156,#3197,.T.);
#6530=EDGE_CURVE('',#5157,#5155,#3981,.T.);
#6531=EDGE_CURVE('',#5158,#5156,#3982,.T.);
#6532=EDGE_CURVE('',#5157,#5158,#3198,.T.);
#6533=EDGE_CURVE('',#4945,#5157,#497,.T.);
#6534=EDGE_CURVE('',#4946,#5158,#498,.T.);
#6535=EDGE_CURVE('',#4952,#5159,#499,.T.);
#6536=EDGE_CURVE('',#5160,#4951,#500,.T.);
#6537=EDGE_CURVE('',#5159,#5160,#3199,.T.);
#6538=EDGE_CURVE('',#5161,#5159,#3983,.T.);
#6539=EDGE_CURVE('',#5162,#5160,#3984,.T.);
#6540=EDGE_CURVE('',#5161,#5162,#3200,.T.);
#6541=EDGE_CURVE('',#4957,#5161,#501,.T.);
#6542=EDGE_CURVE('',#4958,#5162,#502,.T.);
#6543=EDGE_CURVE('',#4964,#5163,#503,.T.);
#6544=EDGE_CURVE('',#5164,#4963,#504,.T.);
#6545=EDGE_CURVE('',#5163,#5164,#3201,.T.);
#6546=EDGE_CURVE('',#5165,#5163,#3985,.T.);
#6547=EDGE_CURVE('',#5166,#5164,#3986,.T.);
#6548=EDGE_CURVE('',#5165,#5166,#3202,.T.);
#6549=EDGE_CURVE('',#4969,#5165,#505,.T.);
#6550=EDGE_CURVE('',#4970,#5166,#506,.T.);
#6551=EDGE_CURVE('',#4976,#5167,#507,.T.);
#6552=EDGE_CURVE('',#5168,#4975,#508,.T.);
#6553=EDGE_CURVE('',#5167,#5168,#3203,.T.);
#6554=EDGE_CURVE('',#5169,#5167,#3987,.T.);
#6555=EDGE_CURVE('',#5170,#5168,#3988,.T.);
#6556=EDGE_CURVE('',#5169,#5170,#3204,.T.);
#6557=EDGE_CURVE('',#4981,#5169,#509,.T.);
#6558=EDGE_CURVE('',#4982,#5170,#510,.T.);
#6559=EDGE_CURVE('',#4988,#5171,#511,.T.);
#6560=EDGE_CURVE('',#5172,#4987,#512,.T.);
#6561=EDGE_CURVE('',#5171,#5172,#3205,.T.);
#6562=EDGE_CURVE('',#5173,#5171,#3989,.T.);
#6563=EDGE_CURVE('',#5174,#5172,#3990,.T.);
#6564=EDGE_CURVE('',#5173,#5174,#3206,.T.);
#6565=EDGE_CURVE('',#4993,#5173,#513,.T.);
#6566=EDGE_CURVE('',#4994,#5174,#514,.T.);
#6567=EDGE_CURVE('',#5000,#5175,#515,.T.);
#6568=EDGE_CURVE('',#5176,#4999,#516,.T.);
#6569=EDGE_CURVE('',#5175,#5176,#3207,.T.);
#6570=EDGE_CURVE('',#5177,#5175,#3991,.T.);
#6571=EDGE_CURVE('',#5178,#5176,#3992,.T.);
#6572=EDGE_CURVE('',#5177,#5178,#3208,.T.);
#6573=EDGE_CURVE('',#5005,#5177,#517,.T.);
#6574=EDGE_CURVE('',#5006,#5178,#518,.T.);
#6575=EDGE_CURVE('',#5012,#5179,#519,.T.);
#6576=EDGE_CURVE('',#5180,#5011,#520,.T.);
#6577=EDGE_CURVE('',#5179,#5180,#3209,.T.);
#6578=EDGE_CURVE('',#5181,#5179,#3993,.T.);
#6579=EDGE_CURVE('',#5182,#5180,#3994,.T.);
#6580=EDGE_CURVE('',#5181,#5182,#3210,.T.);
#6581=EDGE_CURVE('',#5017,#5181,#521,.T.);
#6582=EDGE_CURVE('',#5018,#5182,#522,.T.);
#6583=EDGE_CURVE('',#5024,#5183,#523,.T.);
#6584=EDGE_CURVE('',#5184,#5023,#524,.T.);
#6585=EDGE_CURVE('',#5183,#5184,#3211,.T.);
#6586=EDGE_CURVE('',#5185,#5183,#3995,.T.);
#6587=EDGE_CURVE('',#5186,#5184,#3996,.T.);
#6588=EDGE_CURVE('',#5185,#5186,#3212,.T.);
#6589=EDGE_CURVE('',#5029,#5185,#525,.T.);
#6590=EDGE_CURVE('',#5030,#5186,#526,.T.);
#6591=EDGE_CURVE('',#5036,#5187,#527,.T.);
#6592=EDGE_CURVE('',#5188,#5035,#528,.T.);
#6593=EDGE_CURVE('',#5187,#5188,#3213,.T.);
#6594=EDGE_CURVE('',#5189,#5187,#3997,.T.);
#6595=EDGE_CURVE('',#5190,#5188,#3998,.T.);
#6596=EDGE_CURVE('',#5189,#5190,#3214,.T.);
#6597=EDGE_CURVE('',#5041,#5189,#529,.T.);
#6598=EDGE_CURVE('',#5042,#5190,#530,.T.);
#6599=EDGE_CURVE('',#5048,#5191,#531,.T.);
#6600=EDGE_CURVE('',#5192,#5047,#532,.T.);
#6601=EDGE_CURVE('',#5191,#5192,#3215,.T.);
#6602=EDGE_CURVE('',#5193,#5191,#3999,.T.);
#6603=EDGE_CURVE('',#5194,#5192,#4000,.T.);
#6604=EDGE_CURVE('',#5193,#5194,#3216,.T.);
#6605=EDGE_CURVE('',#5053,#5193,#533,.T.);
#6606=EDGE_CURVE('',#5054,#5194,#534,.T.);
#6607=EDGE_CURVE('',#5060,#5195,#535,.T.);
#6608=EDGE_CURVE('',#5196,#5059,#536,.T.);
#6609=EDGE_CURVE('',#5195,#5196,#3217,.T.);
#6610=EDGE_CURVE('',#5197,#5195,#4001,.T.);
#6611=EDGE_CURVE('',#5198,#5196,#4002,.T.);
#6612=EDGE_CURVE('',#5197,#5198,#3218,.T.);
#6613=EDGE_CURVE('',#5065,#5197,#537,.T.);
#6614=EDGE_CURVE('',#5066,#5198,#538,.T.);
#6615=EDGE_CURVE('',#5072,#5199,#539,.T.);
#6616=EDGE_CURVE('',#5200,#5071,#540,.T.);
#6617=EDGE_CURVE('',#5199,#5200,#3219,.T.);
#6618=EDGE_CURVE('',#5201,#5199,#4003,.T.);
#6619=EDGE_CURVE('',#5202,#5200,#4004,.T.);
#6620=EDGE_CURVE('',#5201,#5202,#3220,.T.);
#6621=EDGE_CURVE('',#5077,#5201,#541,.T.);
#6622=EDGE_CURVE('',#5078,#5202,#542,.T.);
#6623=EDGE_CURVE('',#5084,#5203,#543,.T.);
#6624=EDGE_CURVE('',#5204,#5083,#544,.T.);
#6625=EDGE_CURVE('',#5203,#5204,#3221,.T.);
#6626=EDGE_CURVE('',#5205,#5203,#4005,.T.);
#6627=EDGE_CURVE('',#5206,#5204,#4006,.T.);
#6628=EDGE_CURVE('',#5205,#5206,#3222,.T.);
#6629=EDGE_CURVE('',#5089,#5205,#545,.T.);
#6630=EDGE_CURVE('',#5090,#5206,#546,.T.);
#6631=EDGE_CURVE('',#5096,#5207,#547,.T.);
#6632=EDGE_CURVE('',#5208,#5095,#548,.T.);
#6633=EDGE_CURVE('',#5207,#5208,#3223,.T.);
#6634=EDGE_CURVE('',#5209,#5207,#4007,.T.);
#6635=EDGE_CURVE('',#5210,#5208,#4008,.T.);
#6636=EDGE_CURVE('',#5209,#5210,#3224,.T.);
#6637=EDGE_CURVE('',#5101,#5209,#549,.T.);
#6638=EDGE_CURVE('',#5102,#5210,#550,.T.);
#6639=EDGE_CURVE('',#5108,#5211,#551,.T.);
#6640=EDGE_CURVE('',#5212,#5107,#552,.T.);
#6641=EDGE_CURVE('',#5211,#5212,#3225,.T.);
#6642=EDGE_CURVE('',#5213,#5211,#4009,.T.);
#6643=EDGE_CURVE('',#5214,#5212,#4010,.T.);
#6644=EDGE_CURVE('',#5213,#5214,#3226,.T.);
#6645=EDGE_CURVE('',#5113,#5213,#553,.T.);
#6646=EDGE_CURVE('',#5114,#5214,#554,.T.);
#6647=EDGE_CURVE('',#5120,#5215,#555,.T.);
#6648=EDGE_CURVE('',#5216,#5119,#556,.T.);
#6649=EDGE_CURVE('',#5215,#5216,#3227,.T.);
#6650=EDGE_CURVE('',#5217,#5215,#4011,.T.);
#6651=EDGE_CURVE('',#5218,#5216,#4012,.T.);
#6652=EDGE_CURVE('',#5217,#5218,#3228,.T.);
#6653=EDGE_CURVE('',#5125,#5217,#557,.T.);
#6654=EDGE_CURVE('',#5126,#5218,#558,.T.);
#6655=EDGE_CURVE('',#5132,#5219,#559,.T.);
#6656=EDGE_CURVE('',#5220,#5131,#560,.T.);
#6657=EDGE_CURVE('',#5219,#5220,#3229,.T.);
#6658=EDGE_CURVE('',#5221,#5219,#4013,.T.);
#6659=EDGE_CURVE('',#5222,#5220,#4014,.T.);
#6660=EDGE_CURVE('',#5221,#5222,#3230,.T.);
#6661=EDGE_CURVE('',#5137,#5221,#561,.T.);
#6662=EDGE_CURVE('',#5138,#5222,#562,.T.);
#6663=EDGE_CURVE('',#5144,#5223,#563,.T.);
#6664=EDGE_CURVE('',#5224,#5143,#564,.T.);
#6665=EDGE_CURVE('',#5223,#5224,#3231,.T.);
#6666=EDGE_CURVE('',#5225,#5223,#4015,.T.);
#6667=EDGE_CURVE('',#5226,#5224,#4016,.T.);
#6668=EDGE_CURVE('',#5225,#5226,#3232,.T.);
#6669=EDGE_CURVE('',#5149,#5225,#565,.T.);
#6670=EDGE_CURVE('',#5150,#5226,#566,.T.);
#6671=EDGE_CURVE('',#4950,#4941,#4017,.T.);
#6672=EDGE_CURVE('',#4962,#4953,#4018,.T.);
#6673=EDGE_CURVE('',#4974,#4965,#4019,.T.);
#6674=EDGE_CURVE('',#4986,#4977,#4020,.T.);
#6675=EDGE_CURVE('',#4998,#4989,#4021,.T.);
#6676=EDGE_CURVE('',#5010,#5001,#4022,.T.);
#6677=EDGE_CURVE('',#5022,#5013,#4023,.T.);
#6678=EDGE_CURVE('',#5034,#5025,#4024,.T.);
#6679=EDGE_CURVE('',#5046,#5037,#4025,.T.);
#6680=EDGE_CURVE('',#5058,#5049,#4026,.T.);
#6681=EDGE_CURVE('',#5070,#5061,#4027,.T.);
#6682=EDGE_CURVE('',#5082,#5073,#4028,.T.);
#6683=EDGE_CURVE('',#5094,#5085,#4029,.T.);
#6684=EDGE_CURVE('',#5106,#5097,#4030,.T.);
#6685=EDGE_CURVE('',#5118,#5109,#4031,.T.);
#6686=EDGE_CURVE('',#5130,#5121,#4032,.T.);
#6687=EDGE_CURVE('',#5142,#5133,#4033,.T.);
#6688=EDGE_CURVE('',#5227,#5145,#4034,.T.);
#6689=EDGE_CURVE('',#5228,#5227,#4035,.T.);
#6690=EDGE_CURVE('',#5228,#5229,#3233,.T.);
#6691=EDGE_CURVE('',#5229,#5230,#567,.T.);
#6692=EDGE_CURVE('',#5231,#5230,#4036,.T.);
#6693=EDGE_CURVE('',#5232,#5231,#568,.T.);
#6694=EDGE_CURVE('',#5233,#5232,#3234,.T.);
#6695=EDGE_CURVE('',#5234,#5233,#4037,.T.);
#6696=EDGE_CURVE('',#4926,#5234,#4038,.T.);
#6697=EDGE_CURVE('',#4938,#4929,#4039,.T.);
#6698=EDGE_CURVE('',#4923,#5235,#4040,.T.);
#6699=EDGE_CURVE('',#5236,#5235,#4041,.T.);
#6700=EDGE_CURVE('',#5236,#5237,#3235,.T.);
#6701=EDGE_CURVE('',#5237,#5238,#569,.T.);
#6702=EDGE_CURVE('',#5238,#5239,#4042,.T.);
#6703=EDGE_CURVE('',#5239,#5240,#570,.T.);
#6704=EDGE_CURVE('',#5240,#5241,#3236,.T.);
#6705=EDGE_CURVE('',#5242,#5241,#4043,.T.);
#6706=EDGE_CURVE('',#5242,#5148,#4044,.T.);
#6707=EDGE_CURVE('',#5139,#5136,#4045,.T.);
#6708=EDGE_CURVE('',#5127,#5124,#4046,.T.);
#6709=EDGE_CURVE('',#5115,#5112,#4047,.T.);
#6710=EDGE_CURVE('',#5103,#5100,#4048,.T.);
#6711=EDGE_CURVE('',#5091,#5088,#4049,.T.);
#6712=EDGE_CURVE('',#5079,#5076,#4050,.T.);
#6713=EDGE_CURVE('',#5067,#5064,#4051,.T.);
#6714=EDGE_CURVE('',#5055,#5052,#4052,.T.);
#6715=EDGE_CURVE('',#5043,#5040,#4053,.T.);
#6716=EDGE_CURVE('',#5031,#5028,#4054,.T.);
#6717=EDGE_CURVE('',#5019,#5016,#4055,.T.);
#6718=EDGE_CURVE('',#5007,#5004,#4056,.T.);
#6719=EDGE_CURVE('',#4995,#4992,#4057,.T.);
#6720=EDGE_CURVE('',#4983,#4980,#4058,.T.);
#6721=EDGE_CURVE('',#4971,#4968,#4059,.T.);
#6722=EDGE_CURVE('',#4959,#4956,#4060,.T.);
#6723=EDGE_CURVE('',#4947,#4944,#4061,.T.);
#6724=EDGE_CURVE('',#4935,#4932,#4062,.T.);
#6725=EDGE_CURVE('',#5227,#5242,#3237,.T.);
#6726=EDGE_CURVE('',#5241,#5228,#3238,.T.);
#6727=EDGE_CURVE('',#5229,#5240,#3239,.T.);
#6728=EDGE_CURVE('',#5233,#5236,#3240,.T.);
#6729=EDGE_CURVE('',#5235,#5234,#3241,.T.);
#6730=EDGE_CURVE('',#5232,#5237,#3242,.T.);
#6731=EDGE_CURVE('',#5230,#5239,#3243,.T.);
#6732=EDGE_CURVE('',#5231,#5238,#3244,.T.);
#8171=ORIENTED_EDGE('',*,*,#6247,.F.);
#8172=ORIENTED_EDGE('',*,*,#6248,.T.);
#8173=ORIENTED_EDGE('',*,*,#6249,.F.);
#8174=ORIENTED_EDGE('',*,*,#6248,.F.);
#8175=ORIENTED_EDGE('',*,*,#6250,.F.);
#8176=ORIENTED_EDGE('',*,*,#6251,.T.);
#8177=ORIENTED_EDGE('',*,*,#6252,.F.);
#8178=ORIENTED_EDGE('',*,*,#6251,.F.);
#8179=ORIENTED_EDGE('',*,*,#6249,.T.);
#8180=ORIENTED_EDGE('',*,*,#6250,.T.);
#8181=ORIENTED_EDGE('',*,*,#6253,.T.);
#8182=ORIENTED_EDGE('',*,*,#6254,.T.);
#8183=ORIENTED_EDGE('',*,*,#6255,.T.);
#8184=ORIENTED_EDGE('',*,*,#6256,.T.);
#8185=ORIENTED_EDGE('',*,*,#6254,.F.);
#8186=ORIENTED_EDGE('',*,*,#6257,.F.);
#8187=ORIENTED_EDGE('',*,*,#6258,.F.);
#8188=ORIENTED_EDGE('',*,*,#6259,.F.);
#8189=ORIENTED_EDGE('',*,*,#6260,.T.);
#8190=ORIENTED_EDGE('',*,*,#6261,.T.);
#8191=ORIENTED_EDGE('',*,*,#6262,.T.);
#8192=ORIENTED_EDGE('',*,*,#6263,.T.);
#8193=ORIENTED_EDGE('',*,*,#6261,.F.);
#8194=ORIENTED_EDGE('',*,*,#6264,.T.);
#8195=ORIENTED_EDGE('',*,*,#6265,.T.);
#8196=ORIENTED_EDGE('',*,*,#6266,.F.);
#8197=ORIENTED_EDGE('',*,*,#6267,.T.);
#8198=ORIENTED_EDGE('',*,*,#6268,.T.);
#8199=ORIENTED_EDGE('',*,*,#6269,.T.);
#8200=ORIENTED_EDGE('',*,*,#6270,.T.);
#8201=ORIENTED_EDGE('',*,*,#6268,.F.);
#8202=ORIENTED_EDGE('',*,*,#6271,.F.);
#8203=ORIENTED_EDGE('',*,*,#6272,.F.);
#8204=ORIENTED_EDGE('',*,*,#6273,.F.);
#8205=ORIENTED_EDGE('',*,*,#6274,.T.);
#8206=ORIENTED_EDGE('',*,*,#6275,.T.);
#8207=ORIENTED_EDGE('',*,*,#6276,.T.);
#8208=ORIENTED_EDGE('',*,*,#6277,.T.);
#8209=ORIENTED_EDGE('',*,*,#6275,.F.);
#8210=ORIENTED_EDGE('',*,*,#6278,.T.);
#8211=ORIENTED_EDGE('',*,*,#6279,.T.);
#8212=ORIENTED_EDGE('',*,*,#6280,.F.);
#8213=ORIENTED_EDGE('',*,*,#6281,.T.);
#8214=ORIENTED_EDGE('',*,*,#6282,.T.);
#8215=ORIENTED_EDGE('',*,*,#6283,.T.);
#8216=ORIENTED_EDGE('',*,*,#6284,.T.);
#8217=ORIENTED_EDGE('',*,*,#6282,.F.);
#8218=ORIENTED_EDGE('',*,*,#6285,.F.);
#8219=ORIENTED_EDGE('',*,*,#6286,.F.);
#8220=ORIENTED_EDGE('',*,*,#6287,.F.);
#8221=ORIENTED_EDGE('',*,*,#6288,.T.);
#8222=ORIENTED_EDGE('',*,*,#6289,.T.);
#8223=ORIENTED_EDGE('',*,*,#6290,.T.);
#8224=ORIENTED_EDGE('',*,*,#6291,.T.);
#8225=ORIENTED_EDGE('',*,*,#6289,.F.);
#8226=ORIENTED_EDGE('',*,*,#6292,.T.);
#8227=ORIENTED_EDGE('',*,*,#6293,.T.);
#8228=ORIENTED_EDGE('',*,*,#6294,.F.);
#8229=ORIENTED_EDGE('',*,*,#6295,.T.);
#8230=ORIENTED_EDGE('',*,*,#6296,.T.);
#8231=ORIENTED_EDGE('',*,*,#6297,.T.);
#8232=ORIENTED_EDGE('',*,*,#6298,.T.);
#8233=ORIENTED_EDGE('',*,*,#6296,.F.);
#8234=ORIENTED_EDGE('',*,*,#6299,.F.);
#8235=ORIENTED_EDGE('',*,*,#6300,.F.);
#8236=ORIENTED_EDGE('',*,*,#6301,.F.);
#8237=ORIENTED_EDGE('',*,*,#6302,.T.);
#8238=ORIENTED_EDGE('',*,*,#6303,.T.);
#8239=ORIENTED_EDGE('',*,*,#6304,.T.);
#8240=ORIENTED_EDGE('',*,*,#6305,.T.);
#8241=ORIENTED_EDGE('',*,*,#6303,.F.);
#8242=ORIENTED_EDGE('',*,*,#6306,.T.);
#8243=ORIENTED_EDGE('',*,*,#6307,.T.);
#8244=ORIENTED_EDGE('',*,*,#6308,.F.);
#8245=ORIENTED_EDGE('',*,*,#6309,.T.);
#8246=ORIENTED_EDGE('',*,*,#6310,.T.);
#8247=ORIENTED_EDGE('',*,*,#6311,.T.);
#8248=ORIENTED_EDGE('',*,*,#6312,.T.);
#8249=ORIENTED_EDGE('',*,*,#6310,.F.);
#8250=ORIENTED_EDGE('',*,*,#6313,.F.);
#8251=ORIENTED_EDGE('',*,*,#6314,.F.);
#8252=ORIENTED_EDGE('',*,*,#6315,.F.);
#8253=ORIENTED_EDGE('',*,*,#6316,.T.);
#8254=ORIENTED_EDGE('',*,*,#6317,.T.);
#8255=ORIENTED_EDGE('',*,*,#6318,.T.);
#8256=ORIENTED_EDGE('',*,*,#6319,.T.);
#8257=ORIENTED_EDGE('',*,*,#6317,.F.);
#8258=ORIENTED_EDGE('',*,*,#6320,.T.);
#8259=ORIENTED_EDGE('',*,*,#6321,.T.);
#8260=ORIENTED_EDGE('',*,*,#6322,.F.);
#8261=ORIENTED_EDGE('',*,*,#6323,.T.);
#8262=ORIENTED_EDGE('',*,*,#6324,.T.);
#8263=ORIENTED_EDGE('',*,*,#6325,.T.);
#8264=ORIENTED_EDGE('',*,*,#6326,.T.);
#8265=ORIENTED_EDGE('',*,*,#6324,.F.);
#8266=ORIENTED_EDGE('',*,*,#6327,.F.);
#8267=ORIENTED_EDGE('',*,*,#6328,.F.);
#8268=ORIENTED_EDGE('',*,*,#6329,.F.);
#8269=ORIENTED_EDGE('',*,*,#6330,.T.);
#8270=ORIENTED_EDGE('',*,*,#6331,.T.);
#8271=ORIENTED_EDGE('',*,*,#6332,.T.);
#8272=ORIENTED_EDGE('',*,*,#6333,.T.);
#8273=ORIENTED_EDGE('',*,*,#6331,.F.);
#8274=ORIENTED_EDGE('',*,*,#6334,.T.);
#8275=ORIENTED_EDGE('',*,*,#6335,.T.);
#8276=ORIENTED_EDGE('',*,*,#6336,.F.);
#8277=ORIENTED_EDGE('',*,*,#6337,.T.);
#8278=ORIENTED_EDGE('',*,*,#6338,.T.);
#8279=ORIENTED_EDGE('',*,*,#6339,.T.);
#8280=ORIENTED_EDGE('',*,*,#6340,.T.);
#8281=ORIENTED_EDGE('',*,*,#6338,.F.);
#8282=ORIENTED_EDGE('',*,*,#6341,.F.);
#8283=ORIENTED_EDGE('',*,*,#6342,.F.);
#8284=ORIENTED_EDGE('',*,*,#6343,.F.);
#8285=ORIENTED_EDGE('',*,*,#6344,.T.);
#8286=ORIENTED_EDGE('',*,*,#6345,.T.);
#8287=ORIENTED_EDGE('',*,*,#6346,.T.);
#8288=ORIENTED_EDGE('',*,*,#6347,.T.);
#8289=ORIENTED_EDGE('',*,*,#6345,.F.);
#8290=ORIENTED_EDGE('',*,*,#6348,.T.);
#8291=ORIENTED_EDGE('',*,*,#6349,.T.);
#8292=ORIENTED_EDGE('',*,*,#6350,.F.);
#8293=ORIENTED_EDGE('',*,*,#6351,.T.);
#8294=ORIENTED_EDGE('',*,*,#6352,.T.);
#8295=ORIENTED_EDGE('',*,*,#6353,.T.);
#8296=ORIENTED_EDGE('',*,*,#6354,.T.);
#8297=ORIENTED_EDGE('',*,*,#6352,.F.);
#8298=ORIENTED_EDGE('',*,*,#6355,.F.);
#8299=ORIENTED_EDGE('',*,*,#6356,.F.);
#8300=ORIENTED_EDGE('',*,*,#6357,.F.);
#8301=ORIENTED_EDGE('',*,*,#6358,.T.);
#8302=ORIENTED_EDGE('',*,*,#6359,.T.);
#8303=ORIENTED_EDGE('',*,*,#6360,.T.);
#8304=ORIENTED_EDGE('',*,*,#6361,.T.);
#8305=ORIENTED_EDGE('',*,*,#6359,.F.);
#8306=ORIENTED_EDGE('',*,*,#6362,.T.);
#8307=ORIENTED_EDGE('',*,*,#6363,.T.);
#8308=ORIENTED_EDGE('',*,*,#6364,.F.);
#8309=ORIENTED_EDGE('',*,*,#6365,.T.);
#8310=ORIENTED_EDGE('',*,*,#6366,.T.);
#8311=ORIENTED_EDGE('',*,*,#6367,.T.);
#8312=ORIENTED_EDGE('',*,*,#6368,.T.);
#8313=ORIENTED_EDGE('',*,*,#6366,.F.);
#8314=ORIENTED_EDGE('',*,*,#6369,.F.);
#8315=ORIENTED_EDGE('',*,*,#6370,.F.);
#8316=ORIENTED_EDGE('',*,*,#6371,.F.);
#8317=ORIENTED_EDGE('',*,*,#6372,.T.);
#8318=ORIENTED_EDGE('',*,*,#6373,.T.);
#8319=ORIENTED_EDGE('',*,*,#6374,.T.);
#8320=ORIENTED_EDGE('',*,*,#6375,.T.);
#8321=ORIENTED_EDGE('',*,*,#6373,.F.);
#8322=ORIENTED_EDGE('',*,*,#6376,.T.);
#8323=ORIENTED_EDGE('',*,*,#6377,.T.);
#8324=ORIENTED_EDGE('',*,*,#6378,.F.);
#8325=ORIENTED_EDGE('',*,*,#6379,.T.);
#8326=ORIENTED_EDGE('',*,*,#6380,.T.);
#8327=ORIENTED_EDGE('',*,*,#6381,.T.);
#8328=ORIENTED_EDGE('',*,*,#6382,.T.);
#8329=ORIENTED_EDGE('',*,*,#6380,.F.);
#8330=ORIENTED_EDGE('',*,*,#6383,.F.);
#8331=ORIENTED_EDGE('',*,*,#6384,.F.);
#8332=ORIENTED_EDGE('',*,*,#6385,.F.);
#8333=ORIENTED_EDGE('',*,*,#6386,.T.);
#8334=ORIENTED_EDGE('',*,*,#6387,.T.);
#8335=ORIENTED_EDGE('',*,*,#6388,.T.);
#8336=ORIENTED_EDGE('',*,*,#6389,.T.);
#8337=ORIENTED_EDGE('',*,*,#6387,.F.);
#8338=ORIENTED_EDGE('',*,*,#6390,.T.);
#8339=ORIENTED_EDGE('',*,*,#6391,.T.);
#8340=ORIENTED_EDGE('',*,*,#6392,.F.);
#8341=ORIENTED_EDGE('',*,*,#6393,.T.);
#8342=ORIENTED_EDGE('',*,*,#6394,.T.);
#8343=ORIENTED_EDGE('',*,*,#6395,.T.);
#8344=ORIENTED_EDGE('',*,*,#6396,.T.);
#8345=ORIENTED_EDGE('',*,*,#6394,.F.);
#8346=ORIENTED_EDGE('',*,*,#6397,.F.);
#8347=ORIENTED_EDGE('',*,*,#6398,.F.);
#8348=ORIENTED_EDGE('',*,*,#6399,.F.);
#8349=ORIENTED_EDGE('',*,*,#6400,.T.);
#8350=ORIENTED_EDGE('',*,*,#6401,.T.);
#8351=ORIENTED_EDGE('',*,*,#6402,.T.);
#8352=ORIENTED_EDGE('',*,*,#6403,.T.);
#8353=ORIENTED_EDGE('',*,*,#6401,.F.);
#8354=ORIENTED_EDGE('',*,*,#6404,.T.);
#8355=ORIENTED_EDGE('',*,*,#6405,.T.);
#8356=ORIENTED_EDGE('',*,*,#6406,.F.);
#8357=ORIENTED_EDGE('',*,*,#6407,.T.);
#8358=ORIENTED_EDGE('',*,*,#6408,.T.);
#8359=ORIENTED_EDGE('',*,*,#6409,.T.);
#8360=ORIENTED_EDGE('',*,*,#6410,.T.);
#8361=ORIENTED_EDGE('',*,*,#6408,.F.);
#8362=ORIENTED_EDGE('',*,*,#6411,.F.);
#8363=ORIENTED_EDGE('',*,*,#6412,.F.);
#8364=ORIENTED_EDGE('',*,*,#6413,.F.);
#8365=ORIENTED_EDGE('',*,*,#6414,.T.);
#8366=ORIENTED_EDGE('',*,*,#6415,.T.);
#8367=ORIENTED_EDGE('',*,*,#6416,.T.);
#8368=ORIENTED_EDGE('',*,*,#6417,.T.);
#8369=ORIENTED_EDGE('',*,*,#6415,.F.);
#8370=ORIENTED_EDGE('',*,*,#6418,.T.);
#8371=ORIENTED_EDGE('',*,*,#6419,.T.);
#8372=ORIENTED_EDGE('',*,*,#6420,.F.);
#8373=ORIENTED_EDGE('',*,*,#6421,.T.);
#8374=ORIENTED_EDGE('',*,*,#6422,.T.);
#8375=ORIENTED_EDGE('',*,*,#6423,.T.);
#8376=ORIENTED_EDGE('',*,*,#6424,.T.);
#8377=ORIENTED_EDGE('',*,*,#6422,.F.);
#8378=ORIENTED_EDGE('',*,*,#6425,.F.);
#8379=ORIENTED_EDGE('',*,*,#6426,.F.);
#8380=ORIENTED_EDGE('',*,*,#6427,.F.);
#8381=ORIENTED_EDGE('',*,*,#6428,.T.);
#8382=ORIENTED_EDGE('',*,*,#6429,.T.);
#8383=ORIENTED_EDGE('',*,*,#6430,.T.);
#8384=ORIENTED_EDGE('',*,*,#6431,.T.);
#8385=ORIENTED_EDGE('',*,*,#6429,.F.);
#8386=ORIENTED_EDGE('',*,*,#6432,.T.);
#8387=ORIENTED_EDGE('',*,*,#6433,.T.);
#8388=ORIENTED_EDGE('',*,*,#6434,.F.);
#8389=ORIENTED_EDGE('',*,*,#6435,.T.);
#8390=ORIENTED_EDGE('',*,*,#6436,.T.);
#8391=ORIENTED_EDGE('',*,*,#6437,.T.);
#8392=ORIENTED_EDGE('',*,*,#6438,.T.);
#8393=ORIENTED_EDGE('',*,*,#6436,.F.);
#8394=ORIENTED_EDGE('',*,*,#6439,.F.);
#8395=ORIENTED_EDGE('',*,*,#6440,.F.);
#8396=ORIENTED_EDGE('',*,*,#6441,.F.);
#8397=ORIENTED_EDGE('',*,*,#6442,.T.);
#8398=ORIENTED_EDGE('',*,*,#6443,.T.);
#8399=ORIENTED_EDGE('',*,*,#6444,.T.);
#8400=ORIENTED_EDGE('',*,*,#6445,.T.);
#8401=ORIENTED_EDGE('',*,*,#6443,.F.);
#8402=ORIENTED_EDGE('',*,*,#6446,.T.);
#8403=ORIENTED_EDGE('',*,*,#6447,.T.);
#8404=ORIENTED_EDGE('',*,*,#6448,.F.);
#8405=ORIENTED_EDGE('',*,*,#6449,.T.);
#8406=ORIENTED_EDGE('',*,*,#6450,.T.);
#8407=ORIENTED_EDGE('',*,*,#6451,.T.);
#8408=ORIENTED_EDGE('',*,*,#6452,.T.);
#8409=ORIENTED_EDGE('',*,*,#6450,.F.);
#8410=ORIENTED_EDGE('',*,*,#6453,.F.);
#8411=ORIENTED_EDGE('',*,*,#6454,.F.);
#8412=ORIENTED_EDGE('',*,*,#6455,.F.);
#8413=ORIENTED_EDGE('',*,*,#6456,.T.);
#8414=ORIENTED_EDGE('',*,*,#6457,.T.);
#8415=ORIENTED_EDGE('',*,*,#6458,.T.);
#8416=ORIENTED_EDGE('',*,*,#6459,.T.);
#8417=ORIENTED_EDGE('',*,*,#6457,.F.);
#8418=ORIENTED_EDGE('',*,*,#6460,.T.);
#8419=ORIENTED_EDGE('',*,*,#6461,.T.);
#8420=ORIENTED_EDGE('',*,*,#6462,.F.);
#8421=ORIENTED_EDGE('',*,*,#6463,.T.);
#8422=ORIENTED_EDGE('',*,*,#6464,.T.);
#8423=ORIENTED_EDGE('',*,*,#6465,.T.);
#8424=ORIENTED_EDGE('',*,*,#6466,.T.);
#8425=ORIENTED_EDGE('',*,*,#6464,.F.);
#8426=ORIENTED_EDGE('',*,*,#6467,.F.);
#8427=ORIENTED_EDGE('',*,*,#6468,.F.);
#8428=ORIENTED_EDGE('',*,*,#6469,.F.);
#8429=ORIENTED_EDGE('',*,*,#6470,.T.);
#8430=ORIENTED_EDGE('',*,*,#6471,.T.);
#8431=ORIENTED_EDGE('',*,*,#6472,.T.);
#8432=ORIENTED_EDGE('',*,*,#6473,.T.);
#8433=ORIENTED_EDGE('',*,*,#6471,.F.);
#8434=ORIENTED_EDGE('',*,*,#6474,.T.);
#8435=ORIENTED_EDGE('',*,*,#6475,.T.);
#8436=ORIENTED_EDGE('',*,*,#6476,.F.);
#8437=ORIENTED_EDGE('',*,*,#6477,.T.);
#8438=ORIENTED_EDGE('',*,*,#6478,.T.);
#8439=ORIENTED_EDGE('',*,*,#6479,.T.);
#8440=ORIENTED_EDGE('',*,*,#6480,.T.);
#8441=ORIENTED_EDGE('',*,*,#6478,.F.);
#8442=ORIENTED_EDGE('',*,*,#6481,.F.);
#8443=ORIENTED_EDGE('',*,*,#6482,.F.);
#8444=ORIENTED_EDGE('',*,*,#6483,.F.);
#8445=ORIENTED_EDGE('',*,*,#6484,.T.);
#8446=ORIENTED_EDGE('',*,*,#6485,.T.);
#8447=ORIENTED_EDGE('',*,*,#6486,.T.);
#8448=ORIENTED_EDGE('',*,*,#6487,.T.);
#8449=ORIENTED_EDGE('',*,*,#6485,.F.);
#8450=ORIENTED_EDGE('',*,*,#6488,.T.);
#8451=ORIENTED_EDGE('',*,*,#6489,.T.);
#8452=ORIENTED_EDGE('',*,*,#6490,.F.);
#8453=ORIENTED_EDGE('',*,*,#6491,.T.);
#8454=ORIENTED_EDGE('',*,*,#6492,.T.);
#8455=ORIENTED_EDGE('',*,*,#6493,.T.);
#8456=ORIENTED_EDGE('',*,*,#6494,.T.);
#8457=ORIENTED_EDGE('',*,*,#6492,.F.);
#8458=ORIENTED_EDGE('',*,*,#6495,.F.);
#8459=ORIENTED_EDGE('',*,*,#6496,.F.);
#8460=ORIENTED_EDGE('',*,*,#6497,.F.);
#8461=ORIENTED_EDGE('',*,*,#6498,.T.);
#8462=ORIENTED_EDGE('',*,*,#6499,.T.);
#8463=ORIENTED_EDGE('',*,*,#6500,.T.);
#8464=ORIENTED_EDGE('',*,*,#6501,.T.);
#8465=ORIENTED_EDGE('',*,*,#6499,.F.);
#8466=ORIENTED_EDGE('',*,*,#6502,.T.);
#8467=ORIENTED_EDGE('',*,*,#6503,.T.);
#8468=ORIENTED_EDGE('',*,*,#6504,.F.);
#8469=ORIENTED_EDGE('',*,*,#6505,.T.);
#8470=ORIENTED_EDGE('',*,*,#6506,.T.);
#8471=ORIENTED_EDGE('',*,*,#6507,.T.);
#8472=ORIENTED_EDGE('',*,*,#6508,.T.);
#8473=ORIENTED_EDGE('',*,*,#6506,.F.);
#8474=ORIENTED_EDGE('',*,*,#6509,.F.);
#8475=ORIENTED_EDGE('',*,*,#6510,.F.);
#8476=ORIENTED_EDGE('',*,*,#6511,.F.);
#8477=ORIENTED_EDGE('',*,*,#6512,.T.);
#8478=ORIENTED_EDGE('',*,*,#6513,.T.);
#8479=ORIENTED_EDGE('',*,*,#6514,.T.);
#8480=ORIENTED_EDGE('',*,*,#6515,.T.);
#8481=ORIENTED_EDGE('',*,*,#6513,.F.);
#8482=ORIENTED_EDGE('',*,*,#6516,.T.);
#8483=ORIENTED_EDGE('',*,*,#6517,.T.);
#8484=ORIENTED_EDGE('',*,*,#6518,.F.);
#8485=ORIENTED_EDGE('',*,*,#6519,.F.);
#8486=ORIENTED_EDGE('',*,*,#6258,.T.);
#8487=ORIENTED_EDGE('',*,*,#6520,.F.);
#8488=ORIENTED_EDGE('',*,*,#6521,.F.);
#8489=ORIENTED_EDGE('',*,*,#6522,.T.);
#8490=ORIENTED_EDGE('',*,*,#6521,.T.);
#8491=ORIENTED_EDGE('',*,*,#6523,.F.);
#8492=ORIENTED_EDGE('',*,*,#6524,.F.);
#8493=ORIENTED_EDGE('',*,*,#6525,.T.);
#8494=ORIENTED_EDGE('',*,*,#6524,.T.);
#8495=ORIENTED_EDGE('',*,*,#6526,.F.);
#8496=ORIENTED_EDGE('',*,*,#6265,.F.);
#8497=ORIENTED_EDGE('',*,*,#6527,.F.);
#8498=ORIENTED_EDGE('',*,*,#6272,.T.);
#8499=ORIENTED_EDGE('',*,*,#6528,.F.);
#8500=ORIENTED_EDGE('',*,*,#6529,.F.);
#8501=ORIENTED_EDGE('',*,*,#6530,.T.);
#8502=ORIENTED_EDGE('',*,*,#6529,.T.);
#8503=ORIENTED_EDGE('',*,*,#6531,.F.);
#8504=ORIENTED_EDGE('',*,*,#6532,.F.);
#8505=ORIENTED_EDGE('',*,*,#6533,.T.);
#8506=ORIENTED_EDGE('',*,*,#6532,.T.);
#8507=ORIENTED_EDGE('',*,*,#6534,.F.);
#8508=ORIENTED_EDGE('',*,*,#6279,.F.);
#8509=ORIENTED_EDGE('',*,*,#6535,.F.);
#8510=ORIENTED_EDGE('',*,*,#6286,.T.);
#8511=ORIENTED_EDGE('',*,*,#6536,.F.);
#8512=ORIENTED_EDGE('',*,*,#6537,.F.);
#8513=ORIENTED_EDGE('',*,*,#6538,.T.);
#8514=ORIENTED_EDGE('',*,*,#6537,.T.);
#8515=ORIENTED_EDGE('',*,*,#6539,.F.);
#8516=ORIENTED_EDGE('',*,*,#6540,.F.);
#8517=ORIENTED_EDGE('',*,*,#6541,.T.);
#8518=ORIENTED_EDGE('',*,*,#6540,.T.);
#8519=ORIENTED_EDGE('',*,*,#6542,.F.);
#8520=ORIENTED_EDGE('',*,*,#6293,.F.);
#8521=ORIENTED_EDGE('',*,*,#6543,.F.);
#8522=ORIENTED_EDGE('',*,*,#6300,.T.);
#8523=ORIENTED_EDGE('',*,*,#6544,.F.);
#8524=ORIENTED_EDGE('',*,*,#6545,.F.);
#8525=ORIENTED_EDGE('',*,*,#6546,.T.);
#8526=ORIENTED_EDGE('',*,*,#6545,.T.);
#8527=ORIENTED_EDGE('',*,*,#6547,.F.);
#8528=ORIENTED_EDGE('',*,*,#6548,.F.);
#8529=ORIENTED_EDGE('',*,*,#6549,.T.);
#8530=ORIENTED_EDGE('',*,*,#6548,.T.);
#8531=ORIENTED_EDGE('',*,*,#6550,.F.);
#8532=ORIENTED_EDGE('',*,*,#6307,.F.);
#8533=ORIENTED_EDGE('',*,*,#6551,.F.);
#8534=ORIENTED_EDGE('',*,*,#6314,.T.);
#8535=ORIENTED_EDGE('',*,*,#6552,.F.);
#8536=ORIENTED_EDGE('',*,*,#6553,.F.);
#8537=ORIENTED_EDGE('',*,*,#6554,.T.);
#8538=ORIENTED_EDGE('',*,*,#6553,.T.);
#8539=ORIENTED_EDGE('',*,*,#6555,.F.);
#8540=ORIENTED_EDGE('',*,*,#6556,.F.);
#8541=ORIENTED_EDGE('',*,*,#6557,.T.);
#8542=ORIENTED_EDGE('',*,*,#6556,.T.);
#8543=ORIENTED_EDGE('',*,*,#6558,.F.);
#8544=ORIENTED_EDGE('',*,*,#6321,.F.);
#8545=ORIENTED_EDGE('',*,*,#6559,.F.);
#8546=ORIENTED_EDGE('',*,*,#6328,.T.);
#8547=ORIENTED_EDGE('',*,*,#6560,.F.);
#8548=ORIENTED_EDGE('',*,*,#6561,.F.);
#8549=ORIENTED_EDGE('',*,*,#6562,.T.);
#8550=ORIENTED_EDGE('',*,*,#6561,.T.);
#8551=ORIENTED_EDGE('',*,*,#6563,.F.);
#8552=ORIENTED_EDGE('',*,*,#6564,.F.);
#8553=ORIENTED_EDGE('',*,*,#6565,.T.);
#8554=ORIENTED_EDGE('',*,*,#6564,.T.);
#8555=ORIENTED_EDGE('',*,*,#6566,.F.);
#8556=ORIENTED_EDGE('',*,*,#6335,.F.);
#8557=ORIENTED_EDGE('',*,*,#6567,.F.);
#8558=ORIENTED_EDGE('',*,*,#6342,.T.);
#8559=ORIENTED_EDGE('',*,*,#6568,.F.);
#8560=ORIENTED_EDGE('',*,*,#6569,.F.);
#8561=ORIENTED_EDGE('',*,*,#6570,.T.);
#8562=ORIENTED_EDGE('',*,*,#6569,.T.);
#8563=ORIENTED_EDGE('',*,*,#6571,.F.);
#8564=ORIENTED_EDGE('',*,*,#6572,.F.);
#8565=ORIENTED_EDGE('',*,*,#6573,.T.);
#8566=ORIENTED_EDGE('',*,*,#6572,.T.);
#8567=ORIENTED_EDGE('',*,*,#6574,.F.);
#8568=ORIENTED_EDGE('',*,*,#6349,.F.);
#8569=ORIENTED_EDGE('',*,*,#6575,.F.);
#8570=ORIENTED_EDGE('',*,*,#6356,.T.);
#8571=ORIENTED_EDGE('',*,*,#6576,.F.);
#8572=ORIENTED_EDGE('',*,*,#6577,.F.);
#8573=ORIENTED_EDGE('',*,*,#6578,.T.);
#8574=ORIENTED_EDGE('',*,*,#6577,.T.);
#8575=ORIENTED_EDGE('',*,*,#6579,.F.);
#8576=ORIENTED_EDGE('',*,*,#6580,.F.);
#8577=ORIENTED_EDGE('',*,*,#6581,.T.);
#8578=ORIENTED_EDGE('',*,*,#6580,.T.);
#8579=ORIENTED_EDGE('',*,*,#6582,.F.);
#8580=ORIENTED_EDGE('',*,*,#6363,.F.);
#8581=ORIENTED_EDGE('',*,*,#6583,.F.);
#8582=ORIENTED_EDGE('',*,*,#6370,.T.);
#8583=ORIENTED_EDGE('',*,*,#6584,.F.);
#8584=ORIENTED_EDGE('',*,*,#6585,.F.);
#8585=ORIENTED_EDGE('',*,*,#6586,.T.);
#8586=ORIENTED_EDGE('',*,*,#6585,.T.);
#8587=ORIENTED_EDGE('',*,*,#6587,.F.);
#8588=ORIENTED_EDGE('',*,*,#6588,.F.);
#8589=ORIENTED_EDGE('',*,*,#6589,.T.);
#8590=ORIENTED_EDGE('',*,*,#6588,.T.);
#8591=ORIENTED_EDGE('',*,*,#6590,.F.);
#8592=ORIENTED_EDGE('',*,*,#6377,.F.);
#8593=ORIENTED_EDGE('',*,*,#6591,.F.);
#8594=ORIENTED_EDGE('',*,*,#6384,.T.);
#8595=ORIENTED_EDGE('',*,*,#6592,.F.);
#8596=ORIENTED_EDGE('',*,*,#6593,.F.);
#8597=ORIENTED_EDGE('',*,*,#6594,.T.);
#8598=ORIENTED_EDGE('',*,*,#6593,.T.);
#8599=ORIENTED_EDGE('',*,*,#6595,.F.);
#8600=ORIENTED_EDGE('',*,*,#6596,.F.);
#8601=ORIENTED_EDGE('',*,*,#6597,.T.);
#8602=ORIENTED_EDGE('',*,*,#6596,.T.);
#8603=ORIENTED_EDGE('',*,*,#6598,.F.);
#8604=ORIENTED_EDGE('',*,*,#6391,.F.);
#8605=ORIENTED_EDGE('',*,*,#6599,.F.);
#8606=ORIENTED_EDGE('',*,*,#6398,.T.);
#8607=ORIENTED_EDGE('',*,*,#6600,.F.);
#8608=ORIENTED_EDGE('',*,*,#6601,.F.);
#8609=ORIENTED_EDGE('',*,*,#6602,.T.);
#8610=ORIENTED_EDGE('',*,*,#6601,.T.);
#8611=ORIENTED_EDGE('',*,*,#6603,.F.);
#8612=ORIENTED_EDGE('',*,*,#6604,.F.);
#8613=ORIENTED_EDGE('',*,*,#6605,.T.);
#8614=ORIENTED_EDGE('',*,*,#6604,.T.);
#8615=ORIENTED_EDGE('',*,*,#6606,.F.);
#8616=ORIENTED_EDGE('',*,*,#6405,.F.);
#8617=ORIENTED_EDGE('',*,*,#6607,.F.);
#8618=ORIENTED_EDGE('',*,*,#6412,.T.);
#8619=ORIENTED_EDGE('',*,*,#6608,.F.);
#8620=ORIENTED_EDGE('',*,*,#6609,.F.);
#8621=ORIENTED_EDGE('',*,*,#6610,.T.);
#8622=ORIENTED_EDGE('',*,*,#6609,.T.);
#8623=ORIENTED_EDGE('',*,*,#6611,.F.);
#8624=ORIENTED_EDGE('',*,*,#6612,.F.);
#8625=ORIENTED_EDGE('',*,*,#6613,.T.);
#8626=ORIENTED_EDGE('',*,*,#6612,.T.);
#8627=ORIENTED_EDGE('',*,*,#6614,.F.);
#8628=ORIENTED_EDGE('',*,*,#6419,.F.);
#8629=ORIENTED_EDGE('',*,*,#6615,.F.);
#8630=ORIENTED_EDGE('',*,*,#6426,.T.);
#8631=ORIENTED_EDGE('',*,*,#6616,.F.);
#8632=ORIENTED_EDGE('',*,*,#6617,.F.);
#8633=ORIENTED_EDGE('',*,*,#6618,.T.);
#8634=ORIENTED_EDGE('',*,*,#6617,.T.);
#8635=ORIENTED_EDGE('',*,*,#6619,.F.);
#8636=ORIENTED_EDGE('',*,*,#6620,.F.);
#8637=ORIENTED_EDGE('',*,*,#6621,.T.);
#8638=ORIENTED_EDGE('',*,*,#6620,.T.);
#8639=ORIENTED_EDGE('',*,*,#6622,.F.);
#8640=ORIENTED_EDGE('',*,*,#6433,.F.);
#8641=ORIENTED_EDGE('',*,*,#6623,.F.);
#8642=ORIENTED_EDGE('',*,*,#6440,.T.);
#8643=ORIENTED_EDGE('',*,*,#6624,.F.);
#8644=ORIENTED_EDGE('',*,*,#6625,.F.);
#8645=ORIENTED_EDGE('',*,*,#6626,.T.);
#8646=ORIENTED_EDGE('',*,*,#6625,.T.);
#8647=ORIENTED_EDGE('',*,*,#6627,.F.);
#8648=ORIENTED_EDGE('',*,*,#6628,.F.);
#8649=ORIENTED_EDGE('',*,*,#6629,.T.);
#8650=ORIENTED_EDGE('',*,*,#6628,.T.);
#8651=ORIENTED_EDGE('',*,*,#6630,.F.);
#8652=ORIENTED_EDGE('',*,*,#6447,.F.);
#8653=ORIENTED_EDGE('',*,*,#6631,.F.);
#8654=ORIENTED_EDGE('',*,*,#6454,.T.);
#8655=ORIENTED_EDGE('',*,*,#6632,.F.);
#8656=ORIENTED_EDGE('',*,*,#6633,.F.);
#8657=ORIENTED_EDGE('',*,*,#6634,.T.);
#8658=ORIENTED_EDGE('',*,*,#6633,.T.);
#8659=ORIENTED_EDGE('',*,*,#6635,.F.);
#8660=ORIENTED_EDGE('',*,*,#6636,.F.);
#8661=ORIENTED_EDGE('',*,*,#6637,.T.);
#8662=ORIENTED_EDGE('',*,*,#6636,.T.);
#8663=ORIENTED_EDGE('',*,*,#6638,.F.);
#8664=ORIENTED_EDGE('',*,*,#6461,.F.);
#8665=ORIENTED_EDGE('',*,*,#6639,.F.);
#8666=ORIENTED_EDGE('',*,*,#6468,.T.);
#8667=ORIENTED_EDGE('',*,*,#6640,.F.);
#8668=ORIENTED_EDGE('',*,*,#6641,.F.);
#8669=ORIENTED_EDGE('',*,*,#6642,.T.);
#8670=ORIENTED_EDGE('',*,*,#6641,.T.);
#8671=ORIENTED_EDGE('',*,*,#6643,.F.);
#8672=ORIENTED_EDGE('',*,*,#6644,.F.);
#8673=ORIENTED_EDGE('',*,*,#6645,.T.);
#8674=ORIENTED_EDGE('',*,*,#6644,.T.);
#8675=ORIENTED_EDGE('',*,*,#6646,.F.);
#8676=ORIENTED_EDGE('',*,*,#6475,.F.);
#8677=ORIENTED_EDGE('',*,*,#6647,.F.);
#8678=ORIENTED_EDGE('',*,*,#6482,.T.);
#8679=ORIENTED_EDGE('',*,*,#6648,.F.);
#8680=ORIENTED_EDGE('',*,*,#6649,.F.);
#8681=ORIENTED_EDGE('',*,*,#6650,.T.);
#8682=ORIENTED_EDGE('',*,*,#6649,.T.);
#8683=ORIENTED_EDGE('',*,*,#6651,.F.);
#8684=ORIENTED_EDGE('',*,*,#6652,.F.);
#8685=ORIENTED_EDGE('',*,*,#6653,.T.);
#8686=ORIENTED_EDGE('',*,*,#6652,.T.);
#8687=ORIENTED_EDGE('',*,*,#6654,.F.);
#8688=ORIENTED_EDGE('',*,*,#6489,.F.);
#8689=ORIENTED_EDGE('',*,*,#6655,.F.);
#8690=ORIENTED_EDGE('',*,*,#6496,.T.);
#8691=ORIENTED_EDGE('',*,*,#6656,.F.);
#8692=ORIENTED_EDGE('',*,*,#6657,.F.);
#8693=ORIENTED_EDGE('',*,*,#6658,.T.);
#8694=ORIENTED_EDGE('',*,*,#6657,.T.);
#8695=ORIENTED_EDGE('',*,*,#6659,.F.);
#8696=ORIENTED_EDGE('',*,*,#6660,.F.);
#8697=ORIENTED_EDGE('',*,*,#6661,.T.);
#8698=ORIENTED_EDGE('',*,*,#6660,.T.);
#8699=ORIENTED_EDGE('',*,*,#6662,.F.);
#8700=ORIENTED_EDGE('',*,*,#6503,.F.);
#8701=ORIENTED_EDGE('',*,*,#6663,.F.);
#8702=ORIENTED_EDGE('',*,*,#6510,.T.);
#8703=ORIENTED_EDGE('',*,*,#6664,.F.);
#8704=ORIENTED_EDGE('',*,*,#6665,.F.);
#8705=ORIENTED_EDGE('',*,*,#6666,.T.);
#8706=ORIENTED_EDGE('',*,*,#6665,.T.);
#8707=ORIENTED_EDGE('',*,*,#6667,.F.);
#8708=ORIENTED_EDGE('',*,*,#6668,.F.);
#8709=ORIENTED_EDGE('',*,*,#6669,.T.);
#8710=ORIENTED_EDGE('',*,*,#6668,.T.);
#8711=ORIENTED_EDGE('',*,*,#6670,.F.);
#8712=ORIENTED_EDGE('',*,*,#6517,.F.);
#8713=ORIENTED_EDGE('',*,*,#6269,.F.);
#8714=ORIENTED_EDGE('',*,*,#6273,.T.);
#8715=ORIENTED_EDGE('',*,*,#6527,.T.);
#8716=ORIENTED_EDGE('',*,*,#6530,.F.);
#8717=ORIENTED_EDGE('',*,*,#6533,.F.);
#8718=ORIENTED_EDGE('',*,*,#6278,.F.);
#8719=ORIENTED_EDGE('',*,*,#6274,.F.);
#8720=ORIENTED_EDGE('',*,*,#6671,.F.);
#8721=ORIENTED_EDGE('',*,*,#6283,.F.);
#8722=ORIENTED_EDGE('',*,*,#6287,.T.);
#8723=ORIENTED_EDGE('',*,*,#6535,.T.);
#8724=ORIENTED_EDGE('',*,*,#6538,.F.);
#8725=ORIENTED_EDGE('',*,*,#6541,.F.);
#8726=ORIENTED_EDGE('',*,*,#6292,.F.);
#8727=ORIENTED_EDGE('',*,*,#6288,.F.);
#8728=ORIENTED_EDGE('',*,*,#6672,.F.);
#8729=ORIENTED_EDGE('',*,*,#6297,.F.);
#8730=ORIENTED_EDGE('',*,*,#6301,.T.);
#8731=ORIENTED_EDGE('',*,*,#6543,.T.);
#8732=ORIENTED_EDGE('',*,*,#6546,.F.);
#8733=ORIENTED_EDGE('',*,*,#6549,.F.);
#8734=ORIENTED_EDGE('',*,*,#6306,.F.);
#8735=ORIENTED_EDGE('',*,*,#6302,.F.);
#8736=ORIENTED_EDGE('',*,*,#6673,.F.);
#8737=ORIENTED_EDGE('',*,*,#6311,.F.);
#8738=ORIENTED_EDGE('',*,*,#6315,.T.);
#8739=ORIENTED_EDGE('',*,*,#6551,.T.);
#8740=ORIENTED_EDGE('',*,*,#6554,.F.);
#8741=ORIENTED_EDGE('',*,*,#6557,.F.);
#8742=ORIENTED_EDGE('',*,*,#6320,.F.);
#8743=ORIENTED_EDGE('',*,*,#6316,.F.);
#8744=ORIENTED_EDGE('',*,*,#6674,.F.);
#8745=ORIENTED_EDGE('',*,*,#6325,.F.);
#8746=ORIENTED_EDGE('',*,*,#6329,.T.);
#8747=ORIENTED_EDGE('',*,*,#6559,.T.);
#8748=ORIENTED_EDGE('',*,*,#6562,.F.);
#8749=ORIENTED_EDGE('',*,*,#6565,.F.);
#8750=ORIENTED_EDGE('',*,*,#6334,.F.);
#8751=ORIENTED_EDGE('',*,*,#6330,.F.);
#8752=ORIENTED_EDGE('',*,*,#6675,.F.);
#8753=ORIENTED_EDGE('',*,*,#6339,.F.);
#8754=ORIENTED_EDGE('',*,*,#6343,.T.);
#8755=ORIENTED_EDGE('',*,*,#6567,.T.);
#8756=ORIENTED_EDGE('',*,*,#6570,.F.);
#8757=ORIENTED_EDGE('',*,*,#6573,.F.);
#8758=ORIENTED_EDGE('',*,*,#6348,.F.);
#8759=ORIENTED_EDGE('',*,*,#6344,.F.);
#8760=ORIENTED_EDGE('',*,*,#6676,.F.);
#8761=ORIENTED_EDGE('',*,*,#6353,.F.);
#8762=ORIENTED_EDGE('',*,*,#6357,.T.);
#8763=ORIENTED_EDGE('',*,*,#6575,.T.);
#8764=ORIENTED_EDGE('',*,*,#6578,.F.);
#8765=ORIENTED_EDGE('',*,*,#6581,.F.);
#8766=ORIENTED_EDGE('',*,*,#6362,.F.);
#8767=ORIENTED_EDGE('',*,*,#6358,.F.);
#8768=ORIENTED_EDGE('',*,*,#6677,.F.);
#8769=ORIENTED_EDGE('',*,*,#6367,.F.);
#8770=ORIENTED_EDGE('',*,*,#6371,.T.);
#8771=ORIENTED_EDGE('',*,*,#6583,.T.);
#8772=ORIENTED_EDGE('',*,*,#6586,.F.);
#8773=ORIENTED_EDGE('',*,*,#6589,.F.);
#8774=ORIENTED_EDGE('',*,*,#6376,.F.);
#8775=ORIENTED_EDGE('',*,*,#6372,.F.);
#8776=ORIENTED_EDGE('',*,*,#6678,.F.);
#8777=ORIENTED_EDGE('',*,*,#6381,.F.);
#8778=ORIENTED_EDGE('',*,*,#6385,.T.);
#8779=ORIENTED_EDGE('',*,*,#6591,.T.);
#8780=ORIENTED_EDGE('',*,*,#6594,.F.);
#8781=ORIENTED_EDGE('',*,*,#6597,.F.);
#8782=ORIENTED_EDGE('',*,*,#6390,.F.);
#8783=ORIENTED_EDGE('',*,*,#6386,.F.);
#8784=ORIENTED_EDGE('',*,*,#6679,.F.);
#8785=ORIENTED_EDGE('',*,*,#6395,.F.);
#8786=ORIENTED_EDGE('',*,*,#6399,.T.);
#8787=ORIENTED_EDGE('',*,*,#6599,.T.);
#8788=ORIENTED_EDGE('',*,*,#6602,.F.);
#8789=ORIENTED_EDGE('',*,*,#6605,.F.);
#8790=ORIENTED_EDGE('',*,*,#6404,.F.);
#8791=ORIENTED_EDGE('',*,*,#6400,.F.);
#8792=ORIENTED_EDGE('',*,*,#6680,.F.);
#8793=ORIENTED_EDGE('',*,*,#6409,.F.);
#8794=ORIENTED_EDGE('',*,*,#6413,.T.);
#8795=ORIENTED_EDGE('',*,*,#6607,.T.);
#8796=ORIENTED_EDGE('',*,*,#6610,.F.);
#8797=ORIENTED_EDGE('',*,*,#6613,.F.);
#8798=ORIENTED_EDGE('',*,*,#6418,.F.);
#8799=ORIENTED_EDGE('',*,*,#6414,.F.);
#8800=ORIENTED_EDGE('',*,*,#6681,.F.);
#8801=ORIENTED_EDGE('',*,*,#6423,.F.);
#8802=ORIENTED_EDGE('',*,*,#6427,.T.);
#8803=ORIENTED_EDGE('',*,*,#6615,.T.);
#8804=ORIENTED_EDGE('',*,*,#6618,.F.);
#8805=ORIENTED_EDGE('',*,*,#6621,.F.);
#8806=ORIENTED_EDGE('',*,*,#6432,.F.);
#8807=ORIENTED_EDGE('',*,*,#6428,.F.);
#8808=ORIENTED_EDGE('',*,*,#6682,.F.);
#8809=ORIENTED_EDGE('',*,*,#6437,.F.);
#8810=ORIENTED_EDGE('',*,*,#6441,.T.);
#8811=ORIENTED_EDGE('',*,*,#6623,.T.);
#8812=ORIENTED_EDGE('',*,*,#6626,.F.);
#8813=ORIENTED_EDGE('',*,*,#6629,.F.);
#8814=ORIENTED_EDGE('',*,*,#6446,.F.);
#8815=ORIENTED_EDGE('',*,*,#6442,.F.);
#8816=ORIENTED_EDGE('',*,*,#6683,.F.);
#8817=ORIENTED_EDGE('',*,*,#6451,.F.);
#8818=ORIENTED_EDGE('',*,*,#6455,.T.);
#8819=ORIENTED_EDGE('',*,*,#6631,.T.);
#8820=ORIENTED_EDGE('',*,*,#6634,.F.);
#8821=ORIENTED_EDGE('',*,*,#6637,.F.);
#8822=ORIENTED_EDGE('',*,*,#6460,.F.);
#8823=ORIENTED_EDGE('',*,*,#6456,.F.);
#8824=ORIENTED_EDGE('',*,*,#6684,.F.);
#8825=ORIENTED_EDGE('',*,*,#6465,.F.);
#8826=ORIENTED_EDGE('',*,*,#6469,.T.);
#8827=ORIENTED_EDGE('',*,*,#6639,.T.);
#8828=ORIENTED_EDGE('',*,*,#6642,.F.);
#8829=ORIENTED_EDGE('',*,*,#6645,.F.);
#8830=ORIENTED_EDGE('',*,*,#6474,.F.);
#8831=ORIENTED_EDGE('',*,*,#6470,.F.);
#8832=ORIENTED_EDGE('',*,*,#6685,.F.);
#8833=ORIENTED_EDGE('',*,*,#6479,.F.);
#8834=ORIENTED_EDGE('',*,*,#6483,.T.);
#8835=ORIENTED_EDGE('',*,*,#6647,.T.);
#8836=ORIENTED_EDGE('',*,*,#6650,.F.);
#8837=ORIENTED_EDGE('',*,*,#6653,.F.);
#8838=ORIENTED_EDGE('',*,*,#6488,.F.);
#8839=ORIENTED_EDGE('',*,*,#6484,.F.);
#8840=ORIENTED_EDGE('',*,*,#6686,.F.);
#8841=ORIENTED_EDGE('',*,*,#6493,.F.);
#8842=ORIENTED_EDGE('',*,*,#6497,.T.);
#8843=ORIENTED_EDGE('',*,*,#6655,.T.);
#8844=ORIENTED_EDGE('',*,*,#6658,.F.);
#8845=ORIENTED_EDGE('',*,*,#6661,.F.);
#8846=ORIENTED_EDGE('',*,*,#6502,.F.);
#8847=ORIENTED_EDGE('',*,*,#6498,.F.);
#8848=ORIENTED_EDGE('',*,*,#6687,.F.);
#8849=ORIENTED_EDGE('',*,*,#6507,.F.);
#8850=ORIENTED_EDGE('',*,*,#6511,.T.);
#8851=ORIENTED_EDGE('',*,*,#6663,.T.);
#8852=ORIENTED_EDGE('',*,*,#6666,.F.);
#8853=ORIENTED_EDGE('',*,*,#6669,.F.);
#8854=ORIENTED_EDGE('',*,*,#6516,.F.);
#8855=ORIENTED_EDGE('',*,*,#6512,.F.);
#8856=ORIENTED_EDGE('',*,*,#6688,.F.);
#8857=ORIENTED_EDGE('',*,*,#6689,.F.);
#8858=ORIENTED_EDGE('',*,*,#6690,.T.);
#8859=ORIENTED_EDGE('',*,*,#6691,.T.);
#8860=ORIENTED_EDGE('',*,*,#6692,.F.);
#8861=ORIENTED_EDGE('',*,*,#6693,.F.);
#8862=ORIENTED_EDGE('',*,*,#6694,.F.);
#8863=ORIENTED_EDGE('',*,*,#6695,.F.);
#8864=ORIENTED_EDGE('',*,*,#6696,.F.);
#8865=ORIENTED_EDGE('',*,*,#6255,.F.);
#8866=ORIENTED_EDGE('',*,*,#6259,.T.);
#8867=ORIENTED_EDGE('',*,*,#6519,.T.);
#8868=ORIENTED_EDGE('',*,*,#6522,.F.);
#8869=ORIENTED_EDGE('',*,*,#6525,.F.);
#8870=ORIENTED_EDGE('',*,*,#6264,.F.);
#8871=ORIENTED_EDGE('',*,*,#6260,.F.);
#8872=ORIENTED_EDGE('',*,*,#6697,.F.);
#8873=ORIENTED_EDGE('',*,*,#6252,.T.);
#8874=ORIENTED_EDGE('',*,*,#6698,.T.);
#8875=ORIENTED_EDGE('',*,*,#6699,.F.);
#8876=ORIENTED_EDGE('',*,*,#6700,.T.);
#8877=ORIENTED_EDGE('',*,*,#6701,.T.);
#8878=ORIENTED_EDGE('',*,*,#6702,.T.);
#8879=ORIENTED_EDGE('',*,*,#6703,.T.);
#8880=ORIENTED_EDGE('',*,*,#6704,.T.);
#8881=ORIENTED_EDGE('',*,*,#6705,.F.);
#8882=ORIENTED_EDGE('',*,*,#6706,.T.);
#8883=ORIENTED_EDGE('',*,*,#6514,.F.);
#8884=ORIENTED_EDGE('',*,*,#6518,.T.);
#8885=ORIENTED_EDGE('',*,*,#6670,.T.);
#8886=ORIENTED_EDGE('',*,*,#6667,.T.);
#8887=ORIENTED_EDGE('',*,*,#6664,.T.);
#8888=ORIENTED_EDGE('',*,*,#6509,.T.);
#8889=ORIENTED_EDGE('',*,*,#6505,.F.);
#8890=ORIENTED_EDGE('',*,*,#6707,.T.);
#8891=ORIENTED_EDGE('',*,*,#6500,.F.);
#8892=ORIENTED_EDGE('',*,*,#6504,.T.);
#8893=ORIENTED_EDGE('',*,*,#6662,.T.);
#8894=ORIENTED_EDGE('',*,*,#6659,.T.);
#8895=ORIENTED_EDGE('',*,*,#6656,.T.);
#8896=ORIENTED_EDGE('',*,*,#6495,.T.);
#8897=ORIENTED_EDGE('',*,*,#6491,.F.);
#8898=ORIENTED_EDGE('',*,*,#6708,.T.);
#8899=ORIENTED_EDGE('',*,*,#6486,.F.);
#8900=ORIENTED_EDGE('',*,*,#6490,.T.);
#8901=ORIENTED_EDGE('',*,*,#6654,.T.);
#8902=ORIENTED_EDGE('',*,*,#6651,.T.);
#8903=ORIENTED_EDGE('',*,*,#6648,.T.);
#8904=ORIENTED_EDGE('',*,*,#6481,.T.);
#8905=ORIENTED_EDGE('',*,*,#6477,.F.);
#8906=ORIENTED_EDGE('',*,*,#6709,.T.);
#8907=ORIENTED_EDGE('',*,*,#6472,.F.);
#8908=ORIENTED_EDGE('',*,*,#6476,.T.);
#8909=ORIENTED_EDGE('',*,*,#6646,.T.);
#8910=ORIENTED_EDGE('',*,*,#6643,.T.);
#8911=ORIENTED_EDGE('',*,*,#6640,.T.);
#8912=ORIENTED_EDGE('',*,*,#6467,.T.);
#8913=ORIENTED_EDGE('',*,*,#6463,.F.);
#8914=ORIENTED_EDGE('',*,*,#6710,.T.);
#8915=ORIENTED_EDGE('',*,*,#6458,.F.);
#8916=ORIENTED_EDGE('',*,*,#6462,.T.);
#8917=ORIENTED_EDGE('',*,*,#6638,.T.);
#8918=ORIENTED_EDGE('',*,*,#6635,.T.);
#8919=ORIENTED_EDGE('',*,*,#6632,.T.);
#8920=ORIENTED_EDGE('',*,*,#6453,.T.);
#8921=ORIENTED_EDGE('',*,*,#6449,.F.);
#8922=ORIENTED_EDGE('',*,*,#6711,.T.);
#8923=ORIENTED_EDGE('',*,*,#6444,.F.);
#8924=ORIENTED_EDGE('',*,*,#6448,.T.);
#8925=ORIENTED_EDGE('',*,*,#6630,.T.);
#8926=ORIENTED_EDGE('',*,*,#6627,.T.);
#8927=ORIENTED_EDGE('',*,*,#6624,.T.);
#8928=ORIENTED_EDGE('',*,*,#6439,.T.);
#8929=ORIENTED_EDGE('',*,*,#6435,.F.);
#8930=ORIENTED_EDGE('',*,*,#6712,.T.);
#8931=ORIENTED_EDGE('',*,*,#6430,.F.);
#8932=ORIENTED_EDGE('',*,*,#6434,.T.);
#8933=ORIENTED_EDGE('',*,*,#6622,.T.);
#8934=ORIENTED_EDGE('',*,*,#6619,.T.);
#8935=ORIENTED_EDGE('',*,*,#6616,.T.);
#8936=ORIENTED_EDGE('',*,*,#6425,.T.);
#8937=ORIENTED_EDGE('',*,*,#6421,.F.);
#8938=ORIENTED_EDGE('',*,*,#6713,.T.);
#8939=ORIENTED_EDGE('',*,*,#6416,.F.);
#8940=ORIENTED_EDGE('',*,*,#6420,.T.);
#8941=ORIENTED_EDGE('',*,*,#6614,.T.);
#8942=ORIENTED_EDGE('',*,*,#6611,.T.);
#8943=ORIENTED_EDGE('',*,*,#6608,.T.);
#8944=ORIENTED_EDGE('',*,*,#6411,.T.);
#8945=ORIENTED_EDGE('',*,*,#6407,.F.);
#8946=ORIENTED_EDGE('',*,*,#6714,.T.);
#8947=ORIENTED_EDGE('',*,*,#6402,.F.);
#8948=ORIENTED_EDGE('',*,*,#6406,.T.);
#8949=ORIENTED_EDGE('',*,*,#6606,.T.);
#8950=ORIENTED_EDGE('',*,*,#6603,.T.);
#8951=ORIENTED_EDGE('',*,*,#6600,.T.);
#8952=ORIENTED_EDGE('',*,*,#6397,.T.);
#8953=ORIENTED_EDGE('',*,*,#6393,.F.);
#8954=ORIENTED_EDGE('',*,*,#6715,.T.);
#8955=ORIENTED_EDGE('',*,*,#6388,.F.);
#8956=ORIENTED_EDGE('',*,*,#6392,.T.);
#8957=ORIENTED_EDGE('',*,*,#6598,.T.);
#8958=ORIENTED_EDGE('',*,*,#6595,.T.);
#8959=ORIENTED_EDGE('',*,*,#6592,.T.);
#8960=ORIENTED_EDGE('',*,*,#6383,.T.);
#8961=ORIENTED_EDGE('',*,*,#6379,.F.);
#8962=ORIENTED_EDGE('',*,*,#6716,.T.);
#8963=ORIENTED_EDGE('',*,*,#6374,.F.);
#8964=ORIENTED_EDGE('',*,*,#6378,.T.);
#8965=ORIENTED_EDGE('',*,*,#6590,.T.);
#8966=ORIENTED_EDGE('',*,*,#6587,.T.);
#8967=ORIENTED_EDGE('',*,*,#6584,.T.);
#8968=ORIENTED_EDGE('',*,*,#6369,.T.);
#8969=ORIENTED_EDGE('',*,*,#6365,.F.);
#8970=ORIENTED_EDGE('',*,*,#6717,.T.);
#8971=ORIENTED_EDGE('',*,*,#6360,.F.);
#8972=ORIENTED_EDGE('',*,*,#6364,.T.);
#8973=ORIENTED_EDGE('',*,*,#6582,.T.);
#8974=ORIENTED_EDGE('',*,*,#6579,.T.);
#8975=ORIENTED_EDGE('',*,*,#6576,.T.);
#8976=ORIENTED_EDGE('',*,*,#6355,.T.);
#8977=ORIENTED_EDGE('',*,*,#6351,.F.);
#8978=ORIENTED_EDGE('',*,*,#6718,.T.);
#8979=ORIENTED_EDGE('',*,*,#6346,.F.);
#8980=ORIENTED_EDGE('',*,*,#6350,.T.);
#8981=ORIENTED_EDGE('',*,*,#6574,.T.);
#8982=ORIENTED_EDGE('',*,*,#6571,.T.);
#8983=ORIENTED_EDGE('',*,*,#6568,.T.);
#8984=ORIENTED_EDGE('',*,*,#6341,.T.);
#8985=ORIENTED_EDGE('',*,*,#6337,.F.);
#8986=ORIENTED_EDGE('',*,*,#6719,.T.);
#8987=ORIENTED_EDGE('',*,*,#6332,.F.);
#8988=ORIENTED_EDGE('',*,*,#6336,.T.);
#8989=ORIENTED_EDGE('',*,*,#6566,.T.);
#8990=ORIENTED_EDGE('',*,*,#6563,.T.);
#8991=ORIENTED_EDGE('',*,*,#6560,.T.);
#8992=ORIENTED_EDGE('',*,*,#6327,.T.);
#8993=ORIENTED_EDGE('',*,*,#6323,.F.);
#8994=ORIENTED_EDGE('',*,*,#6720,.T.);
#8995=ORIENTED_EDGE('',*,*,#6318,.F.);
#8996=ORIENTED_EDGE('',*,*,#6322,.T.);
#8997=ORIENTED_EDGE('',*,*,#6558,.T.);
#8998=ORIENTED_EDGE('',*,*,#6555,.T.);
#8999=ORIENTED_EDGE('',*,*,#6552,.T.);
#9000=ORIENTED_EDGE('',*,*,#6313,.T.);
#9001=ORIENTED_EDGE('',*,*,#6309,.F.);
#9002=ORIENTED_EDGE('',*,*,#6721,.T.);
#9003=ORIENTED_EDGE('',*,*,#6304,.F.);
#9004=ORIENTED_EDGE('',*,*,#6308,.T.);
#9005=ORIENTED_EDGE('',*,*,#6550,.T.);
#9006=ORIENTED_EDGE('',*,*,#6547,.T.);
#9007=ORIENTED_EDGE('',*,*,#6544,.T.);
#9008=ORIENTED_EDGE('',*,*,#6299,.T.);
#9009=ORIENTED_EDGE('',*,*,#6295,.F.);
#9010=ORIENTED_EDGE('',*,*,#6722,.T.);
#9011=ORIENTED_EDGE('',*,*,#6290,.F.);
#9012=ORIENTED_EDGE('',*,*,#6294,.T.);
#9013=ORIENTED_EDGE('',*,*,#6542,.T.);
#9014=ORIENTED_EDGE('',*,*,#6539,.T.);
#9015=ORIENTED_EDGE('',*,*,#6536,.T.);
#9016=ORIENTED_EDGE('',*,*,#6285,.T.);
#9017=ORIENTED_EDGE('',*,*,#6281,.F.);
#9018=ORIENTED_EDGE('',*,*,#6723,.T.);
#9019=ORIENTED_EDGE('',*,*,#6276,.F.);
#9020=ORIENTED_EDGE('',*,*,#6280,.T.);
#9021=ORIENTED_EDGE('',*,*,#6534,.T.);
#9022=ORIENTED_EDGE('',*,*,#6531,.T.);
#9023=ORIENTED_EDGE('',*,*,#6528,.T.);
#9024=ORIENTED_EDGE('',*,*,#6271,.T.);
#9025=ORIENTED_EDGE('',*,*,#6267,.F.);
#9026=ORIENTED_EDGE('',*,*,#6724,.T.);
#9027=ORIENTED_EDGE('',*,*,#6262,.F.);
#9028=ORIENTED_EDGE('',*,*,#6266,.T.);
#9029=ORIENTED_EDGE('',*,*,#6526,.T.);
#9030=ORIENTED_EDGE('',*,*,#6523,.T.);
#9031=ORIENTED_EDGE('',*,*,#6520,.T.);
#9032=ORIENTED_EDGE('',*,*,#6257,.T.);
#9033=ORIENTED_EDGE('',*,*,#6253,.F.);
#9034=ORIENTED_EDGE('',*,*,#6247,.T.);
#9035=ORIENTED_EDGE('',*,*,#6515,.F.);
#9036=ORIENTED_EDGE('',*,*,#6706,.F.);
#9037=ORIENTED_EDGE('',*,*,#6725,.F.);
#9038=ORIENTED_EDGE('',*,*,#6688,.T.);
#9039=ORIENTED_EDGE('',*,*,#6501,.F.);
#9040=ORIENTED_EDGE('',*,*,#6707,.F.);
#9041=ORIENTED_EDGE('',*,*,#6508,.F.);
#9042=ORIENTED_EDGE('',*,*,#6687,.T.);
#9043=ORIENTED_EDGE('',*,*,#6487,.F.);
#9044=ORIENTED_EDGE('',*,*,#6708,.F.);
#9045=ORIENTED_EDGE('',*,*,#6494,.F.);
#9046=ORIENTED_EDGE('',*,*,#6686,.T.);
#9047=ORIENTED_EDGE('',*,*,#6473,.F.);
#9048=ORIENTED_EDGE('',*,*,#6709,.F.);
#9049=ORIENTED_EDGE('',*,*,#6480,.F.);
#9050=ORIENTED_EDGE('',*,*,#6685,.T.);
#9051=ORIENTED_EDGE('',*,*,#6459,.F.);
#9052=ORIENTED_EDGE('',*,*,#6710,.F.);
#9053=ORIENTED_EDGE('',*,*,#6466,.F.);
#9054=ORIENTED_EDGE('',*,*,#6684,.T.);
#9055=ORIENTED_EDGE('',*,*,#6445,.F.);
#9056=ORIENTED_EDGE('',*,*,#6711,.F.);
#9057=ORIENTED_EDGE('',*,*,#6452,.F.);
#9058=ORIENTED_EDGE('',*,*,#6683,.T.);
#9059=ORIENTED_EDGE('',*,*,#6431,.F.);
#9060=ORIENTED_EDGE('',*,*,#6712,.F.);
#9061=ORIENTED_EDGE('',*,*,#6438,.F.);
#9062=ORIENTED_EDGE('',*,*,#6682,.T.);
#9063=ORIENTED_EDGE('',*,*,#6417,.F.);
#9064=ORIENTED_EDGE('',*,*,#6713,.F.);
#9065=ORIENTED_EDGE('',*,*,#6424,.F.);
#9066=ORIENTED_EDGE('',*,*,#6681,.T.);
#9067=ORIENTED_EDGE('',*,*,#6403,.F.);
#9068=ORIENTED_EDGE('',*,*,#6714,.F.);
#9069=ORIENTED_EDGE('',*,*,#6410,.F.);
#9070=ORIENTED_EDGE('',*,*,#6680,.T.);
#9071=ORIENTED_EDGE('',*,*,#6389,.F.);
#9072=ORIENTED_EDGE('',*,*,#6715,.F.);
#9073=ORIENTED_EDGE('',*,*,#6396,.F.);
#9074=ORIENTED_EDGE('',*,*,#6679,.T.);
#9075=ORIENTED_EDGE('',*,*,#6375,.F.);
#9076=ORIENTED_EDGE('',*,*,#6716,.F.);
#9077=ORIENTED_EDGE('',*,*,#6382,.F.);
#9078=ORIENTED_EDGE('',*,*,#6678,.T.);
#9079=ORIENTED_EDGE('',*,*,#6361,.F.);
#9080=ORIENTED_EDGE('',*,*,#6717,.F.);
#9081=ORIENTED_EDGE('',*,*,#6368,.F.);
#9082=ORIENTED_EDGE('',*,*,#6677,.T.);
#9083=ORIENTED_EDGE('',*,*,#6347,.F.);
#9084=ORIENTED_EDGE('',*,*,#6718,.F.);
#9085=ORIENTED_EDGE('',*,*,#6354,.F.);
#9086=ORIENTED_EDGE('',*,*,#6676,.T.);
#9087=ORIENTED_EDGE('',*,*,#6333,.F.);
#9088=ORIENTED_EDGE('',*,*,#6719,.F.);
#9089=ORIENTED_EDGE('',*,*,#6340,.F.);
#9090=ORIENTED_EDGE('',*,*,#6675,.T.);
#9091=ORIENTED_EDGE('',*,*,#6319,.F.);
#9092=ORIENTED_EDGE('',*,*,#6720,.F.);
#9093=ORIENTED_EDGE('',*,*,#6326,.F.);
#9094=ORIENTED_EDGE('',*,*,#6674,.T.);
#9095=ORIENTED_EDGE('',*,*,#6305,.F.);
#9096=ORIENTED_EDGE('',*,*,#6721,.F.);
#9097=ORIENTED_EDGE('',*,*,#6312,.F.);
#9098=ORIENTED_EDGE('',*,*,#6673,.T.);
#9099=ORIENTED_EDGE('',*,*,#6291,.F.);
#9100=ORIENTED_EDGE('',*,*,#6722,.F.);
#9101=ORIENTED_EDGE('',*,*,#6298,.F.);
#9102=ORIENTED_EDGE('',*,*,#6672,.T.);
#9103=ORIENTED_EDGE('',*,*,#6277,.F.);
#9104=ORIENTED_EDGE('',*,*,#6723,.F.);
#9105=ORIENTED_EDGE('',*,*,#6284,.F.);
#9106=ORIENTED_EDGE('',*,*,#6671,.T.);
#9107=ORIENTED_EDGE('',*,*,#6263,.F.);
#9108=ORIENTED_EDGE('',*,*,#6724,.F.);
#9109=ORIENTED_EDGE('',*,*,#6270,.F.);
#9110=ORIENTED_EDGE('',*,*,#6697,.T.);
#9111=ORIENTED_EDGE('',*,*,#6705,.T.);
#9112=ORIENTED_EDGE('',*,*,#6726,.T.);
#9113=ORIENTED_EDGE('',*,*,#6689,.T.);
#9114=ORIENTED_EDGE('',*,*,#6725,.T.);
#9115=ORIENTED_EDGE('',*,*,#6726,.F.);
#9116=ORIENTED_EDGE('',*,*,#6704,.F.);
#9117=ORIENTED_EDGE('',*,*,#6727,.F.);
#9118=ORIENTED_EDGE('',*,*,#6690,.F.);
#9119=ORIENTED_EDGE('',*,*,#6695,.T.);
#9120=ORIENTED_EDGE('',*,*,#6728,.T.);
#9121=ORIENTED_EDGE('',*,*,#6699,.T.);
#9122=ORIENTED_EDGE('',*,*,#6729,.T.);
#9123=ORIENTED_EDGE('',*,*,#6728,.F.);
#9124=ORIENTED_EDGE('',*,*,#6694,.T.);
#9125=ORIENTED_EDGE('',*,*,#6730,.T.);
#9126=ORIENTED_EDGE('',*,*,#6700,.F.);
#9127=ORIENTED_EDGE('',*,*,#6691,.F.);
#9128=ORIENTED_EDGE('',*,*,#6727,.T.);
#9129=ORIENTED_EDGE('',*,*,#6703,.F.);
#9130=ORIENTED_EDGE('',*,*,#6731,.F.);
#9131=ORIENTED_EDGE('',*,*,#6692,.T.);
#9132=ORIENTED_EDGE('',*,*,#6731,.T.);
#9133=ORIENTED_EDGE('',*,*,#6702,.F.);
#9134=ORIENTED_EDGE('',*,*,#6732,.F.);
#9135=ORIENTED_EDGE('',*,*,#6693,.T.);
#9136=ORIENTED_EDGE('',*,*,#6732,.T.);
#9137=ORIENTED_EDGE('',*,*,#6701,.F.);
#9138=ORIENTED_EDGE('',*,*,#6730,.F.);
#9139=ORIENTED_EDGE('',*,*,#6256,.F.);
#9140=ORIENTED_EDGE('',*,*,#6696,.T.);
#9141=ORIENTED_EDGE('',*,*,#6729,.F.);
#9142=ORIENTED_EDGE('',*,*,#6698,.F.);
#12019=CYLINDRICAL_SURFACE('',#13186,7.5);
#12020=CYLINDRICAL_SURFACE('',#13189,7.5);
#12021=CYLINDRICAL_SURFACE('',#13194,1.);
#12022=CYLINDRICAL_SURFACE('',#13198,1.);
#12023=CYLINDRICAL_SURFACE('',#13202,1.);
#12024=CYLINDRICAL_SURFACE('',#13206,1.);
#12025=CYLINDRICAL_SURFACE('',#13210,1.);
#12026=CYLINDRICAL_SURFACE('',#13214,1.);
#12027=CYLINDRICAL_SURFACE('',#13218,1.);
#12028=CYLINDRICAL_SURFACE('',#13222,1.);
#12029=CYLINDRICAL_SURFACE('',#13226,1.);
#12030=CYLINDRICAL_SURFACE('',#13230,1.);
#12031=CYLINDRICAL_SURFACE('',#13234,1.);
#12032=CYLINDRICAL_SURFACE('',#13238,1.);
#12033=CYLINDRICAL_SURFACE('',#13242,1.);
#12034=CYLINDRICAL_SURFACE('',#13246,1.);
#12035=CYLINDRICAL_SURFACE('',#13250,1.);
#12036=CYLINDRICAL_SURFACE('',#13254,1.);
#12037=CYLINDRICAL_SURFACE('',#13258,1.);
#12038=CYLINDRICAL_SURFACE('',#13262,1.);
#12039=CYLINDRICAL_SURFACE('',#13266,1.);
#12040=CYLINDRICAL_SURFACE('',#13270,1.);
#12041=CYLINDRICAL_SURFACE('',#13274,1.);
#12042=CYLINDRICAL_SURFACE('',#13278,1.);
#12043=CYLINDRICAL_SURFACE('',#13282,1.);
#12044=CYLINDRICAL_SURFACE('',#13286,1.);
#12045=CYLINDRICAL_SURFACE('',#13290,1.);
#12046=CYLINDRICAL_SURFACE('',#13294,1.);
#12047=CYLINDRICAL_SURFACE('',#13298,1.);
#12048=CYLINDRICAL_SURFACE('',#13302,1.);
#12049=CYLINDRICAL_SURFACE('',#13306,1.);
#12050=CYLINDRICAL_SURFACE('',#13310,1.);
#12051=CYLINDRICAL_SURFACE('',#13314,1.);
#12052=CYLINDRICAL_SURFACE('',#13318,1.);
#12053=CYLINDRICAL_SURFACE('',#13322,1.);
#12054=CYLINDRICAL_SURFACE('',#13326,1.);
#12055=CYLINDRICAL_SURFACE('',#13330,1.);
#12056=CYLINDRICAL_SURFACE('',#13334,1.);
#12057=CYLINDRICAL_SURFACE('',#13338,1.);
#12058=CYLINDRICAL_SURFACE('',#13342,1.);
#12059=CYLINDRICAL_SURFACE('',#13346,43.9999999999887);
#12060=CYLINDRICAL_SURFACE('',#13349,43.9999999999887);
#12061=CYLINDRICAL_SURFACE('',#13352,43.9999999999887);
#12062=CYLINDRICAL_SURFACE('',#13355,43.9999999999887);
#12063=CYLINDRICAL_SURFACE('',#13358,43.9999999999887);
#12064=CYLINDRICAL_SURFACE('',#13361,43.9999999999887);
#12065=CYLINDRICAL_SURFACE('',#13364,43.9999999999887);
#12066=CYLINDRICAL_SURFACE('',#13367,43.9999999999887);
#12067=CYLINDRICAL_SURFACE('',#13370,43.9999999999887);
#12068=CYLINDRICAL_SURFACE('',#13373,43.9999999999887);
#12069=CYLINDRICAL_SURFACE('',#13376,43.9999999999887);
#12070=CYLINDRICAL_SURFACE('',#13379,43.9999999999887);
#12071=CYLINDRICAL_SURFACE('',#13382,43.9999999999887);
#12072=CYLINDRICAL_SURFACE('',#13385,43.9999999999887);
#12073=CYLINDRICAL_SURFACE('',#13388,43.9999999999887);
#12074=CYLINDRICAL_SURFACE('',#13391,43.9999999999887);
#12075=CYLINDRICAL_SURFACE('',#13394,43.9999999999887);
#12076=CYLINDRICAL_SURFACE('',#13397,43.9999999999887);
#12077=CYLINDRICAL_SURFACE('',#13400,43.9999999999887);
#12078=CYLINDRICAL_SURFACE('',#13451,35.372);
#12079=CYLINDRICAL_SURFACE('',#13452,35.372);
#12080=CYLINDRICAL_SURFACE('',#13453,35.372);
#12081=CYLINDRICAL_SURFACE('',#13454,35.372);
#12082=CYLINDRICAL_SURFACE('',#13455,35.372);
#12083=CYLINDRICAL_SURFACE('',#13456,35.372);
#12084=CYLINDRICAL_SURFACE('',#13457,35.372);
#12085=CYLINDRICAL_SURFACE('',#13458,35.372);
#12086=CYLINDRICAL_SURFACE('',#13459,35.372);
#12087=CYLINDRICAL_SURFACE('',#13460,35.372);
#12088=CYLINDRICAL_SURFACE('',#13461,35.372);
#12089=CYLINDRICAL_SURFACE('',#13462,35.372);
#12090=CYLINDRICAL_SURFACE('',#13463,35.372);
#12091=CYLINDRICAL_SURFACE('',#13464,35.372);
#12092=CYLINDRICAL_SURFACE('',#13465,35.372);
#12093=CYLINDRICAL_SURFACE('',#13466,35.372);
#12094=CYLINDRICAL_SURFACE('',#13467,35.372);
#12095=CYLINDRICAL_SURFACE('',#13468,35.372);
#12096=CYLINDRICAL_SURFACE('',#13469,35.372);
#12097=CYLINDRICAL_SURFACE('',#13470,1.);
#12098=CYLINDRICAL_SURFACE('',#13472,1.);
#12099=CYLINDRICAL_SURFACE('',#13474,43.9999999999887);
#12100=CYLINDRICAL_SURFACE('',#13475,35.372);
#12299=ADVANCED_FACE('',(#1287),#12019,.T.);
#12300=ADVANCED_FACE('',(#1288),#12020,.T.);
#12301=ADVANCED_FACE('',(#1289),#1007,.F.);
#12302=ADVANCED_FACE('',(#1290),#1008,.T.);
#12303=ADVANCED_FACE('',(#1291),#12021,.F.);
#12304=ADVANCED_FACE('',(#1292),#1009,.T.);
#12305=ADVANCED_FACE('',(#1293),#12022,.F.);
#12306=ADVANCED_FACE('',(#1294),#1010,.T.);
#12307=ADVANCED_FACE('',(#1295),#12023,.F.);
#12308=ADVANCED_FACE('',(#1296),#1011,.T.);
#12309=ADVANCED_FACE('',(#1297),#12024,.F.);
#12310=ADVANCED_FACE('',(#1298),#1012,.T.);
#12311=ADVANCED_FACE('',(#1299),#12025,.F.);
#12312=ADVANCED_FACE('',(#1300),#1013,.T.);
#12313=ADVANCED_FACE('',(#1301),#12026,.F.);
#12314=ADVANCED_FACE('',(#1302),#1014,.T.);
#12315=ADVANCED_FACE('',(#1303),#12027,.F.);
#12316=ADVANCED_FACE('',(#1304),#1015,.T.);
#12317=ADVANCED_FACE('',(#1305),#12028,.F.);
#12318=ADVANCED_FACE('',(#1306),#1016,.T.);
#12319=ADVANCED_FACE('',(#1307),#12029,.F.);
#12320=ADVANCED_FACE('',(#1308),#1017,.T.);
#12321=ADVANCED_FACE('',(#1309),#12030,.F.);
#12322=ADVANCED_FACE('',(#1310),#1018,.T.);
#12323=ADVANCED_FACE('',(#1311),#12031,.F.);
#12324=ADVANCED_FACE('',(#1312),#1019,.T.);
#12325=ADVANCED_FACE('',(#1313),#12032,.F.);
#12326=ADVANCED_FACE('',(#1314),#1020,.T.);
#12327=ADVANCED_FACE('',(#1315),#12033,.F.);
#12328=ADVANCED_FACE('',(#1316),#1021,.T.);
#12329=ADVANCED_FACE('',(#1317),#12034,.F.);
#12330=ADVANCED_FACE('',(#1318),#1022,.T.);
#12331=ADVANCED_FACE('',(#1319),#12035,.F.);
#12332=ADVANCED_FACE('',(#1320),#1023,.T.);
#12333=ADVANCED_FACE('',(#1321),#12036,.F.);
#12334=ADVANCED_FACE('',(#1322),#1024,.T.);
#12335=ADVANCED_FACE('',(#1323),#12037,.F.);
#12336=ADVANCED_FACE('',(#1324),#1025,.T.);
#12337=ADVANCED_FACE('',(#1325),#12038,.F.);
#12338=ADVANCED_FACE('',(#1326),#1026,.T.);
#12339=ADVANCED_FACE('',(#1327),#12039,.F.);
#12340=ADVANCED_FACE('',(#1328),#1027,.T.);
#12341=ADVANCED_FACE('',(#1329),#12040,.F.);
#12342=ADVANCED_FACE('',(#1330),#1028,.T.);
#12343=ADVANCED_FACE('',(#1331),#12041,.F.);
#12344=ADVANCED_FACE('',(#1332),#1029,.T.);
#12345=ADVANCED_FACE('',(#1333),#12042,.F.);
#12346=ADVANCED_FACE('',(#1334),#1030,.T.);
#12347=ADVANCED_FACE('',(#1335),#12043,.F.);
#12348=ADVANCED_FACE('',(#1336),#1031,.T.);
#12349=ADVANCED_FACE('',(#1337),#12044,.F.);
#12350=ADVANCED_FACE('',(#1338),#1032,.T.);
#12351=ADVANCED_FACE('',(#1339),#12045,.F.);
#12352=ADVANCED_FACE('',(#1340),#1033,.T.);
#12353=ADVANCED_FACE('',(#1341),#12046,.F.);
#12354=ADVANCED_FACE('',(#1342),#1034,.T.);
#12355=ADVANCED_FACE('',(#1343),#12047,.F.);
#12356=ADVANCED_FACE('',(#1344),#1035,.T.);
#12357=ADVANCED_FACE('',(#1345),#12048,.F.);
#12358=ADVANCED_FACE('',(#1346),#1036,.T.);
#12359=ADVANCED_FACE('',(#1347),#12049,.F.);
#12360=ADVANCED_FACE('',(#1348),#1037,.T.);
#12361=ADVANCED_FACE('',(#1349),#12050,.F.);
#12362=ADVANCED_FACE('',(#1350),#1038,.T.);
#12363=ADVANCED_FACE('',(#1351),#12051,.F.);
#12364=ADVANCED_FACE('',(#1352),#1039,.T.);
#12365=ADVANCED_FACE('',(#1353),#12052,.F.);
#12366=ADVANCED_FACE('',(#1354),#1040,.T.);
#12367=ADVANCED_FACE('',(#1355),#12053,.F.);
#12368=ADVANCED_FACE('',(#1356),#1041,.T.);
#12369=ADVANCED_FACE('',(#1357),#12054,.F.);
#12370=ADVANCED_FACE('',(#1358),#1042,.T.);
#12371=ADVANCED_FACE('',(#1359),#12055,.F.);
#12372=ADVANCED_FACE('',(#1360),#1043,.T.);
#12373=ADVANCED_FACE('',(#1361),#12056,.F.);
#12374=ADVANCED_FACE('',(#1362),#1044,.T.);
#12375=ADVANCED_FACE('',(#1363),#12057,.F.);
#12376=ADVANCED_FACE('',(#1364),#1045,.T.);
#12377=ADVANCED_FACE('',(#1365),#12058,.F.);
#12378=ADVANCED_FACE('',(#1366),#1046,.T.);
#12379=ADVANCED_FACE('',(#1367),#947,.T.);
#12380=ADVANCED_FACE('',(#1368),#12059,.T.);
#12381=ADVANCED_FACE('',(#1369),#948,.T.);
#12382=ADVANCED_FACE('',(#1370),#949,.T.);
#12383=ADVANCED_FACE('',(#1371),#12060,.T.);
#12384=ADVANCED_FACE('',(#1372),#950,.T.);
#12385=ADVANCED_FACE('',(#1373),#951,.T.);
#12386=ADVANCED_FACE('',(#1374),#12061,.T.);
#12387=ADVANCED_FACE('',(#1375),#952,.T.);
#12388=ADVANCED_FACE('',(#1376),#953,.T.);
#12389=ADVANCED_FACE('',(#1377),#12062,.T.);
#12390=ADVANCED_FACE('',(#1378),#954,.T.);
#12391=ADVANCED_FACE('',(#1379),#955,.T.);
#12392=ADVANCED_FACE('',(#1380),#12063,.T.);
#12393=ADVANCED_FACE('',(#1381),#956,.T.);
#12394=ADVANCED_FACE('',(#1382),#957,.T.);
#12395=ADVANCED_FACE('',(#1383),#12064,.T.);
#12396=ADVANCED_FACE('',(#1384),#958,.T.);
#12397=ADVANCED_FACE('',(#1385),#959,.T.);
#12398=ADVANCED_FACE('',(#1386),#12065,.T.);
#12399=ADVANCED_FACE('',(#1387),#960,.T.);
#12400=ADVANCED_FACE('',(#1388),#961,.T.);
#12401=ADVANCED_FACE('',(#1389),#12066,.T.);
#12402=ADVANCED_FACE('',(#1390),#962,.T.);
#12403=ADVANCED_FACE('',(#1391),#963,.T.);
#12404=ADVANCED_FACE('',(#1392),#12067,.T.);
#12405=ADVANCED_FACE('',(#1393),#964,.T.);
#12406=ADVANCED_FACE('',(#1394),#965,.T.);
#12407=ADVANCED_FACE('',(#1395),#12068,.T.);
#12408=ADVANCED_FACE('',(#1396),#966,.T.);
#12409=ADVANCED_FACE('',(#1397),#967,.T.);
#12410=ADVANCED_FACE('',(#1398),#12069,.T.);
#12411=ADVANCED_FACE('',(#1399),#968,.T.);
#12412=ADVANCED_FACE('',(#1400),#969,.T.);
#12413=ADVANCED_FACE('',(#1401),#12070,.T.);
#12414=ADVANCED_FACE('',(#1402),#970,.T.);
#12415=ADVANCED_FACE('',(#1403),#971,.T.);
#12416=ADVANCED_FACE('',(#1404),#12071,.T.);
#12417=ADVANCED_FACE('',(#1405),#972,.T.);
#12418=ADVANCED_FACE('',(#1406),#973,.T.);
#12419=ADVANCED_FACE('',(#1407),#12072,.T.);
#12420=ADVANCED_FACE('',(#1408),#974,.T.);
#12421=ADVANCED_FACE('',(#1409),#975,.T.);
#12422=ADVANCED_FACE('',(#1410),#12073,.T.);
#12423=ADVANCED_FACE('',(#1411),#976,.T.);
#12424=ADVANCED_FACE('',(#1412),#977,.T.);
#12425=ADVANCED_FACE('',(#1413),#12074,.T.);
#12426=ADVANCED_FACE('',(#1414),#978,.T.);
#12427=ADVANCED_FACE('',(#1415),#979,.T.);
#12428=ADVANCED_FACE('',(#1416),#12075,.T.);
#12429=ADVANCED_FACE('',(#1417),#980,.T.);
#12430=ADVANCED_FACE('',(#1418),#981,.T.);
#12431=ADVANCED_FACE('',(#1419),#12076,.T.);
#12432=ADVANCED_FACE('',(#1420),#982,.T.);
#12433=ADVANCED_FACE('',(#1421),#983,.T.);
#12434=ADVANCED_FACE('',(#1422),#12077,.T.);
#12435=ADVANCED_FACE('',(#1423),#984,.T.);
#12436=ADVANCED_FACE('',(#1424,#279),#1047,.F.);
#12437=ADVANCED_FACE('',(#1425,#280),#1048,.T.);
#12438=ADVANCED_FACE('',(#1426),#12078,.T.);
#12439=ADVANCED_FACE('',(#1427),#12079,.T.);
#12440=ADVANCED_FACE('',(#1428),#12080,.T.);
#12441=ADVANCED_FACE('',(#1429),#12081,.T.);
#12442=ADVANCED_FACE('',(#1430),#12082,.T.);
#12443=ADVANCED_FACE('',(#1431),#12083,.T.);
#12444=ADVANCED_FACE('',(#1432),#12084,.T.);
#12445=ADVANCED_FACE('',(#1433),#12085,.T.);
#12446=ADVANCED_FACE('',(#1434),#12086,.T.);
#12447=ADVANCED_FACE('',(#1435),#12087,.T.);
#12448=ADVANCED_FACE('',(#1436),#12088,.T.);
#12449=ADVANCED_FACE('',(#1437),#12089,.T.);
#12450=ADVANCED_FACE('',(#1438),#12090,.T.);
#12451=ADVANCED_FACE('',(#1439),#12091,.T.);
#12452=ADVANCED_FACE('',(#1440),#12092,.T.);
#12453=ADVANCED_FACE('',(#1441),#12093,.T.);
#12454=ADVANCED_FACE('',(#1442),#12094,.T.);
#12455=ADVANCED_FACE('',(#1443),#12095,.T.);
#12456=ADVANCED_FACE('',(#1444),#12096,.T.);
#12457=ADVANCED_FACE('',(#1445),#12097,.F.);
#12458=ADVANCED_FACE('',(#1446),#1049,.T.);
#12459=ADVANCED_FACE('',(#1447),#12098,.F.);
#12460=ADVANCED_FACE('',(#1448),#1050,.T.);
#12461=ADVANCED_FACE('',(#1449),#985,.T.);
#12462=ADVANCED_FACE('',(#1450),#12099,.T.);
#12463=ADVANCED_FACE('',(#1451),#986,.T.);
#12464=ADVANCED_FACE('',(#1452),#12100,.T.);
#13051=CLOSED_SHELL('',(#12299,#12300,#12301,#12302,#12303,#12304,#12305,
#12306,#12307,#12308,#12309,#12310,#12311,#12312,#12313,#12314,#12315,#12316,
#12317,#12318,#12319,#12320,#12321,#12322,#12323,#12324,#12325,#12326,#12327,
#12328,#12329,#12330,#12331,#12332,#12333,#12334,#12335,#12336,#12337,#12338,
#12339,#12340,#12341,#12342,#12343,#12344,#12345,#12346,#12347,#12348,#12349,
#12350,#12351,#12352,#12353,#12354,#12355,#12356,#12357,#12358,#12359,#12360,
#12361,#12362,#12363,#12364,#12365,#12366,#12367,#12368,#12369,#12370,#12371,
#12372,#12373,#12374,#12375,#12376,#12377,#12378,#12379,#12380,#12381,#12382,
#12383,#12384,#12385,#12386,#12387,#12388,#12389,#12390,#12391,#12392,#12393,
#12394,#12395,#12396,#12397,#12398,#12399,#12400,#12401,#12402,#12403,#12404,
#12405,#12406,#12407,#12408,#12409,#12410,#12411,#12412,#12413,#12414,#12415,
#12416,#12417,#12418,#12419,#12420,#12421,#12422,#12423,#12424,#12425,#12426,
#12427,#12428,#12429,#12430,#12431,#12432,#12433,#12434,#12435,#12436,#12437,
#12438,#12439,#12440,#12441,#12442,#12443,#12444,#12445,#12446,#12447,#12448,
#12449,#12450,#12451,#12452,#12453,#12454,#12455,#12456,#12457,#12458,#12459,
#12460,#12461,#12462,#12463,#12464));
#13185=AXIS2_PLACEMENT_3D('',#18820,#14915,#14916);
#13186=AXIS2_PLACEMENT_3D('',#18821,#14917,#14918);
#13187=AXIS2_PLACEMENT_3D('',#18823,#14919,#14920);
#13188=AXIS2_PLACEMENT_3D('',#18826,#14922,#14923);
#13189=AXIS2_PLACEMENT_3D('',#18827,#14924,#14925);
#13190=AXIS2_PLACEMENT_3D('',#18829,#14926,#14927);
#13191=AXIS2_PLACEMENT_3D('',#18832,#14929,#14930);
#13192=AXIS2_PLACEMENT_3D('',#18833,#14931,#14932);
#13193=AXIS2_PLACEMENT_3D('',#18834,#14933,#14934);
#13194=AXIS2_PLACEMENT_3D('',#18835,#14935,#14936);
#13195=AXIS2_PLACEMENT_3D('',#18838,#14937,#14938);
#13196=AXIS2_PLACEMENT_3D('',#18842,#14940,#14941);
#13197=AXIS2_PLACEMENT_3D('',#18844,#14943,#14944);
#13198=AXIS2_PLACEMENT_3D('',#18850,#14948,#14949);
#13199=AXIS2_PLACEMENT_3D('',#18853,#14950,#14951);
#13200=AXIS2_PLACEMENT_3D('',#18857,#14953,#14954);
#13201=AXIS2_PLACEMENT_3D('',#18859,#14956,#14957);
#13202=AXIS2_PLACEMENT_3D('',#18865,#14961,#14962);
#13203=AXIS2_PLACEMENT_3D('',#18868,#14963,#14964);
#13204=AXIS2_PLACEMENT_3D('',#18872,#14966,#14967);
#13205=AXIS2_PLACEMENT_3D('',#18874,#14969,#14970);
#13206=AXIS2_PLACEMENT_3D('',#18880,#14974,#14975);
#13207=AXIS2_PLACEMENT_3D('',#18883,#14976,#14977);
#13208=AXIS2_PLACEMENT_3D('',#18887,#14979,#14980);
#13209=AXIS2_PLACEMENT_3D('',#18889,#14982,#14983);
#13210=AXIS2_PLACEMENT_3D('',#18895,#14987,#14988);
#13211=AXIS2_PLACEMENT_3D('',#18898,#14989,#14990);
#13212=AXIS2_PLACEMENT_3D('',#18902,#14992,#14993);
#13213=AXIS2_PLACEMENT_3D('',#18904,#14995,#14996);
#13214=AXIS2_PLACEMENT_3D('',#18910,#15000,#15001);
#13215=AXIS2_PLACEMENT_3D('',#18913,#15002,#15003);
#13216=AXIS2_PLACEMENT_3D('',#18917,#15005,#15006);
#13217=AXIS2_PLACEMENT_3D('',#18919,#15008,#15009);
#13218=AXIS2_PLACEMENT_3D('',#18925,#15013,#15014);
#13219=AXIS2_PLACEMENT_3D('',#18928,#15015,#15016);
#13220=AXIS2_PLACEMENT_3D('',#18932,#15018,#15019);
#13221=AXIS2_PLACEMENT_3D('',#18934,#15021,#15022);
#13222=AXIS2_PLACEMENT_3D('',#18940,#15026,#15027);
#13223=AXIS2_PLACEMENT_3D('',#18943,#15028,#15029);
#13224=AXIS2_PLACEMENT_3D('',#18947,#15031,#15032);
#13225=AXIS2_PLACEMENT_3D('',#18949,#15034,#15035);
#13226=AXIS2_PLACEMENT_3D('',#18955,#15039,#15040);
#13227=AXIS2_PLACEMENT_3D('',#18958,#15041,#15042);
#13228=AXIS2_PLACEMENT_3D('',#18962,#15044,#15045);
#13229=AXIS2_PLACEMENT_3D('',#18964,#15047,#15048);
#13230=AXIS2_PLACEMENT_3D('',#18970,#15052,#15053);
#13231=AXIS2_PLACEMENT_3D('',#18973,#15054,#15055);
#13232=AXIS2_PLACEMENT_3D('',#18977,#15057,#15058);
#13233=AXIS2_PLACEMENT_3D('',#18979,#15060,#15061);
#13234=AXIS2_PLACEMENT_3D('',#18985,#15065,#15066);
#13235=AXIS2_PLACEMENT_3D('',#18988,#15067,#15068);
#13236=AXIS2_PLACEMENT_3D('',#18992,#15070,#15071);
#13237=AXIS2_PLACEMENT_3D('',#18994,#15073,#15074);
#13238=AXIS2_PLACEMENT_3D('',#19000,#15078,#15079);
#13239=AXIS2_PLACEMENT_3D('',#19003,#15080,#15081);
#13240=AXIS2_PLACEMENT_3D('',#19007,#15083,#15084);
#13241=AXIS2_PLACEMENT_3D('',#19009,#15086,#15087);
#13242=AXIS2_PLACEMENT_3D('',#19015,#15091,#15092);
#13243=AXIS2_PLACEMENT_3D('',#19018,#15093,#15094);
#13244=AXIS2_PLACEMENT_3D('',#19022,#15096,#15097);
#13245=AXIS2_PLACEMENT_3D('',#19024,#15099,#15100);
#13246=AXIS2_PLACEMENT_3D('',#19030,#15104,#15105);
#13247=AXIS2_PLACEMENT_3D('',#19033,#15106,#15107);
#13248=AXIS2_PLACEMENT_3D('',#19037,#15109,#15110);
#13249=AXIS2_PLACEMENT_3D('',#19039,#15112,#15113);
#13250=AXIS2_PLACEMENT_3D('',#19045,#15117,#15118);
#13251=AXIS2_PLACEMENT_3D('',#19048,#15119,#15120);
#13252=AXIS2_PLACEMENT_3D('',#19052,#15122,#15123);
#13253=AXIS2_PLACEMENT_3D('',#19054,#15125,#15126);
#13254=AXIS2_PLACEMENT_3D('',#19060,#15130,#15131);
#13255=AXIS2_PLACEMENT_3D('',#19063,#15132,#15133);
#13256=AXIS2_PLACEMENT_3D('',#19067,#15135,#15136);
#13257=AXIS2_PLACEMENT_3D('',#19069,#15138,#15139);
#13258=AXIS2_PLACEMENT_3D('',#19075,#15143,#15144);
#13259=AXIS2_PLACEMENT_3D('',#19078,#15145,#15146);
#13260=AXIS2_PLACEMENT_3D('',#19082,#15148,#15149);
#13261=AXIS2_PLACEMENT_3D('',#19084,#15151,#15152);
#13262=AXIS2_PLACEMENT_3D('',#19090,#15156,#15157);
#13263=AXIS2_PLACEMENT_3D('',#19093,#15158,#15159);
#13264=AXIS2_PLACEMENT_3D('',#19097,#15161,#15162);
#13265=AXIS2_PLACEMENT_3D('',#19099,#15164,#15165);
#13266=AXIS2_PLACEMENT_3D('',#19105,#15169,#15170);
#13267=AXIS2_PLACEMENT_3D('',#19108,#15171,#15172);
#13268=AXIS2_PLACEMENT_3D('',#19112,#15174,#15175);
#13269=AXIS2_PLACEMENT_3D('',#19114,#15177,#15178);
#13270=AXIS2_PLACEMENT_3D('',#19120,#15182,#15183);
#13271=AXIS2_PLACEMENT_3D('',#19123,#15184,#15185);
#13272=AXIS2_PLACEMENT_3D('',#19127,#15187,#15188);
#13273=AXIS2_PLACEMENT_3D('',#19129,#15190,#15191);
#13274=AXIS2_PLACEMENT_3D('',#19135,#15195,#15196);
#13275=AXIS2_PLACEMENT_3D('',#19138,#15197,#15198);
#13276=AXIS2_PLACEMENT_3D('',#19142,#15200,#15201);
#13277=AXIS2_PLACEMENT_3D('',#19144,#15203,#15204);
#13278=AXIS2_PLACEMENT_3D('',#19150,#15208,#15209);
#13279=AXIS2_PLACEMENT_3D('',#19153,#15210,#15211);
#13280=AXIS2_PLACEMENT_3D('',#19157,#15213,#15214);
#13281=AXIS2_PLACEMENT_3D('',#19159,#15216,#15217);
#13282=AXIS2_PLACEMENT_3D('',#19165,#15221,#15222);
#13283=AXIS2_PLACEMENT_3D('',#19168,#15223,#15224);
#13284=AXIS2_PLACEMENT_3D('',#19172,#15226,#15227);
#13285=AXIS2_PLACEMENT_3D('',#19174,#15229,#15230);
#13286=AXIS2_PLACEMENT_3D('',#19180,#15234,#15235);
#13287=AXIS2_PLACEMENT_3D('',#19183,#15236,#15237);
#13288=AXIS2_PLACEMENT_3D('',#19187,#15239,#15240);
#13289=AXIS2_PLACEMENT_3D('',#19189,#15242,#15243);
#13290=AXIS2_PLACEMENT_3D('',#19195,#15247,#15248);
#13291=AXIS2_PLACEMENT_3D('',#19198,#15249,#15250);
#13292=AXIS2_PLACEMENT_3D('',#19202,#15252,#15253);
#13293=AXIS2_PLACEMENT_3D('',#19204,#15255,#15256);
#13294=AXIS2_PLACEMENT_3D('',#19210,#15260,#15261);
#13295=AXIS2_PLACEMENT_3D('',#19213,#15262,#15263);
#13296=AXIS2_PLACEMENT_3D('',#19217,#15265,#15266);
#13297=AXIS2_PLACEMENT_3D('',#19219,#15268,#15269);
#13298=AXIS2_PLACEMENT_3D('',#19225,#15273,#15274);
#13299=AXIS2_PLACEMENT_3D('',#19228,#15275,#15276);
#13300=AXIS2_PLACEMENT_3D('',#19232,#15278,#15279);
#13301=AXIS2_PLACEMENT_3D('',#19234,#15281,#15282);
#13302=AXIS2_PLACEMENT_3D('',#19240,#15286,#15287);
#13303=AXIS2_PLACEMENT_3D('',#19243,#15288,#15289);
#13304=AXIS2_PLACEMENT_3D('',#19247,#15291,#15292);
#13305=AXIS2_PLACEMENT_3D('',#19249,#15294,#15295);
#13306=AXIS2_PLACEMENT_3D('',#19255,#15299,#15300);
#13307=AXIS2_PLACEMENT_3D('',#19258,#15301,#15302);
#13308=AXIS2_PLACEMENT_3D('',#19262,#15304,#15305);
#13309=AXIS2_PLACEMENT_3D('',#19264,#15307,#15308);
#13310=AXIS2_PLACEMENT_3D('',#19270,#15312,#15313);
#13311=AXIS2_PLACEMENT_3D('',#19273,#15314,#15315);
#13312=AXIS2_PLACEMENT_3D('',#19277,#15317,#15318);
#13313=AXIS2_PLACEMENT_3D('',#19279,#15320,#15321);
#13314=AXIS2_PLACEMENT_3D('',#19285,#15325,#15326);
#13315=AXIS2_PLACEMENT_3D('',#19288,#15327,#15328);
#13316=AXIS2_PLACEMENT_3D('',#19292,#15330,#15331);
#13317=AXIS2_PLACEMENT_3D('',#19294,#15333,#15334);
#13318=AXIS2_PLACEMENT_3D('',#19300,#15338,#15339);
#13319=AXIS2_PLACEMENT_3D('',#19303,#15340,#15341);
#13320=AXIS2_PLACEMENT_3D('',#19307,#15343,#15344);
#13321=AXIS2_PLACEMENT_3D('',#19309,#15346,#15347);
#13322=AXIS2_PLACEMENT_3D('',#19315,#15351,#15352);
#13323=AXIS2_PLACEMENT_3D('',#19318,#15353,#15354);
#13324=AXIS2_PLACEMENT_3D('',#19322,#15356,#15357);
#13325=AXIS2_PLACEMENT_3D('',#19324,#15359,#15360);
#13326=AXIS2_PLACEMENT_3D('',#19330,#15364,#15365);
#13327=AXIS2_PLACEMENT_3D('',#19333,#15366,#15367);
#13328=AXIS2_PLACEMENT_3D('',#19337,#15369,#15370);
#13329=AXIS2_PLACEMENT_3D('',#19339,#15372,#15373);
#13330=AXIS2_PLACEMENT_3D('',#19345,#15377,#15378);
#13331=AXIS2_PLACEMENT_3D('',#19348,#15379,#15380);
#13332=AXIS2_PLACEMENT_3D('',#19352,#15382,#15383);
#13333=AXIS2_PLACEMENT_3D('',#19354,#15385,#15386);
#13334=AXIS2_PLACEMENT_3D('',#19360,#15390,#15391);
#13335=AXIS2_PLACEMENT_3D('',#19363,#15392,#15393);
#13336=AXIS2_PLACEMENT_3D('',#19367,#15395,#15396);
#13337=AXIS2_PLACEMENT_3D('',#19369,#15398,#15399);
#13338=AXIS2_PLACEMENT_3D('',#19375,#15403,#15404);
#13339=AXIS2_PLACEMENT_3D('',#19378,#15405,#15406);
#13340=AXIS2_PLACEMENT_3D('',#19382,#15408,#15409);
#13341=AXIS2_PLACEMENT_3D('',#19384,#15411,#15412);
#13342=AXIS2_PLACEMENT_3D('',#19390,#15416,#15417);
#13343=AXIS2_PLACEMENT_3D('',#19393,#15418,#15419);
#13344=AXIS2_PLACEMENT_3D('',#19397,#15421,#15422);
#13345=AXIS2_PLACEMENT_3D('',#19399,#15424,#15425);
#13346=AXIS2_PLACEMENT_3D('',#19707,#15430,#15431);
#13347=AXIS2_PLACEMENT_3D('',#19709,#15432,#15433);
#13348=AXIS2_PLACEMENT_3D('',#19711,#15434,#15435);
#13349=AXIS2_PLACEMENT_3D('',#20313,#15438,#15439);
#13350=AXIS2_PLACEMENT_3D('',#20315,#15440,#15441);
#13351=AXIS2_PLACEMENT_3D('',#20317,#15442,#15443);
#13352=AXIS2_PLACEMENT_3D('',#20919,#15446,#15447);
#13353=AXIS2_PLACEMENT_3D('',#20921,#15448,#15449);
#13354=AXIS2_PLACEMENT_3D('',#20923,#15450,#15451);
#13355=AXIS2_PLACEMENT_3D('',#21525,#15454,#15455);
#13356=AXIS2_PLACEMENT_3D('',#21527,#15456,#15457);
#13357=AXIS2_PLACEMENT_3D('',#21529,#15458,#15459);
#13358=AXIS2_PLACEMENT_3D('',#22131,#15462,#15463);
#13359=AXIS2_PLACEMENT_3D('',#22133,#15464,#15465);
#13360=AXIS2_PLACEMENT_3D('',#22135,#15466,#15467);
#13361=AXIS2_PLACEMENT_3D('',#22737,#15470,#15471);
#13362=AXIS2_PLACEMENT_3D('',#22739,#15472,#15473);
#13363=AXIS2_PLACEMENT_3D('',#22741,#15474,#15475);
#13364=AXIS2_PLACEMENT_3D('',#23343,#15478,#15479);
#13365=AXIS2_PLACEMENT_3D('',#23345,#15480,#15481);
#13366=AXIS2_PLACEMENT_3D('',#23347,#15482,#15483);
#13367=AXIS2_PLACEMENT_3D('',#23949,#15486,#15487);
#13368=AXIS2_PLACEMENT_3D('',#23951,#15488,#15489);
#13369=AXIS2_PLACEMENT_3D('',#23953,#15490,#15491);
#13370=AXIS2_PLACEMENT_3D('',#24555,#15494,#15495);
#13371=AXIS2_PLACEMENT_3D('',#24557,#15496,#15497);
#13372=AXIS2_PLACEMENT_3D('',#24559,#15498,#15499);
#13373=AXIS2_PLACEMENT_3D('',#25161,#15502,#15503);
#13374=AXIS2_PLACEMENT_3D('',#25163,#15504,#15505);
#13375=AXIS2_PLACEMENT_3D('',#25165,#15506,#15507);
#13376=AXIS2_PLACEMENT_3D('',#25767,#15510,#15511);
#13377=AXIS2_PLACEMENT_3D('',#25769,#15512,#15513);
#13378=AXIS2_PLACEMENT_3D('',#25771,#15514,#15515);
#13379=AXIS2_PLACEMENT_3D('',#26373,#15518,#15519);
#13380=AXIS2_PLACEMENT_3D('',#26375,#15520,#15521);
#13381=AXIS2_PLACEMENT_3D('',#26377,#15522,#15523);
#13382=AXIS2_PLACEMENT_3D('',#26979,#15526,#15527);
#13383=AXIS2_PLACEMENT_3D('',#26981,#15528,#15529);
#13384=AXIS2_PLACEMENT_3D('',#26983,#15530,#15531);
#13385=AXIS2_PLACEMENT_3D('',#27585,#15534,#15535);
#13386=AXIS2_PLACEMENT_3D('',#27587,#15536,#15537);
#13387=AXIS2_PLACEMENT_3D('',#27589,#15538,#15539);
#13388=AXIS2_PLACEMENT_3D('',#28191,#15542,#15543);
#13389=AXIS2_PLACEMENT_3D('',#28193,#15544,#15545);
#13390=AXIS2_PLACEMENT_3D('',#28195,#15546,#15547);
#13391=AXIS2_PLACEMENT_3D('',#28797,#15550,#15551);
#13392=AXIS2_PLACEMENT_3D('',#28799,#15552,#15553);
#13393=AXIS2_PLACEMENT_3D('',#28801,#15554,#15555);
#13394=AXIS2_PLACEMENT_3D('',#29403,#15558,#15559);
#13395=AXIS2_PLACEMENT_3D('',#29405,#15560,#15561);
#13396=AXIS2_PLACEMENT_3D('',#29407,#15562,#15563);
#13397=AXIS2_PLACEMENT_3D('',#30009,#15566,#15567);
#13398=AXIS2_PLACEMENT_3D('',#30011,#15568,#15569);
#13399=AXIS2_PLACEMENT_3D('',#30013,#15570,#15571);
#13400=AXIS2_PLACEMENT_3D('',#30615,#15574,#15575);
#13401=AXIS2_PLACEMENT_3D('',#30617,#15576,#15577);
#13402=AXIS2_PLACEMENT_3D('',#30619,#15578,#15579);
#13403=AXIS2_PLACEMENT_3D('',#30919,#15581,#15582);
#13404=AXIS2_PLACEMENT_3D('',#30920,#15583,#15584);
#13405=AXIS2_PLACEMENT_3D('',#30921,#15585,#15586);
#13406=AXIS2_PLACEMENT_3D('',#30922,#15587,#15588);
#13407=AXIS2_PLACEMENT_3D('',#30923,#15589,#15590);
#13408=AXIS2_PLACEMENT_3D('',#30924,#15591,#15592);
#13409=AXIS2_PLACEMENT_3D('',#30925,#15593,#15594);
#13410=AXIS2_PLACEMENT_3D('',#30926,#15595,#15596);
#13411=AXIS2_PLACEMENT_3D('',#30927,#15597,#15598);
#13412=AXIS2_PLACEMENT_3D('',#30928,#15599,#15600);
#13413=AXIS2_PLACEMENT_3D('',#30929,#15601,#15602);
#13414=AXIS2_PLACEMENT_3D('',#30930,#15603,#15604);
#13415=AXIS2_PLACEMENT_3D('',#30931,#15605,#15606);
#13416=AXIS2_PLACEMENT_3D('',#30932,#15607,#15608);
#13417=AXIS2_PLACEMENT_3D('',#30933,#15609,#15610);
#13418=AXIS2_PLACEMENT_3D('',#30934,#15611,#15612);
#13419=AXIS2_PLACEMENT_3D('',#30935,#15613,#15614);
#13420=AXIS2_PLACEMENT_3D('',#30936,#15615,#15616);
#13421=AXIS2_PLACEMENT_3D('',#30938,#15617,#15618);
#13422=AXIS2_PLACEMENT_3D('',#30940,#15619,#15620);
#13423=AXIS2_PLACEMENT_3D('',#31019,#15622,#15623);
#13424=AXIS2_PLACEMENT_3D('',#31098,#15625,#15626);
#13425=AXIS2_PLACEMENT_3D('',#31099,#15627,#15628);
#13426=AXIS2_PLACEMENT_3D('',#31100,#15629,#15630);
#13427=AXIS2_PLACEMENT_3D('',#31101,#15631,#15632);
#13428=AXIS2_PLACEMENT_3D('',#31103,#15633,#15634);
#13429=AXIS2_PLACEMENT_3D('',#31105,#15635,#15636);
#13430=AXIS2_PLACEMENT_3D('',#31184,#15638,#15639);
#13431=AXIS2_PLACEMENT_3D('',#31264,#15641,#15642);
#13432=AXIS2_PLACEMENT_3D('',#31265,#15643,#15644);
#13433=AXIS2_PLACEMENT_3D('',#31266,#15645,#15646);
#13434=AXIS2_PLACEMENT_3D('',#31267,#15647,#15648);
#13435=AXIS2_PLACEMENT_3D('',#31268,#15649,#15650);
#13436=AXIS2_PLACEMENT_3D('',#31269,#15651,#15652);
#13437=AXIS2_PLACEMENT_3D('',#31270,#15653,#15654);
#13438=AXIS2_PLACEMENT_3D('',#31271,#15655,#15656);
#13439=AXIS2_PLACEMENT_3D('',#31272,#15657,#15658);
#13440=AXIS2_PLACEMENT_3D('',#31273,#15659,#15660);
#13441=AXIS2_PLACEMENT_3D('',#31274,#15661,#15662);
#13442=AXIS2_PLACEMENT_3D('',#31275,#15663,#15664);
#13443=AXIS2_PLACEMENT_3D('',#31276,#15665,#15666);
#13444=AXIS2_PLACEMENT_3D('',#31277,#15667,#15668);
#13445=AXIS2_PLACEMENT_3D('',#31278,#15669,#15670);
#13446=AXIS2_PLACEMENT_3D('',#31279,#15671,#15672);
#13447=AXIS2_PLACEMENT_3D('',#31280,#15673,#15674);
#13448=AXIS2_PLACEMENT_3D('',#31281,#15675,#15676);
#13449=AXIS2_PLACEMENT_3D('',#31282,#15677,#15678);
#13450=AXIS2_PLACEMENT_3D('',#31283,#15679,#15680);
#13451=AXIS2_PLACEMENT_3D('',#31284,#15681,#15682);
#13452=AXIS2_PLACEMENT_3D('',#31286,#15684,#15685);
#13453=AXIS2_PLACEMENT_3D('',#31287,#15686,#15687);
#13454=AXIS2_PLACEMENT_3D('',#31288,#15688,#15689);
#13455=AXIS2_PLACEMENT_3D('',#31289,#15690,#15691);
#13456=AXIS2_PLACEMENT_3D('',#31290,#15692,#15693);
#13457=AXIS2_PLACEMENT_3D('',#31291,#15694,#15695);
#13458=AXIS2_PLACEMENT_3D('',#31292,#15696,#15697);
#13459=AXIS2_PLACEMENT_3D('',#31293,#15698,#15699);
#13460=AXIS2_PLACEMENT_3D('',#31294,#15700,#15701);
#13461=AXIS2_PLACEMENT_3D('',#31295,#15702,#15703);
#13462=AXIS2_PLACEMENT_3D('',#31296,#15704,#15705);
#13463=AXIS2_PLACEMENT_3D('',#31297,#15706,#15707);
#13464=AXIS2_PLACEMENT_3D('',#31298,#15708,#15709);
#13465=AXIS2_PLACEMENT_3D('',#31299,#15710,#15711);
#13466=AXIS2_PLACEMENT_3D('',#31300,#15712,#15713);
#13467=AXIS2_PLACEMENT_3D('',#31301,#15714,#15715);
#13468=AXIS2_PLACEMENT_3D('',#31302,#15716,#15717);
#13469=AXIS2_PLACEMENT_3D('',#31303,#15718,#15719);
#13470=AXIS2_PLACEMENT_3D('',#31304,#15720,#15721);
#13471=AXIS2_PLACEMENT_3D('',#31306,#15723,#15724);
#13472=AXIS2_PLACEMENT_3D('',#31308,#15726,#15727);
#13473=AXIS2_PLACEMENT_3D('',#31311,#15730,#15731);
#13474=AXIS2_PLACEMENT_3D('',#31464,#15734,#15735);
#13475=AXIS2_PLACEMENT_3D('',#31616,#15737,#15738);
#14915=DIRECTION('axis',(0.,0.,1.));
#14916=DIRECTION('refdir',(1.,0.,0.));
#14917=DIRECTION('center_axis',(0.,-2.4980018054066E-16,-1.));
#14918=DIRECTION('ref_axis',(1.,0.,0.));
#14919=DIRECTION('center_axis',(0.,-2.4980018054066E-16,-1.));
#14920=DIRECTION('ref_axis',(1.,0.,0.));
#14921=DIRECTION('',(0.,2.4980018054066E-16,1.));
#14922=DIRECTION('center_axis',(0.,-2.4980018054066E-16,-1.));
#14923=DIRECTION('ref_axis',(1.,0.,0.));
#14924=DIRECTION('center_axis',(0.,-2.4980018054066E-16,-1.));
#14925=DIRECTION('ref_axis',(1.,0.,0.));
#14926=DIRECTION('center_axis',(0.,-2.4980018054066E-16,-1.));
#14927=DIRECTION('ref_axis',(1.,0.,0.));
#14928=DIRECTION('',(0.,2.4980018054066E-16,1.));
#14929=DIRECTION('center_axis',(0.,2.4980018054066E-16,1.));
#14930=DIRECTION('ref_axis',(1.,0.,0.));
#14931=DIRECTION('center_axis',(0.,-2.4980018054066E-16,-1.));
#14932=DIRECTION('ref_axis',(1.,0.,0.));
#14933=DIRECTION('center_axis',(0.,-2.4980018054066E-16,-1.));
#14934=DIRECTION('ref_axis',(1.,0.,0.));
#14935=DIRECTION('center_axis',(0.,0.,-1.));
#14936=DIRECTION('ref_axis',(-0.837321103817045,-0.546711412998307,0.));
#14937=DIRECTION('center_axis',(0.,0.,1.));
#14938=DIRECTION('ref_axis',(-0.837321103817045,-0.546711412998307,0.));
#14939=DIRECTION('',(0.,0.,-1.));
#14940=DIRECTION('center_axis',(0.,0.,-1.));
#14941=DIRECTION('ref_axis',(-0.837321103817045,-0.546711412998307,0.));
#14942=DIRECTION('',(0.,0.,1.));
#14943=DIRECTION('center_axis',(0.21892739748686,0.975741151448288,0.));
#14944=DIRECTION('ref_axis',(-0.975741151448288,0.21892739748686,0.));
#14945=DIRECTION('',(-0.975741151448288,0.218927397486859,0.));
#14946=DIRECTION('',(0.,0.,1.));
#14947=DIRECTION('',(0.975741151448288,-0.218927397486859,0.));
#14948=DIRECTION('center_axis',(0.,0.,1.));
#14949=DIRECTION('ref_axis',(-0.356058096916393,0.934463820391285,0.));
#14950=DIRECTION('center_axis',(0.,0.,-1.));
#14951=DIRECTION('ref_axis',(-0.356058096916393,0.934463820391285,0.));
#14952=DIRECTION('',(0.,0.,1.));
#14953=DIRECTION('center_axis',(0.,0.,1.));
#14954=DIRECTION('ref_axis',(-0.356058096916393,0.934463820391285,0.));
#14955=DIRECTION('',(0.,0.,-1.));
#14956=DIRECTION('center_axis',(-0.396410273775032,-0.918073469198192,0.));
#14957=DIRECTION('ref_axis',(0.918073469198192,-0.396410273775032,0.));
#14958=DIRECTION('',(0.918073469198192,-0.396410273775032,0.));
#14959=DIRECTION('',(0.,0.,1.));
#14960=DIRECTION('',(0.918073469198192,-0.396410273775032,0.));
#14961=DIRECTION('center_axis',(0.,0.,-1.));
#14962=DIRECTION('ref_axis',(-0.96528280965187,-0.261207001036709,0.));
#14963=DIRECTION('center_axis',(0.,0.,1.));
#14964=DIRECTION('ref_axis',(-0.96528280965187,-0.261207001036709,0.));
#14965=DIRECTION('',(0.,0.,-1.));
#14966=DIRECTION('center_axis',(0.,0.,-1.));
#14967=DIRECTION('ref_axis',(-0.96528280965187,-0.261207001036709,0.));
#14968=DIRECTION('',(0.,0.,1.));
#14969=DIRECTION('center_axis',(0.509732925883917,0.860332693944512,0.));
#14970=DIRECTION('ref_axis',(-0.860332693944512,0.509732925883917,0.));
#14971=DIRECTION('',(-0.860332693944512,0.509732925883917,0.));
#14972=DIRECTION('',(0.,0.,1.));
#14973=DIRECTION('',(0.860332693944512,-0.509732925883917,0.));
#14974=DIRECTION('center_axis',(0.,0.,1.));
#14975=DIRECTION('ref_axis',(-0.0498661721225461,0.998755908557163,0.));
#14976=DIRECTION('center_axis',(0.,0.,-1.));
#14977=DIRECTION('ref_axis',(-0.0498661721225461,0.998755908557163,0.));
#14978=DIRECTION('',(0.,0.,1.));
#14979=DIRECTION('center_axis',(0.,0.,1.));
#14980=DIRECTION('ref_axis',(-0.0498661721225461,0.998755908557163,0.));
#14981=DIRECTION('',(0.,0.,-1.));
#14982=DIRECTION('center_axis',(-0.660708878067096,-0.750642243977328,0.));
#14983=DIRECTION('ref_axis',(0.750642243977328,-0.660708878067096,0.));
#14984=DIRECTION('',(0.750642243977328,-0.660708878067096,0.));
#14985=DIRECTION('',(0.,0.,1.));
#14986=DIRECTION('',(0.750642243977328,-0.660708878067096,0.));
#14987=DIRECTION('center_axis',(0.,0.,-1.));
#14988=DIRECTION('ref_axis',(-0.998755908557163,0.0498661721225458,0.));
#14989=DIRECTION('center_axis',(0.,0.,1.));
#14990=DIRECTION('ref_axis',(-0.998755908557163,0.0498661721225458,0.));
#14991=DIRECTION('',(0.,0.,-1.));
#14992=DIRECTION('center_axis',(0.,0.,-1.));
#14993=DIRECTION('ref_axis',(-0.998755908557163,0.0498661721225458,0.));
#14994=DIRECTION('',(0.,0.,1.));
#14995=DIRECTION('center_axis',(0.750642243977329,0.660708878067096,0.));
#14996=DIRECTION('ref_axis',(-0.660708878067096,0.750642243977329,0.));
#14997=DIRECTION('',(-0.660708878067096,0.750642243977329,0.));
#14998=DIRECTION('',(0.,0.,1.));
#14999=DIRECTION('',(0.660708878067096,-0.750642243977329,0.));
#15000=DIRECTION('center_axis',(0.,0.,1.));
#15001=DIRECTION('ref_axis',(0.261207001036715,0.965282809651869,0.));
#15002=DIRECTION('center_axis',(0.,0.,-1.));
#15003=DIRECTION('ref_axis',(0.261207001036715,0.965282809651869,0.));
#15004=DIRECTION('',(0.,0.,1.));
#15005=DIRECTION('center_axis',(0.,0.,1.));
#15006=DIRECTION('ref_axis',(0.261207001036715,0.965282809651869,0.));
#15007=DIRECTION('',(0.,0.,-1.));
#15008=DIRECTION('center_axis',(-0.860332693944512,-0.509732925883917,0.));
#15009=DIRECTION('ref_axis',(0.509732925883917,-0.860332693944512,0.));
#15010=DIRECTION('',(0.509732925883917,-0.860332693944512,0.));
#15011=DIRECTION('',(0.,0.,1.));
#15012=DIRECTION('',(0.509732925883917,-0.860332693944512,0.));
#15013=DIRECTION('center_axis',(0.,0.,-1.));
#15014=DIRECTION('ref_axis',(-0.934463820391288,0.356058096916388,0.));
#15015=DIRECTION('center_axis',(0.,0.,1.));
#15016=DIRECTION('ref_axis',(-0.934463820391288,0.356058096916388,0.));
#15017=DIRECTION('',(0.,0.,-1.));
#15018=DIRECTION('center_axis',(0.,0.,-1.));
#15019=DIRECTION('ref_axis',(-0.934463820391288,0.356058096916388,0.));
#15020=DIRECTION('',(0.,0.,1.));
#15021=DIRECTION('center_axis',(0.918073469198192,0.396410273775032,0.));
#15022=DIRECTION('ref_axis',(-0.396410273775032,0.918073469198192,0.));
#15023=DIRECTION('',(-0.396410273775032,0.918073469198192,0.));
#15024=DIRECTION('',(0.,0.,1.));
#15025=DIRECTION('',(0.396410273775032,-0.918073469198192,0.));
#15026=DIRECTION('center_axis',(0.,0.,1.));
#15027=DIRECTION('ref_axis',(0.546711412998308,0.837321103817044,0.));
#15028=DIRECTION('center_axis',(0.,0.,-1.));
#15029=DIRECTION('ref_axis',(0.546711412998308,0.837321103817044,0.));
#15030=DIRECTION('',(0.,0.,1.));
#15031=DIRECTION('center_axis',(0.,0.,1.));
#15032=DIRECTION('ref_axis',(0.546711412998308,0.837321103817044,0.));
#15033=DIRECTION('',(0.,0.,-1.));
#15034=DIRECTION('center_axis',(-0.975741151448288,-0.218927397486859,0.));
#15035=DIRECTION('ref_axis',(0.218927397486859,-0.975741151448288,0.));
#15036=DIRECTION('',(0.218927397486859,-0.975741151448288,0.));
#15037=DIRECTION('',(0.,0.,1.));
#15038=DIRECTION('',(0.218927397486859,-0.975741151448288,0.));
#15039=DIRECTION('center_axis',(0.,0.,-1.));
#15040=DIRECTION('ref_axis',(-0.778699902693228,0.627396574381433,0.));
#15041=DIRECTION('center_axis',(0.,0.,1.));
#15042=DIRECTION('ref_axis',(-0.778699902693228,0.627396574381433,0.));
#15043=DIRECTION('',(0.,0.,-1.));
#15044=DIRECTION('center_axis',(0.,0.,-1.));
#15045=DIRECTION('ref_axis',(-0.778699902693228,0.627396574381433,0.));
#15046=DIRECTION('',(0.,0.,1.));
#15047=DIRECTION('center_axis',(0.995637266659949,0.0933082699330834,0.));
#15048=DIRECTION('ref_axis',(-0.0933082699330834,0.995637266659949,0.));
#15049=DIRECTION('',(-0.0933082699330834,0.995637266659949,0.));
#15050=DIRECTION('',(0.,0.,1.));
#15051=DIRECTION('',(0.0933082699330834,-0.995637266659949,0.));
#15052=DIRECTION('center_axis',(0.,0.,1.));
#15053=DIRECTION('ref_axis',(0.778699902693227,0.627396574381435,0.));
#15054=DIRECTION('center_axis',(0.,0.,-1.));
#15055=DIRECTION('ref_axis',(0.778699902693227,0.627396574381435,0.));
#15056=DIRECTION('',(0.,0.,1.));
#15057=DIRECTION('center_axis',(0.,0.,1.));
#15058=DIRECTION('ref_axis',(0.778699902693227,0.627396574381435,0.));
#15059=DIRECTION('',(0.,0.,-1.));
#15060=DIRECTION('center_axis',(-0.995637266659949,0.0933082699330838,0.));
#15061=DIRECTION('ref_axis',(-0.0933082699330838,-0.995637266659949,0.));
#15062=DIRECTION('',(-0.0933082699330838,-0.995637266659949,0.));
#15063=DIRECTION('',(0.,0.,1.));
#15064=DIRECTION('',(-0.0933082699330838,-0.995637266659949,0.));
#15065=DIRECTION('center_axis',(0.,0.,-1.));
#15066=DIRECTION('ref_axis',(-0.546711412998307,0.837321103817045,0.));
#15067=DIRECTION('center_axis',(0.,0.,1.));
#15068=DIRECTION('ref_axis',(-0.546711412998307,0.837321103817045,0.));
#15069=DIRECTION('',(0.,0.,-1.));
#15070=DIRECTION('center_axis',(0.,0.,-1.));
#15071=DIRECTION('ref_axis',(-0.546711412998307,0.837321103817045,0.));
#15072=DIRECTION('',(0.,0.,1.));
#15073=DIRECTION('center_axis',(0.975741151448288,-0.21892739748686,0.));
#15074=DIRECTION('ref_axis',(0.21892739748686,0.975741151448288,0.));
#15075=DIRECTION('',(0.218927397486859,0.975741151448288,0.));
#15076=DIRECTION('',(0.,0.,1.));
#15077=DIRECTION('',(-0.218927397486859,-0.975741151448288,0.));
#15078=DIRECTION('center_axis',(0.,0.,1.));
#15079=DIRECTION('ref_axis',(0.934463820391285,0.356058096916394,0.));
#15080=DIRECTION('center_axis',(0.,0.,-1.));
#15081=DIRECTION('ref_axis',(0.934463820391285,0.356058096916394,0.));
#15082=DIRECTION('',(0.,0.,1.));
#15083=DIRECTION('center_axis',(0.,0.,1.));
#15084=DIRECTION('ref_axis',(0.934463820391285,0.356058096916394,0.));
#15085=DIRECTION('',(0.,0.,-1.));
#15086=DIRECTION('center_axis',(-0.918073469198192,0.396410273775032,0.));
#15087=DIRECTION('ref_axis',(-0.396410273775032,-0.918073469198192,0.));
#15088=DIRECTION('',(-0.396410273775032,-0.918073469198192,0.));
#15089=DIRECTION('',(0.,0.,1.));
#15090=DIRECTION('',(-0.396410273775032,-0.918073469198192,0.));
#15091=DIRECTION('center_axis',(0.,0.,-1.));
#15092=DIRECTION('ref_axis',(-0.261207001036714,0.965282809651869,0.));
#15093=DIRECTION('center_axis',(0.,0.,1.));
#15094=DIRECTION('ref_axis',(-0.261207001036714,0.965282809651869,0.));
#15095=DIRECTION('',(0.,0.,-1.));
#15096=DIRECTION('center_axis',(0.,0.,-1.));
#15097=DIRECTION('ref_axis',(-0.261207001036714,0.965282809651869,0.));
#15098=DIRECTION('',(0.,0.,1.));
#15099=DIRECTION('center_axis',(0.860332693944512,-0.509732925883917,0.));
#15100=DIRECTION('ref_axis',(0.509732925883917,0.860332693944512,0.));
#15101=DIRECTION('',(0.509732925883917,0.860332693944512,0.));
#15102=DIRECTION('',(0.,0.,1.));
#15103=DIRECTION('',(-0.509732925883917,-0.860332693944512,0.));
#15104=DIRECTION('center_axis',(0.,0.,1.));
#15105=DIRECTION('ref_axis',(0.998755908557164,0.0498661721225399,0.));
#15106=DIRECTION('center_axis',(0.,0.,-1.));
#15107=DIRECTION('ref_axis',(0.998755908557164,0.0498661721225399,0.));
#15108=DIRECTION('',(0.,0.,1.));
#15109=DIRECTION('center_axis',(0.,0.,1.));
#15110=DIRECTION('ref_axis',(0.998755908557164,0.0498661721225399,0.));
#15111=DIRECTION('',(0.,0.,-1.));
#15112=DIRECTION('center_axis',(-0.750642243977328,0.660708878067096,0.));
#15113=DIRECTION('ref_axis',(-0.660708878067096,-0.750642243977328,0.));
#15114=DIRECTION('',(-0.660708878067096,-0.750642243977328,0.));
#15115=DIRECTION('',(0.,0.,1.));
#15116=DIRECTION('',(-0.660708878067096,-0.750642243977328,0.));
#15117=DIRECTION('center_axis',(0.,0.,-1.));
#15118=DIRECTION('ref_axis',(0.0498661721225523,0.998755908557163,0.));
#15119=DIRECTION('center_axis',(0.,0.,1.));
#15120=DIRECTION('ref_axis',(0.0498661721225523,0.998755908557163,0.));
#15121=DIRECTION('',(0.,0.,-1.));
#15122=DIRECTION('center_axis',(0.,0.,-1.));
#15123=DIRECTION('ref_axis',(0.0498661721225523,0.998755908557163,0.));
#15124=DIRECTION('',(0.,0.,1.));
#15125=DIRECTION('center_axis',(0.660708878067096,-0.750642243977329,0.));
#15126=DIRECTION('ref_axis',(0.750642243977329,0.660708878067096,0.));
#15127=DIRECTION('',(0.750642243977329,0.660708878067096,0.));
#15128=DIRECTION('',(0.,0.,1.));
#15129=DIRECTION('',(-0.750642243977329,-0.660708878067096,0.));
#15130=DIRECTION('center_axis',(0.,0.,1.));
#15131=DIRECTION('ref_axis',(0.96528280965187,-0.261207001036712,0.));
#15132=DIRECTION('center_axis',(0.,0.,-1.));
#15133=DIRECTION('ref_axis',(0.96528280965187,-0.261207001036712,0.));
#15134=DIRECTION('',(0.,0.,1.));
#15135=DIRECTION('center_axis',(0.,0.,1.));
#15136=DIRECTION('ref_axis',(0.96528280965187,-0.261207001036712,0.));
#15137=DIRECTION('',(0.,0.,-1.));
#15138=DIRECTION('center_axis',(-0.509732925883917,0.860332693944512,0.));
#15139=DIRECTION('ref_axis',(-0.860332693944512,-0.509732925883917,0.));
#15140=DIRECTION('',(-0.860332693944512,-0.509732925883917,0.));
#15141=DIRECTION('',(0.,0.,1.));
#15142=DIRECTION('',(-0.860332693944512,-0.509732925883917,0.));
#15143=DIRECTION('center_axis',(0.,0.,-1.));
#15144=DIRECTION('ref_axis',(0.356058096916394,0.934463820391285,0.));
#15145=DIRECTION('center_axis',(0.,0.,1.));
#15146=DIRECTION('ref_axis',(0.356058096916394,0.934463820391285,0.));
#15147=DIRECTION('',(0.,0.,-1.));
#15148=DIRECTION('center_axis',(0.,0.,-1.));
#15149=DIRECTION('ref_axis',(0.356058096916394,0.934463820391285,0.));
#15150=DIRECTION('',(0.,0.,1.));
#15151=DIRECTION('center_axis',(0.396410273775032,-0.918073469198192,0.));
#15152=DIRECTION('ref_axis',(0.918073469198192,0.396410273775032,0.));
#15153=DIRECTION('',(0.918073469198192,0.396410273775032,0.));
#15154=DIRECTION('',(0.,0.,1.));
#15155=DIRECTION('',(-0.918073469198192,-0.396410273775032,0.));
#15156=DIRECTION('center_axis',(0.,0.,1.));
#15157=DIRECTION('ref_axis',(0.837321103817046,-0.546711412998306,0.));
#15158=DIRECTION('center_axis',(0.,0.,-1.));
#15159=DIRECTION('ref_axis',(0.837321103817046,-0.546711412998306,0.));
#15160=DIRECTION('',(0.,0.,1.));
#15161=DIRECTION('center_axis',(0.,0.,1.));
#15162=DIRECTION('ref_axis',(0.837321103817046,-0.546711412998306,0.));
#15163=DIRECTION('',(0.,0.,-1.));
#15164=DIRECTION('center_axis',(-0.218927397486859,0.975741151448288,0.));
#15165=DIRECTION('ref_axis',(-0.975741151448288,-0.218927397486859,0.));
#15166=DIRECTION('',(-0.975741151448288,-0.218927397486859,0.));
#15167=DIRECTION('',(0.,0.,1.));
#15168=DIRECTION('',(-0.975741151448288,-0.218927397486859,0.));
#15169=DIRECTION('center_axis',(0.,0.,-1.));
#15170=DIRECTION('ref_axis',(0.627396574381434,0.778699902693227,0.));
#15171=DIRECTION('center_axis',(0.,0.,1.));
#15172=DIRECTION('ref_axis',(0.627396574381434,0.778699902693227,0.));
#15173=DIRECTION('',(0.,0.,-1.));
#15174=DIRECTION('center_axis',(0.,0.,-1.));
#15175=DIRECTION('ref_axis',(0.627396574381434,0.778699902693227,0.));
#15176=DIRECTION('',(0.,0.,1.));
#15177=DIRECTION('center_axis',(0.0933082699330835,-0.995637266659949,0.));
#15178=DIRECTION('ref_axis',(0.995637266659949,0.0933082699330835,0.));
#15179=DIRECTION('',(0.995637266659949,0.0933082699330835,0.));
#15180=DIRECTION('',(0.,0.,1.));
#15181=DIRECTION('',(-0.995637266659949,-0.0933082699330835,0.));
#15182=DIRECTION('center_axis',(0.,0.,1.));
#15183=DIRECTION('ref_axis',(0.627396574381432,-0.778699902693229,0.));
#15184=DIRECTION('center_axis',(0.,0.,-1.));
#15185=DIRECTION('ref_axis',(0.627396574381432,-0.778699902693229,0.));
#15186=DIRECTION('',(0.,0.,1.));
#15187=DIRECTION('center_axis',(0.,0.,1.));
#15188=DIRECTION('ref_axis',(0.627396574381432,-0.778699902693229,0.));
#15189=DIRECTION('',(0.,0.,-1.));
#15190=DIRECTION('center_axis',(0.0933082699330838,0.995637266659949,0.));
#15191=DIRECTION('ref_axis',(-0.995637266659949,0.0933082699330838,0.));
#15192=DIRECTION('',(-0.995637266659949,0.0933082699330838,0.));
#15193=DIRECTION('',(0.,0.,1.));
#15194=DIRECTION('',(-0.995637266659949,0.0933082699330838,0.));
#15195=DIRECTION('center_axis',(0.,0.,-1.));
#15196=DIRECTION('ref_axis',(0.837321103817041,0.546711412998313,0.));
#15197=DIRECTION('center_axis',(0.,0.,1.));
#15198=DIRECTION('ref_axis',(0.837321103817041,0.546711412998313,0.));
#15199=DIRECTION('',(0.,0.,-1.));
#15200=DIRECTION('center_axis',(0.,0.,-1.));
#15201=DIRECTION('ref_axis',(0.837321103817041,0.546711412998313,0.));
#15202=DIRECTION('',(0.,0.,1.));
#15203=DIRECTION('center_axis',(-0.218927397486859,-0.975741151448288,0.));
#15204=DIRECTION('ref_axis',(0.975741151448288,-0.218927397486859,0.));
#15205=DIRECTION('',(0.975741151448288,-0.218927397486859,0.));
#15206=DIRECTION('',(0.,0.,1.));
#15207=DIRECTION('',(-0.975741151448288,0.218927397486859,0.));
#15208=DIRECTION('center_axis',(0.,0.,1.));
#15209=DIRECTION('ref_axis',(0.356058096916391,-0.934463820391286,0.));
#15210=DIRECTION('center_axis',(0.,0.,-1.));
#15211=DIRECTION('ref_axis',(0.356058096916391,-0.934463820391286,0.));
#15212=DIRECTION('',(0.,0.,1.));
#15213=DIRECTION('center_axis',(0.,0.,1.));
#15214=DIRECTION('ref_axis',(0.356058096916391,-0.934463820391286,0.));
#15215=DIRECTION('',(0.,0.,-1.));
#15216=DIRECTION('center_axis',(0.396410273775032,0.918073469198192,0.));
#15217=DIRECTION('ref_axis',(-0.918073469198192,0.396410273775032,0.));
#15218=DIRECTION('',(-0.918073469198192,0.396410273775032,0.));
#15219=DIRECTION('',(0.,0.,1.));
#15220=DIRECTION('',(-0.918073469198192,0.396410273775032,0.));
#15221=DIRECTION('center_axis',(0.,0.,-1.));
#15222=DIRECTION('ref_axis',(0.96528280965187,0.261207001036711,0.));
#15223=DIRECTION('center_axis',(0.,0.,1.));
#15224=DIRECTION('ref_axis',(0.96528280965187,0.261207001036711,0.));
#15225=DIRECTION('',(0.,0.,-1.));
#15226=DIRECTION('center_axis',(0.,0.,-1.));
#15227=DIRECTION('ref_axis',(0.96528280965187,0.261207001036711,0.));
#15228=DIRECTION('',(0.,0.,1.));
#15229=DIRECTION('center_axis',(-0.509732925883917,-0.860332693944512,0.));
#15230=DIRECTION('ref_axis',(0.860332693944512,-0.509732925883917,0.));
#15231=DIRECTION('',(0.860332693944512,-0.509732925883917,0.));
#15232=DIRECTION('',(0.,0.,1.));
#15233=DIRECTION('',(-0.860332693944512,0.509732925883917,0.));
#15234=DIRECTION('center_axis',(0.,0.,1.));
#15235=DIRECTION('ref_axis',(0.0498661721225523,-0.998755908557163,0.));
#15236=DIRECTION('center_axis',(0.,0.,-1.));
#15237=DIRECTION('ref_axis',(0.0498661721225523,-0.998755908557163,0.));
#15238=DIRECTION('',(0.,0.,1.));
#15239=DIRECTION('center_axis',(0.,0.,1.));
#15240=DIRECTION('ref_axis',(0.0498661721225523,-0.998755908557163,0.));
#15241=DIRECTION('',(0.,0.,-1.));
#15242=DIRECTION('center_axis',(0.660708878067096,0.750642243977328,0.));
#15243=DIRECTION('ref_axis',(-0.750642243977328,0.660708878067096,0.));
#15244=DIRECTION('',(-0.750642243977328,0.660708878067096,0.));
#15245=DIRECTION('',(0.,0.,1.));
#15246=DIRECTION('',(-0.750642243977328,0.660708878067096,0.));
#15247=DIRECTION('center_axis',(0.,0.,-1.));
#15248=DIRECTION('ref_axis',(0.998755908557164,-0.0498661721225396,0.));
#15249=DIRECTION('center_axis',(0.,0.,1.));
#15250=DIRECTION('ref_axis',(0.998755908557164,-0.0498661721225396,0.));
#15251=DIRECTION('',(0.,0.,-1.));
#15252=DIRECTION('center_axis',(0.,0.,-1.));
#15253=DIRECTION('ref_axis',(0.998755908557164,-0.0498661721225396,0.));
#15254=DIRECTION('',(0.,0.,1.));
#15255=DIRECTION('center_axis',(-0.750642243977329,-0.660708878067096,0.));
#15256=DIRECTION('ref_axis',(0.660708878067096,-0.750642243977329,0.));
#15257=DIRECTION('',(0.660708878067096,-0.750642243977329,0.));
#15258=DIRECTION('',(0.,0.,1.));
#15259=DIRECTION('',(-0.660708878067096,0.750642243977329,0.));
#15260=DIRECTION('center_axis',(0.,0.,1.));
#15261=DIRECTION('ref_axis',(-0.261207001036715,-0.965282809651869,0.));
#15262=DIRECTION('center_axis',(0.,0.,-1.));
#15263=DIRECTION('ref_axis',(-0.261207001036715,-0.965282809651869,0.));
#15264=DIRECTION('',(0.,0.,1.));
#15265=DIRECTION('center_axis',(0.,0.,1.));
#15266=DIRECTION('ref_axis',(-0.261207001036715,-0.965282809651869,0.));
#15267=DIRECTION('',(0.,0.,-1.));
#15268=DIRECTION('center_axis',(0.860332693944512,0.509732925883917,0.));
#15269=DIRECTION('ref_axis',(-0.509732925883917,0.860332693944512,0.));
#15270=DIRECTION('',(-0.509732925883917,0.860332693944512,0.));
#15271=DIRECTION('',(0.,0.,1.));
#15272=DIRECTION('',(-0.509732925883917,0.860332693944512,0.));
#15273=DIRECTION('center_axis',(0.,0.,-1.));
#15274=DIRECTION('ref_axis',(0.934463820391286,-0.356058096916392,0.));
#15275=DIRECTION('center_axis',(0.,0.,1.));
#15276=DIRECTION('ref_axis',(0.934463820391286,-0.356058096916392,0.));
#15277=DIRECTION('',(0.,0.,-1.));
#15278=DIRECTION('center_axis',(0.,0.,-1.));
#15279=DIRECTION('ref_axis',(0.934463820391286,-0.356058096916392,0.));
#15280=DIRECTION('',(0.,0.,1.));
#15281=DIRECTION('center_axis',(-0.918073469198192,-0.396410273775032,0.));
#15282=DIRECTION('ref_axis',(0.396410273775032,-0.918073469198192,0.));
#15283=DIRECTION('',(0.396410273775032,-0.918073469198192,0.));
#15284=DIRECTION('',(0.,0.,1.));
#15285=DIRECTION('',(-0.396410273775032,0.918073469198192,0.));
#15286=DIRECTION('center_axis',(0.,0.,1.));
#15287=DIRECTION('ref_axis',(-0.546711412998308,-0.837321103817044,0.));
#15288=DIRECTION('center_axis',(0.,0.,-1.));
#15289=DIRECTION('ref_axis',(-0.546711412998308,-0.837321103817044,0.));
#15290=DIRECTION('',(0.,0.,1.));
#15291=DIRECTION('center_axis',(0.,0.,1.));
#15292=DIRECTION('ref_axis',(-0.546711412998308,-0.837321103817044,0.));
#15293=DIRECTION('',(0.,0.,-1.));
#15294=DIRECTION('center_axis',(0.975741151448288,0.218927397486859,0.));
#15295=DIRECTION('ref_axis',(-0.218927397486859,0.975741151448288,0.));
#15296=DIRECTION('',(-0.218927397486859,0.975741151448288,0.));
#15297=DIRECTION('',(0.,0.,1.));
#15298=DIRECTION('',(-0.218927397486859,0.975741151448288,0.));
#15299=DIRECTION('center_axis',(0.,0.,-1.));
#15300=DIRECTION('ref_axis',(0.77869990269323,-0.627396574381431,0.));
#15301=DIRECTION('center_axis',(0.,0.,1.));
#15302=DIRECTION('ref_axis',(0.77869990269323,-0.627396574381431,0.));
#15303=DIRECTION('',(0.,0.,-1.));
#15304=DIRECTION('center_axis',(0.,0.,-1.));
#15305=DIRECTION('ref_axis',(0.77869990269323,-0.627396574381431,0.));
#15306=DIRECTION('',(0.,0.,1.));
#15307=DIRECTION('center_axis',(-0.995637266659949,-0.0933082699330835,
0.));
#15308=DIRECTION('ref_axis',(0.0933082699330835,-0.995637266659949,0.));
#15309=DIRECTION('',(0.0933082699330835,-0.995637266659949,0.));
#15310=DIRECTION('',(0.,0.,1.));
#15311=DIRECTION('',(-0.0933082699330835,0.995637266659949,0.));
#15312=DIRECTION('center_axis',(0.,0.,1.));
#15313=DIRECTION('ref_axis',(-0.77869990269323,-0.627396574381431,0.));
#15314=DIRECTION('center_axis',(0.,0.,-1.));
#15315=DIRECTION('ref_axis',(-0.77869990269323,-0.627396574381431,0.));
#15316=DIRECTION('',(0.,0.,1.));
#15317=DIRECTION('center_axis',(0.,0.,1.));
#15318=DIRECTION('ref_axis',(-0.77869990269323,-0.627396574381431,0.));
#15319=DIRECTION('',(0.,0.,-1.));
#15320=DIRECTION('center_axis',(0.995637266659949,-0.0933082699330837,0.));
#15321=DIRECTION('ref_axis',(0.0933082699330837,0.995637266659949,0.));
#15322=DIRECTION('',(0.0933082699330836,0.995637266659949,0.));
#15323=DIRECTION('',(0.,0.,1.));
#15324=DIRECTION('',(0.0933082699330836,0.995637266659949,0.));
#15325=DIRECTION('center_axis',(0.,0.,-1.));
#15326=DIRECTION('ref_axis',(0.546711412998308,-0.837321103817044,0.));
#15327=DIRECTION('center_axis',(0.,0.,1.));
#15328=DIRECTION('ref_axis',(0.546711412998308,-0.837321103817044,0.));
#15329=DIRECTION('',(0.,0.,-1.));
#15330=DIRECTION('center_axis',(0.,0.,-1.));
#15331=DIRECTION('ref_axis',(0.546711412998308,-0.837321103817044,0.));
#15332=DIRECTION('',(0.,0.,1.));
#15333=DIRECTION('center_axis',(-0.975741151448288,0.218927397486859,0.));
#15334=DIRECTION('ref_axis',(-0.218927397486859,-0.975741151448288,0.));
#15335=DIRECTION('',(-0.218927397486859,-0.975741151448288,0.));
#15336=DIRECTION('',(0.,0.,1.));
#15337=DIRECTION('',(0.218927397486859,0.975741151448288,0.));
#15338=DIRECTION('center_axis',(0.,0.,1.));
#15339=DIRECTION('ref_axis',(-0.934463820391285,-0.356058096916394,0.));
#15340=DIRECTION('center_axis',(0.,0.,-1.));
#15341=DIRECTION('ref_axis',(-0.934463820391285,-0.356058096916394,0.));
#15342=DIRECTION('',(0.,0.,1.));
#15343=DIRECTION('center_axis',(0.,0.,1.));
#15344=DIRECTION('ref_axis',(-0.934463820391285,-0.356058096916394,0.));
#15345=DIRECTION('',(0.,0.,-1.));
#15346=DIRECTION('center_axis',(0.918073469198192,-0.396410273775032,0.));
#15347=DIRECTION('ref_axis',(0.396410273775032,0.918073469198192,0.));
#15348=DIRECTION('',(0.396410273775032,0.918073469198192,0.));
#15349=DIRECTION('',(0.,0.,1.));
#15350=DIRECTION('',(0.396410273775032,0.918073469198192,0.));
#15351=DIRECTION('center_axis',(0.,0.,-1.));
#15352=DIRECTION('ref_axis',(0.261207001036715,-0.965282809651869,0.));
#15353=DIRECTION('center_axis',(0.,0.,1.));
#15354=DIRECTION('ref_axis',(0.261207001036715,-0.965282809651869,0.));
#15355=DIRECTION('',(0.,0.,-1.));
#15356=DIRECTION('center_axis',(0.,0.,-1.));
#15357=DIRECTION('ref_axis',(0.261207001036715,-0.965282809651869,0.));
#15358=DIRECTION('',(0.,0.,1.));
#15359=DIRECTION('center_axis',(-0.860332693944512,0.509732925883917,0.));
#15360=DIRECTION('ref_axis',(-0.509732925883917,-0.860332693944512,0.));
#15361=DIRECTION('',(-0.509732925883917,-0.860332693944512,0.));
#15362=DIRECTION('',(0.,0.,1.));
#15363=DIRECTION('',(0.509732925883917,0.860332693944512,0.));
#15364=DIRECTION('center_axis',(0.,0.,1.));
#15365=DIRECTION('ref_axis',(-0.998755908557164,-0.0498661721225396,0.));
#15366=DIRECTION('center_axis',(0.,0.,-1.));
#15367=DIRECTION('ref_axis',(-0.998755908557164,-0.0498661721225396,0.));
#15368=DIRECTION('',(0.,0.,1.));
#15369=DIRECTION('center_axis',(0.,0.,1.));
#15370=DIRECTION('ref_axis',(-0.998755908557164,-0.0498661721225396,0.));
#15371=DIRECTION('',(0.,0.,-1.));
#15372=DIRECTION('center_axis',(0.750642243977328,-0.660708878067096,0.));
#15373=DIRECTION('ref_axis',(0.660708878067096,0.750642243977328,0.));
#15374=DIRECTION('',(0.660708878067096,0.750642243977328,0.));
#15375=DIRECTION('',(0.,0.,1.));
#15376=DIRECTION('',(0.660708878067096,0.750642243977328,0.));
#15377=DIRECTION('center_axis',(0.,0.,-1.));
#15378=DIRECTION('ref_axis',(-0.0498661721225396,-0.998755908557164,0.));
#15379=DIRECTION('center_axis',(0.,0.,1.));
#15380=DIRECTION('ref_axis',(-0.0498661721225396,-0.998755908557164,0.));
#15381=DIRECTION('',(0.,0.,-1.));
#15382=DIRECTION('center_axis',(0.,0.,-1.));
#15383=DIRECTION('ref_axis',(-0.0498661721225396,-0.998755908557164,0.));
#15384=DIRECTION('',(0.,0.,1.));
#15385=DIRECTION('center_axis',(-0.660708878067096,0.750642243977328,0.));
#15386=DIRECTION('ref_axis',(-0.750642243977328,-0.660708878067096,0.));
#15387=DIRECTION('',(-0.750642243977328,-0.660708878067096,0.));
#15388=DIRECTION('',(0.,0.,1.));
#15389=DIRECTION('',(0.750642243977328,0.660708878067096,0.));
#15390=DIRECTION('center_axis',(0.,0.,1.));
#15391=DIRECTION('ref_axis',(-0.96528280965187,0.261207001036712,0.));
#15392=DIRECTION('center_axis',(0.,0.,-1.));
#15393=DIRECTION('ref_axis',(-0.96528280965187,0.261207001036712,0.));
#15394=DIRECTION('',(0.,0.,1.));
#15395=DIRECTION('center_axis',(0.,0.,1.));
#15396=DIRECTION('ref_axis',(-0.96528280965187,0.261207001036712,0.));
#15397=DIRECTION('',(0.,0.,-1.));
#15398=DIRECTION('center_axis',(0.509732925883917,-0.860332693944512,0.));
#15399=DIRECTION('ref_axis',(0.860332693944512,0.509732925883917,0.));
#15400=DIRECTION('',(0.860332693944512,0.509732925883917,0.));
#15401=DIRECTION('',(0.,0.,1.));
#15402=DIRECTION('',(0.860332693944512,0.509732925883917,0.));
#15403=DIRECTION('center_axis',(0.,0.,-1.));
#15404=DIRECTION('ref_axis',(-0.356058096916394,-0.934463820391285,0.));
#15405=DIRECTION('center_axis',(0.,0.,1.));
#15406=DIRECTION('ref_axis',(-0.356058096916394,-0.934463820391285,0.));
#15407=DIRECTION('',(0.,0.,-1.));
#15408=DIRECTION('center_axis',(0.,0.,-1.));
#15409=DIRECTION('ref_axis',(-0.356058096916394,-0.934463820391285,0.));
#15410=DIRECTION('',(0.,0.,1.));
#15411=DIRECTION('center_axis',(-0.396410273775032,0.918073469198192,0.));
#15412=DIRECTION('ref_axis',(-0.918073469198192,-0.396410273775032,0.));
#15413=DIRECTION('',(-0.918073469198192,-0.396410273775032,0.));
#15414=DIRECTION('',(0.,0.,1.));
#15415=DIRECTION('',(0.918073469198192,0.396410273775032,0.));
#15416=DIRECTION('center_axis',(0.,0.,1.));
#15417=DIRECTION('ref_axis',(-0.837321103817043,0.546711412998309,0.));
#15418=DIRECTION('center_axis',(0.,0.,-1.));
#15419=DIRECTION('ref_axis',(-0.837321103817043,0.546711412998309,0.));
#15420=DIRECTION('',(0.,0.,1.));
#15421=DIRECTION('center_axis',(0.,0.,1.));
#15422=DIRECTION('ref_axis',(-0.837321103817043,0.546711412998309,0.));
#15423=DIRECTION('',(0.,0.,-1.));
#15424=DIRECTION('center_axis',(0.218927397486859,-0.975741151448288,0.));
#15425=DIRECTION('ref_axis',(0.975741151448288,0.218927397486859,0.));
#15426=DIRECTION('',(0.975741151448288,0.218927397486859,0.));
#15427=DIRECTION('',(0.,0.,1.));
#15428=DIRECTION('',(0.975741151448288,0.218927397486859,0.));
#15429=DIRECTION('',(0.,0.,1.));
#15430=DIRECTION('center_axis',(0.,0.,1.));
#15431=DIRECTION('ref_axis',(0.940823330106451,-0.338897420361099,0.));
#15432=DIRECTION('center_axis',(0.,0.,1.));
#15433=DIRECTION('ref_axis',(0.940823330106451,-0.338897420361099,0.));
#15434=DIRECTION('center_axis',(0.,0.,1.));
#15435=DIRECTION('ref_axis',(0.940823330106451,-0.338897420361099,0.));
#15436=DIRECTION('',(0.,0.,1.));
#15437=DIRECTION('',(0.,0.,1.));
#15438=DIRECTION('center_axis',(0.,0.,1.));
#15439=DIRECTION('ref_axis',(0.790051096538837,-0.613040997697366,0.));
#15440=DIRECTION('center_axis',(0.,0.,1.));
#15441=DIRECTION('ref_axis',(0.790051096538837,-0.613040997697366,0.));
#15442=DIRECTION('center_axis',(0.,0.,1.));
#15443=DIRECTION('ref_axis',(0.790051096538837,-0.613040997697366,0.));
#15444=DIRECTION('',(0.,0.,1.));
#15445=DIRECTION('',(0.,0.,1.));
#15446=DIRECTION('center_axis',(0.,0.,1.));
#15447=DIRECTION('ref_axis',(0.561943157032333,-0.827175850871225,0.));
#15448=DIRECTION('center_axis',(0.,0.,1.));
#15449=DIRECTION('ref_axis',(0.561943157032333,-0.827175850871225,0.));
#15450=DIRECTION('center_axis',(0.,0.,1.));
#15451=DIRECTION('ref_axis',(0.561943157032333,-0.827175850871225,0.));
#15452=DIRECTION('',(0.,0.,1.));
#15453=DIRECTION('',(0.,0.,1.));
#15454=DIRECTION('center_axis',(0.,0.,1.));
#15455=DIRECTION('ref_axis',(0.278828306027306,-0.960340968488767,0.));
#15456=DIRECTION('center_axis',(0.,0.,1.));
#15457=DIRECTION('ref_axis',(0.278828306027306,-0.960340968488767,0.));
#15458=DIRECTION('center_axis',(0.,0.,1.));
#15459=DIRECTION('ref_axis',(0.278828306027306,-0.960340968488767,0.));
#15460=DIRECTION('',(0.,0.,1.));
#15461=DIRECTION('',(0.,0.,1.));
#15462=DIRECTION('center_axis',(0.,0.,1.));
#15463=DIRECTION('ref_axis',(-0.0315802022827165,-0.999501221021657,0.));
#15464=DIRECTION('center_axis',(0.,0.,1.));
#15465=DIRECTION('ref_axis',(-0.0315802022827165,-0.999501221021657,0.));
#15466=DIRECTION('center_axis',(0.,0.,1.));
#15467=DIRECTION('ref_axis',(-0.0315802022827165,-0.999501221021657,0.));
#15468=DIRECTION('',(0.,0.,1.));
#15469=DIRECTION('',(0.,0.,1.));
#15470=DIRECTION('center_axis',(0.,0.,1.));
#15471=DIRECTION('ref_axis',(-0.338897420361099,-0.940823330106451,0.));
#15472=DIRECTION('center_axis',(0.,0.,1.));
#15473=DIRECTION('ref_axis',(-0.338897420361099,-0.940823330106451,0.));
#15474=DIRECTION('center_axis',(0.,0.,1.));
#15475=DIRECTION('ref_axis',(-0.338897420361099,-0.940823330106451,0.));
#15476=DIRECTION('',(0.,0.,1.));
#15477=DIRECTION('',(0.,0.,1.));
#15478=DIRECTION('center_axis',(0.,0.,1.));
#15479=DIRECTION('ref_axis',(-0.613040997697366,-0.790051096538837,0.));
#15480=DIRECTION('center_axis',(0.,0.,1.));
#15481=DIRECTION('ref_axis',(-0.613040997697366,-0.790051096538837,0.));
#15482=DIRECTION('center_axis',(0.,0.,1.));
#15483=DIRECTION('ref_axis',(-0.613040997697366,-0.790051096538837,0.));
#15484=DIRECTION('',(0.,0.,1.));
#15485=DIRECTION('',(0.,0.,1.));
#15486=DIRECTION('center_axis',(0.,0.,1.));
#15487=DIRECTION('ref_axis',(-0.827175850871225,-0.561943157032333,0.));
#15488=DIRECTION('center_axis',(0.,0.,1.));
#15489=DIRECTION('ref_axis',(-0.827175850871225,-0.561943157032333,0.));
#15490=DIRECTION('center_axis',(0.,0.,1.));
#15491=DIRECTION('ref_axis',(-0.827175850871225,-0.561943157032333,0.));
#15492=DIRECTION('',(0.,0.,1.));
#15493=DIRECTION('',(0.,0.,1.));
#15494=DIRECTION('center_axis',(0.,0.,1.));
#15495=DIRECTION('ref_axis',(-0.960340968488767,-0.278828306027306,0.));
#15496=DIRECTION('center_axis',(0.,0.,1.));
#15497=DIRECTION('ref_axis',(-0.960340968488767,-0.278828306027306,0.));
#15498=DIRECTION('center_axis',(0.,0.,1.));
#15499=DIRECTION('ref_axis',(-0.960340968488767,-0.278828306027306,0.));
#15500=DIRECTION('',(0.,0.,1.));
#15501=DIRECTION('',(0.,0.,1.));
#15502=DIRECTION('center_axis',(0.,0.,1.));
#15503=DIRECTION('ref_axis',(-0.999501221021657,0.0315802022827165,0.));
#15504=DIRECTION('center_axis',(0.,0.,1.));
#15505=DIRECTION('ref_axis',(-0.999501221021657,0.0315802022827165,0.));
#15506=DIRECTION('center_axis',(0.,0.,1.));
#15507=DIRECTION('ref_axis',(-0.999501221021657,0.0315802022827165,0.));
#15508=DIRECTION('',(0.,0.,1.));
#15509=DIRECTION('',(0.,0.,1.));
#15510=DIRECTION('center_axis',(0.,0.,1.));
#15511=DIRECTION('ref_axis',(-0.940823330106451,0.338897420361099,0.));
#15512=DIRECTION('center_axis',(0.,0.,1.));
#15513=DIRECTION('ref_axis',(-0.940823330106451,0.338897420361099,0.));
#15514=DIRECTION('center_axis',(0.,0.,1.));
#15515=DIRECTION('ref_axis',(-0.940823330106451,0.338897420361099,0.));
#15516=DIRECTION('',(0.,0.,1.));
#15517=DIRECTION('',(0.,0.,1.));
#15518=DIRECTION('center_axis',(0.,0.,1.));
#15519=DIRECTION('ref_axis',(-0.790051096538837,0.613040997697366,0.));
#15520=DIRECTION('center_axis',(0.,0.,1.));
#15521=DIRECTION('ref_axis',(-0.790051096538837,0.613040997697366,0.));
#15522=DIRECTION('center_axis',(0.,0.,1.));
#15523=DIRECTION('ref_axis',(-0.790051096538837,0.613040997697366,0.));
#15524=DIRECTION('',(0.,0.,1.));
#15525=DIRECTION('',(0.,0.,1.));
#15526=DIRECTION('center_axis',(0.,0.,1.));
#15527=DIRECTION('ref_axis',(-0.561943157032333,0.827175850871225,0.));
#15528=DIRECTION('center_axis',(0.,0.,1.));
#15529=DIRECTION('ref_axis',(-0.561943157032333,0.827175850871225,0.));
#15530=DIRECTION('center_axis',(0.,0.,1.));
#15531=DIRECTION('ref_axis',(-0.561943157032333,0.827175850871225,0.));
#15532=DIRECTION('',(0.,0.,1.));
#15533=DIRECTION('',(0.,0.,1.));
#15534=DIRECTION('center_axis',(0.,0.,1.));
#15535=DIRECTION('ref_axis',(-0.278828306027306,0.960340968488767,0.));
#15536=DIRECTION('center_axis',(0.,0.,1.));
#15537=DIRECTION('ref_axis',(-0.278828306027306,0.960340968488767,0.));
#15538=DIRECTION('center_axis',(0.,0.,1.));
#15539=DIRECTION('ref_axis',(-0.278828306027306,0.960340968488767,0.));
#15540=DIRECTION('',(0.,0.,1.));
#15541=DIRECTION('',(0.,0.,1.));
#15542=DIRECTION('center_axis',(0.,0.,1.));
#15543=DIRECTION('ref_axis',(0.0315802022827164,0.999501221021657,0.));
#15544=DIRECTION('center_axis',(0.,0.,1.));
#15545=DIRECTION('ref_axis',(0.0315802022827164,0.999501221021657,0.));
#15546=DIRECTION('center_axis',(0.,0.,1.));
#15547=DIRECTION('ref_axis',(0.0315802022827164,0.999501221021657,0.));
#15548=DIRECTION('',(0.,0.,1.));
#15549=DIRECTION('',(0.,0.,1.));
#15550=DIRECTION('center_axis',(0.,0.,1.));
#15551=DIRECTION('ref_axis',(0.338897420361099,0.940823330106451,0.));
#15552=DIRECTION('center_axis',(0.,0.,1.));
#15553=DIRECTION('ref_axis',(0.338897420361099,0.940823330106451,0.));
#15554=DIRECTION('center_axis',(0.,0.,1.));
#15555=DIRECTION('ref_axis',(0.338897420361099,0.940823330106451,0.));
#15556=DIRECTION('',(0.,0.,1.));
#15557=DIRECTION('',(0.,0.,1.));
#15558=DIRECTION('center_axis',(0.,0.,1.));
#15559=DIRECTION('ref_axis',(0.613040997697366,0.790051096538837,0.));
#15560=DIRECTION('center_axis',(0.,0.,1.));
#15561=DIRECTION('ref_axis',(0.613040997697366,0.790051096538837,0.));
#15562=DIRECTION('center_axis',(0.,0.,1.));
#15563=DIRECTION('ref_axis',(0.613040997697366,0.790051096538837,0.));
#15564=DIRECTION('',(0.,0.,1.));
#15565=DIRECTION('',(0.,0.,1.));
#15566=DIRECTION('center_axis',(0.,0.,1.));
#15567=DIRECTION('ref_axis',(0.827175850871225,0.561943157032333,0.));
#15568=DIRECTION('center_axis',(0.,0.,1.));
#15569=DIRECTION('ref_axis',(0.827175850871225,0.561943157032333,0.));
#15570=DIRECTION('center_axis',(0.,0.,1.));
#15571=DIRECTION('ref_axis',(0.827175850871225,0.561943157032333,0.));
#15572=DIRECTION('',(0.,0.,1.));
#15573=DIRECTION('',(0.,0.,1.));
#15574=DIRECTION('center_axis',(0.,0.,1.));
#15575=DIRECTION('ref_axis',(0.960340968488767,0.278828306027306,0.));
#15576=DIRECTION('center_axis',(0.,0.,1.));
#15577=DIRECTION('ref_axis',(0.960340968488767,0.278828306027306,0.));
#15578=DIRECTION('center_axis',(0.,0.,1.));
#15579=DIRECTION('ref_axis',(0.960340968488767,0.278828306027306,0.));
#15580=DIRECTION('',(0.,0.,1.));
#15581=DIRECTION('center_axis',(0.,0.,1.));
#15582=DIRECTION('ref_axis',(1.,0.,0.));
#15583=DIRECTION('center_axis',(0.,0.,1.));
#15584=DIRECTION('ref_axis',(1.,0.,0.));
#15585=DIRECTION('center_axis',(0.,0.,1.));
#15586=DIRECTION('ref_axis',(1.,0.,0.));
#15587=DIRECTION('center_axis',(0.,0.,1.));
#15588=DIRECTION('ref_axis',(1.,0.,0.));
#15589=DIRECTION('center_axis',(0.,0.,1.));
#15590=DIRECTION('ref_axis',(1.,0.,0.));
#15591=DIRECTION('center_axis',(0.,0.,1.));
#15592=DIRECTION('ref_axis',(1.,0.,0.));
#15593=DIRECTION('center_axis',(0.,0.,1.));
#15594=DIRECTION('ref_axis',(1.,0.,0.));
#15595=DIRECTION('center_axis',(0.,0.,1.));
#15596=DIRECTION('ref_axis',(1.,0.,0.));
#15597=DIRECTION('center_axis',(0.,0.,1.));
#15598=DIRECTION('ref_axis',(1.,0.,0.));
#15599=DIRECTION('center_axis',(0.,0.,1.));
#15600=DIRECTION('ref_axis',(1.,0.,0.));
#15601=DIRECTION('center_axis',(0.,0.,1.));
#15602=DIRECTION('ref_axis',(1.,0.,0.));
#15603=DIRECTION('center_axis',(0.,0.,1.));
#15604=DIRECTION('ref_axis',(1.,0.,0.));
#15605=DIRECTION('center_axis',(0.,0.,1.));
#15606=DIRECTION('ref_axis',(1.,0.,0.));
#15607=DIRECTION('center_axis',(0.,0.,1.));
#15608=DIRECTION('ref_axis',(1.,0.,0.));
#15609=DIRECTION('center_axis',(0.,0.,1.));
#15610=DIRECTION('ref_axis',(1.,0.,0.));
#15611=DIRECTION('center_axis',(0.,0.,1.));
#15612=DIRECTION('ref_axis',(1.,0.,0.));
#15613=DIRECTION('center_axis',(0.,0.,1.));
#15614=DIRECTION('ref_axis',(1.,0.,0.));
#15615=DIRECTION('center_axis',(0.,0.,1.));
#15616=DIRECTION('ref_axis',(1.,0.,0.));
#15617=DIRECTION('center_axis',(0.,0.,1.));
#15618=DIRECTION('ref_axis',(1.,0.,0.));
#15619=DIRECTION('center_axis',(0.,0.,-1.));
#15620=DIRECTION('ref_axis',(-0.627396574381432,-0.778699902693229,0.));
#15621=DIRECTION('',(0.995637266659949,0.0933082699330836,0.));
#15622=DIRECTION('center_axis',(0.,0.,1.));
#15623=DIRECTION('ref_axis',(0.999501221021657,-0.0315802022827163,0.));
#15624=DIRECTION('',(0.995637266659949,-0.0933082699330836,0.));
#15625=DIRECTION('center_axis',(0.,0.,-1.));
#15626=DIRECTION('ref_axis',(-0.627396574381432,0.778699902693229,0.));
#15627=DIRECTION('center_axis',(0.,0.,1.));
#15628=DIRECTION('ref_axis',(1.,0.,0.));
#15629=DIRECTION('center_axis',(0.,0.,1.));
#15630=DIRECTION('ref_axis',(1.,0.,0.));
#15631=DIRECTION('center_axis',(0.,0.,1.));
#15632=DIRECTION('ref_axis',(1.,0.,0.));
#15633=DIRECTION('center_axis',(0.,0.,1.));
#15634=DIRECTION('ref_axis',(1.,0.,0.));
#15635=DIRECTION('center_axis',(0.,0.,1.));
#15636=DIRECTION('ref_axis',(-0.627396574381432,0.778699902693229,0.));
#15637=DIRECTION('',(0.995637266659949,-0.0933082699330836,0.));
#15638=DIRECTION('center_axis',(0.,0.,1.));
#15639=DIRECTION('ref_axis',(0.999501221021657,-0.0315802022827163,0.));
#15640=DIRECTION('',(-0.995637266659949,-0.0933082699330836,0.));
#15641=DIRECTION('center_axis',(0.,0.,1.));
#15642=DIRECTION('ref_axis',(-0.627396574381432,-0.778699902693229,0.));
#15643=DIRECTION('center_axis',(0.,0.,1.));
#15644=DIRECTION('ref_axis',(1.,0.,0.));
#15645=DIRECTION('center_axis',(0.,0.,1.));
#15646=DIRECTION('ref_axis',(1.,0.,0.));
#15647=DIRECTION('center_axis',(0.,0.,1.));
#15648=DIRECTION('ref_axis',(1.,0.,0.));
#15649=DIRECTION('center_axis',(0.,0.,1.));
#15650=DIRECTION('ref_axis',(1.,0.,0.));
#15651=DIRECTION('center_axis',(0.,0.,1.));
#15652=DIRECTION('ref_axis',(1.,0.,0.));
#15653=DIRECTION('center_axis',(0.,0.,1.));
#15654=DIRECTION('ref_axis',(1.,0.,0.));
#15655=DIRECTION('center_axis',(0.,0.,1.));
#15656=DIRECTION('ref_axis',(1.,0.,0.));
#15657=DIRECTION('center_axis',(0.,0.,1.));
#15658=DIRECTION('ref_axis',(1.,0.,0.));
#15659=DIRECTION('center_axis',(0.,0.,1.));
#15660=DIRECTION('ref_axis',(1.,0.,0.));
#15661=DIRECTION('center_axis',(0.,0.,1.));
#15662=DIRECTION('ref_axis',(1.,0.,0.));
#15663=DIRECTION('center_axis',(0.,0.,1.));
#15664=DIRECTION('ref_axis',(1.,0.,0.));
#15665=DIRECTION('center_axis',(0.,0.,1.));
#15666=DIRECTION('ref_axis',(1.,0.,0.));
#15667=DIRECTION('center_axis',(0.,0.,1.));
#15668=DIRECTION('ref_axis',(1.,0.,0.));
#15669=DIRECTION('center_axis',(0.,0.,1.));
#15670=DIRECTION('ref_axis',(1.,0.,0.));
#15671=DIRECTION('center_axis',(0.,0.,1.));
#15672=DIRECTION('ref_axis',(1.,0.,0.));
#15673=DIRECTION('center_axis',(0.,0.,1.));
#15674=DIRECTION('ref_axis',(1.,0.,0.));
#15675=DIRECTION('center_axis',(0.,0.,1.));
#15676=DIRECTION('ref_axis',(1.,0.,0.));
#15677=DIRECTION('center_axis',(0.,0.,1.));
#15678=DIRECTION('ref_axis',(1.,0.,0.));
#15679=DIRECTION('center_axis',(0.,0.,1.));
#15680=DIRECTION('ref_axis',(1.,0.,0.));
#15681=DIRECTION('center_axis',(0.,0.,1.));
#15682=DIRECTION('ref_axis',(1.,0.,0.));
#15683=DIRECTION('',(0.,0.,1.));
#15684=DIRECTION('center_axis',(0.,0.,1.));
#15685=DIRECTION('ref_axis',(1.,0.,0.));
#15686=DIRECTION('center_axis',(0.,0.,1.));
#15687=DIRECTION('ref_axis',(1.,0.,0.));
#15688=DIRECTION('center_axis',(0.,0.,1.));
#15689=DIRECTION('ref_axis',(1.,0.,0.));
#15690=DIRECTION('center_axis',(0.,0.,1.));
#15691=DIRECTION('ref_axis',(1.,0.,0.));
#15692=DIRECTION('center_axis',(0.,0.,1.));
#15693=DIRECTION('ref_axis',(1.,0.,0.));
#15694=DIRECTION('center_axis',(0.,0.,1.));
#15695=DIRECTION('ref_axis',(1.,0.,0.));
#15696=DIRECTION('center_axis',(0.,0.,1.));
#15697=DIRECTION('ref_axis',(1.,0.,0.));
#15698=DIRECTION('center_axis',(0.,0.,1.));
#15699=DIRECTION('ref_axis',(1.,0.,0.));
#15700=DIRECTION('center_axis',(0.,0.,1.));
#15701=DIRECTION('ref_axis',(1.,0.,0.));
#15702=DIRECTION('center_axis',(0.,0.,1.));
#15703=DIRECTION('ref_axis',(1.,0.,0.));
#15704=DIRECTION('center_axis',(0.,0.,1.));
#15705=DIRECTION('ref_axis',(1.,0.,0.));
#15706=DIRECTION('center_axis',(0.,0.,1.));
#15707=DIRECTION('ref_axis',(1.,0.,0.));
#15708=DIRECTION('center_axis',(0.,0.,1.));
#15709=DIRECTION('ref_axis',(1.,0.,0.));
#15710=DIRECTION('center_axis',(0.,0.,1.));
#15711=DIRECTION('ref_axis',(1.,0.,0.));
#15712=DIRECTION('center_axis',(0.,0.,1.));
#15713=DIRECTION('ref_axis',(1.,0.,0.));
#15714=DIRECTION('center_axis',(0.,0.,1.));
#15715=DIRECTION('ref_axis',(1.,0.,0.));
#15716=DIRECTION('center_axis',(0.,0.,1.));
#15717=DIRECTION('ref_axis',(1.,0.,0.));
#15718=DIRECTION('center_axis',(0.,0.,1.));
#15719=DIRECTION('ref_axis',(1.,0.,0.));
#15720=DIRECTION('center_axis',(0.,0.,-1.));
#15721=DIRECTION('ref_axis',(-0.627396574381432,-0.778699902693229,0.));
#15722=DIRECTION('',(0.,0.,-1.));
#15723=DIRECTION('center_axis',(-0.0933082699330836,0.995637266659949,0.));
#15724=DIRECTION('ref_axis',(-0.995637266659949,-0.0933082699330836,0.));
#15725=DIRECTION('',(0.,0.,1.));
#15726=DIRECTION('center_axis',(0.,0.,1.));
#15727=DIRECTION('ref_axis',(-0.627396574381432,0.778699902693229,0.));
#15728=DIRECTION('',(0.,0.,1.));
#15729=DIRECTION('',(0.,0.,-1.));
#15730=DIRECTION('center_axis',(-0.0933082699330836,-0.995637266659949,
0.));
#15731=DIRECTION('ref_axis',(0.995637266659949,-0.0933082699330836,0.));
#15732=DIRECTION('',(0.,0.,1.));
#15733=DIRECTION('',(0.,0.,1.));
#15734=DIRECTION('center_axis',(0.,0.,1.));
#15735=DIRECTION('ref_axis',(0.999501221021657,-0.0315802022827163,0.));
#15736=DIRECTION('',(0.,0.,1.));
#15737=DIRECTION('center_axis',(0.,0.,1.));
#15738=DIRECTION('ref_axis',(1.,0.,0.));
#18820=CARTESIAN_POINT('',(0.,0.,0.));
#18821=CARTESIAN_POINT('Origin',(0.,3.33066907387547E-15,7.50000243576834));
#18822=CARTESIAN_POINT('',(-7.5,4.09394740330526E-15,15.0000024357683));
#18823=CARTESIAN_POINT('Origin',(0.,2.98372437868011E-15,15.0000024357683));
#18824=CARTESIAN_POINT('',(-7.5,1.6739163200269E-14,57.5000024357683));
#18825=CARTESIAN_POINT('',(-7.5,4.24915417323598E-15,7.50000243576834));
#18826=CARTESIAN_POINT('Origin',(0.,1.58206781009085E-14,57.5000024357683));
#18827=CARTESIAN_POINT('Origin',(0.,3.33066907387547E-15,7.50000243576834));
#18828=CARTESIAN_POINT('',(-7.5,-8.49065503433768E-15,-43.4999975642317));
#18829=CARTESIAN_POINT('Origin',(0.,-9.4091401336982E-15,-43.4999975642317));
#18830=CARTESIAN_POINT('',(-7.5,3.46944695195362E-16,2.43576833591774E-6));
#18831=CARTESIAN_POINT('',(-7.5,4.24915417323598E-15,7.50000243576834));
#18832=CARTESIAN_POINT('Origin',(0.,-7.63278329429795E-16,2.43576833591774E-6));
#18833=CARTESIAN_POINT('Origin',(0.,1.69309011255336E-14,57.5000024357683));
#18834=CARTESIAN_POINT('Origin',(0.,-8.29891710907304E-15,-43.4999975642317));
#18835=CARTESIAN_POINT('Origin',(35.6951686664485,-6.98407602147876,0.));
#18836=CARTESIAN_POINT('',(34.7137772481474,-6.79205809501118,15.));
#18837=CARTESIAN_POINT('',(35.4762412689616,-7.95981717292705,15.));
#18838=CARTESIAN_POINT('Origin',(35.6951686664485,-6.98407602147876,15.));
#18839=CARTESIAN_POINT('',(35.4762412689616,-7.95981717292705,0.));
#18840=CARTESIAN_POINT('',(35.4762412689616,-7.95981717292705,0.));
#18841=CARTESIAN_POINT('',(34.7137772481474,-6.79205809501118,0.));
#18842=CARTESIAN_POINT('Origin',(35.6951686664485,-6.98407602147876,0.));
#18843=CARTESIAN_POINT('',(34.7137772481474,-6.79205809501118,0.));
#18844=CARTESIAN_POINT('Origin',(36.6758703925241,-8.22897839625062,0.));
#18845=CARTESIAN_POINT('',(36.6758703925241,-8.22897839625062,15.));
#18846=CARTESIAN_POINT('',(34.5041585975144,-7.74171062993033,15.));
#18847=CARTESIAN_POINT('',(36.6758703925241,-8.22897839625062,0.));
#18848=CARTESIAN_POINT('',(36.6758703925241,-8.22897839625062,0.));
#18849=CARTESIAN_POINT('',(34.5041585975144,-7.74171062993033,0.));
#18850=CARTESIAN_POINT('Origin',(32.9831349545516,-15.3308575288479,0.));
#18851=CARTESIAN_POINT('',(32.0763073136589,-14.909355892181,0.));
#18852=CARTESIAN_POINT('',(33.3795452283267,-14.4127840596497,0.));
#18853=CARTESIAN_POINT('Origin',(32.9831349545516,-15.3308575288479,0.));
#18854=CARTESIAN_POINT('',(33.3795452283267,-14.4127840596497,15.));
#18855=CARTESIAN_POINT('',(33.3795452283267,-14.4127840596497,0.));
#18856=CARTESIAN_POINT('',(32.0763073136589,-14.909355892181,15.));
#18857=CARTESIAN_POINT('Origin',(32.9831349545516,-15.3308575288479,15.));
#18858=CARTESIAN_POINT('',(32.0763073136589,-14.909355892181,0.));
#18859=CARTESIAN_POINT('Origin',(32.4649140177865,-14.0178601012327,0.));
#18860=CARTESIAN_POINT('',(34.5082745737944,-14.9001523628048,0.));
#18861=CARTESIAN_POINT('',(32.4649140177865,-14.0178601012327,0.));
#18862=CARTESIAN_POINT('',(34.5082745737944,-14.9001523628048,15.));
#18863=CARTESIAN_POINT('',(34.5082745737944,-14.9001523628048,0.));
#18864=CARTESIAN_POINT('',(32.4649140177865,-14.0178601012327,15.));
#18865=CARTESIAN_POINT('Origin',(31.7899245798369,-17.6726647455408,0.));
#18866=CARTESIAN_POINT('',(30.9159026789286,-17.1867782189396,15.));
#18867=CARTESIAN_POINT('',(31.280191653953,-18.5329974394853,15.));
#18868=CARTESIAN_POINT('Origin',(31.7899245798369,-17.6726647455408,15.));
#18869=CARTESIAN_POINT('',(31.280191653953,-18.5329974394853,0.));
#18870=CARTESIAN_POINT('',(31.280191653953,-18.5329974394853,0.));
#18871=CARTESIAN_POINT('',(30.9159026789286,-17.1867782189396,0.));
#18872=CARTESIAN_POINT('Origin',(31.7899245798369,-17.6726647455408,0.));
#18873=CARTESIAN_POINT('',(30.9159026789286,-17.1867782189396,0.));
#18874=CARTESIAN_POINT('Origin',(32.3379313568208,-19.1596907609891,0.));
#18875=CARTESIAN_POINT('',(32.3379313568208,-19.1596907609891,15.));
#18876=CARTESIAN_POINT('',(30.4230847232658,-18.0251757251071,15.));
#18877=CARTESIAN_POINT('',(32.3379313568208,-19.1596907609891,0.));
#18878=CARTESIAN_POINT('',(32.3379313568208,-19.1596907609891,0.));
#18879=CARTESIAN_POINT('',(30.4230847232658,-18.0251757251071,0.));
#18880=CARTESIAN_POINT('Origin',(26.6313299116137,-24.7728611819223,0.));
#18881=CARTESIAN_POINT('',(25.899136743473,-24.0917641517363,0.));
#18882=CARTESIAN_POINT('',(27.2920387896808,-24.0222189379449,0.));
#18883=CARTESIAN_POINT('Origin',(26.6313299116137,-24.7728611819223,0.));
#18884=CARTESIAN_POINT('',(27.2920387896808,-24.0222189379449,15.));
#18885=CARTESIAN_POINT('',(27.2920387896808,-24.0222189379449,0.));
#18886=CARTESIAN_POINT('',(25.899136743473,-24.0917641517363,15.));
#18887=CARTESIAN_POINT('Origin',(26.6313299116137,-24.7728611819223,15.));
#18888=CARTESIAN_POINT('',(25.899136743473,-24.0917641517363,0.));
#18889=CARTESIAN_POINT('Origin',(26.5442110315263,-23.3639873462087,0.));
#18890=CARTESIAN_POINT('',(28.2149191006268,-24.8345302882955,0.));
#18891=CARTESIAN_POINT('',(26.5442110315263,-23.3639873462087,0.));
#18892=CARTESIAN_POINT('',(28.2149191006268,-24.8345302882955,15.));
#18893=CARTESIAN_POINT('',(28.2149191006268,-24.8345302882955,0.));
#18894=CARTESIAN_POINT('',(26.5442110315263,-23.3639873462087,15.));
#18895=CARTESIAN_POINT('Origin',(24.7728611819222,-26.6313299116137,0.));
#18896=CARTESIAN_POINT('',(24.0917641517363,-25.899136743473,15.));
#18897=CARTESIAN_POINT('',(24.0222189379449,-27.2920387896808,15.));
#18898=CARTESIAN_POINT('Origin',(24.7728611819222,-26.6313299116137,15.));
#18899=CARTESIAN_POINT('',(24.0222189379449,-27.2920387896808,0.));
#18900=CARTESIAN_POINT('',(24.0222189379449,-27.2920387896808,0.));
#18901=CARTESIAN_POINT('',(24.0917641517363,-25.899136743473,0.));
#18902=CARTESIAN_POINT('Origin',(24.7728611819222,-26.6313299116137,0.));
#18903=CARTESIAN_POINT('',(24.0917641517363,-25.899136743473,0.));
#18904=CARTESIAN_POINT('Origin',(24.8345302882955,-28.2149191006269,0.));
#18905=CARTESIAN_POINT('',(24.8345302882955,-28.2149191006269,15.));
#18906=CARTESIAN_POINT('',(23.3639873462086,-26.5442110315263,15.));
#18907=CARTESIAN_POINT('',(24.8345302882955,-28.2149191006269,0.));
#18908=CARTESIAN_POINT('',(24.8345302882955,-28.2149191006269,0.));
#18909=CARTESIAN_POINT('',(23.3639873462086,-26.5442110315263,0.));
#18910=CARTESIAN_POINT('Origin',(17.6726647455408,-31.7899245798369,0.));
#18911=CARTESIAN_POINT('',(17.1867782189395,-30.9159026789286,0.));
#18912=CARTESIAN_POINT('',(18.5329974394853,-31.280191653953,0.));
#18913=CARTESIAN_POINT('Origin',(17.6726647455408,-31.7899245798369,0.));
#18914=CARTESIAN_POINT('',(18.5329974394853,-31.280191653953,15.));
#18915=CARTESIAN_POINT('',(18.5329974394853,-31.280191653953,0.));
#18916=CARTESIAN_POINT('',(17.1867782189395,-30.9159026789286,15.));
#18917=CARTESIAN_POINT('Origin',(17.6726647455408,-31.7899245798369,15.));
#18918=CARTESIAN_POINT('',(17.1867782189395,-30.9159026789286,0.));
#18919=CARTESIAN_POINT('Origin',(18.0251757251071,-30.4230847232658,0.));
#18920=CARTESIAN_POINT('',(19.1596907609891,-32.3379313568208,0.));
#18921=CARTESIAN_POINT('',(18.0251757251071,-30.4230847232658,0.));
#18922=CARTESIAN_POINT('',(19.1596907609891,-32.3379313568208,15.));
#18923=CARTESIAN_POINT('',(19.1596907609891,-32.3379313568208,0.));
#18924=CARTESIAN_POINT('',(18.0251757251071,-30.4230847232658,15.));
#18925=CARTESIAN_POINT('Origin',(15.3308575288479,-32.9831349545517,0.));
#18926=CARTESIAN_POINT('',(14.909355892181,-32.0763073136589,15.));
#18927=CARTESIAN_POINT('',(14.4127840596497,-33.3795452283267,15.));
#18928=CARTESIAN_POINT('Origin',(15.3308575288479,-32.9831349545517,15.));
#18929=CARTESIAN_POINT('',(14.4127840596497,-33.3795452283267,0.));
#18930=CARTESIAN_POINT('',(14.4127840596497,-33.3795452283267,0.));
#18931=CARTESIAN_POINT('',(14.909355892181,-32.0763073136589,0.));
#18932=CARTESIAN_POINT('Origin',(15.3308575288479,-32.9831349545517,0.));
#18933=CARTESIAN_POINT('',(14.909355892181,-32.0763073136589,0.));
#18934=CARTESIAN_POINT('Origin',(14.9001523628048,-34.5082745737944,0.));
#18935=CARTESIAN_POINT('',(14.9001523628048,-34.5082745737944,15.));
#18936=CARTESIAN_POINT('',(14.0178601012327,-32.4649140177865,15.));
#18937=CARTESIAN_POINT('',(14.9001523628048,-34.5082745737944,0.));
#18938=CARTESIAN_POINT('',(14.9001523628048,-34.5082745737944,0.));
#18939=CARTESIAN_POINT('',(14.0178601012327,-32.4649140177865,0.));
#18940=CARTESIAN_POINT('Origin',(6.98407602147874,-35.6951686664485,0.));
#18941=CARTESIAN_POINT('',(6.79205809501116,-34.7137772481474,0.));
#18942=CARTESIAN_POINT('',(7.95981717292703,-35.4762412689616,0.));
#18943=CARTESIAN_POINT('Origin',(6.98407602147874,-35.6951686664485,0.));
#18944=CARTESIAN_POINT('',(7.95981717292703,-35.4762412689616,15.));
#18945=CARTESIAN_POINT('',(7.95981717292703,-35.4762412689616,0.));
#18946=CARTESIAN_POINT('',(6.79205809501116,-34.7137772481474,15.));
#18947=CARTESIAN_POINT('Origin',(6.98407602147874,-35.6951686664485,15.));
#18948=CARTESIAN_POINT('',(6.79205809501116,-34.7137772481474,0.));
#18949=CARTESIAN_POINT('Origin',(7.74171062993031,-34.5041585975144,0.));
#18950=CARTESIAN_POINT('',(8.2289783962506,-36.6758703925241,0.));
#18951=CARTESIAN_POINT('',(7.74171062993031,-34.5041585975144,0.));
#18952=CARTESIAN_POINT('',(8.2289783962506,-36.6758703925241,15.));
#18953=CARTESIAN_POINT('',(8.2289783962506,-36.6758703925241,0.));
#18954=CARTESIAN_POINT('',(7.74171062993031,-34.5041585975144,15.));
#18955=CARTESIAN_POINT('Origin',(4.3881627244846,-36.1063209411239,0.));
#18956=CARTESIAN_POINT('',(4.2675159983083,-35.1136254352094,15.));
#18957=CARTESIAN_POINT('',(3.39252545782465,-36.199629211057,15.));
#18958=CARTESIAN_POINT('Origin',(4.3881627244846,-36.1063209411239,15.));
#18959=CARTESIAN_POINT('',(3.39252545782465,-36.199629211057,0.));
#18960=CARTESIAN_POINT('',(3.39252545782466,-36.199629211057,0.));
#18961=CARTESIAN_POINT('',(4.2675159983083,-35.1136254352094,0.));
#18962=CARTESIAN_POINT('Origin',(4.3881627244846,-36.1063209411239,0.));
#18963=CARTESIAN_POINT('',(4.2675159983083,-35.1136254352094,0.));
#18964=CARTESIAN_POINT('Origin',(3.50724370857672,-37.4237196983922,0.));
#18965=CARTESIAN_POINT('',(3.50724370857672,-37.4237196983922,15.));
#18966=CARTESIAN_POINT('',(3.29956704137369,-35.2077250236291,15.));
#18967=CARTESIAN_POINT('',(3.50724370857672,-37.4237196983922,0.));
#18968=CARTESIAN_POINT('',(3.50724370857672,-37.4237196983922,0.));
#18969=CARTESIAN_POINT('',(3.29956704137369,-35.2077250236291,0.));
#18970=CARTESIAN_POINT('Origin',(-4.38816272448462,-36.1063209411239,0.));
#18971=CARTESIAN_POINT('',(-4.26751599830832,-35.1136254352094,0.));
#18972=CARTESIAN_POINT('',(-3.39252545782467,-36.199629211057,0.));
#18973=CARTESIAN_POINT('Origin',(-4.38816272448462,-36.1063209411239,0.));
#18974=CARTESIAN_POINT('',(-3.39252545782467,-36.199629211057,15.));
#18975=CARTESIAN_POINT('',(-3.39252545782467,-36.199629211057,0.));
#18976=CARTESIAN_POINT('',(-4.26751599830832,-35.1136254352094,15.));
#18977=CARTESIAN_POINT('Origin',(-4.38816272448462,-36.1063209411239,15.));
#18978=CARTESIAN_POINT('',(-4.26751599830831,-35.1136254352094,0.));
#18979=CARTESIAN_POINT('Origin',(-3.29956704137371,-35.2077250236291,0.));
#18980=CARTESIAN_POINT('',(-3.50724370857673,-37.4237196983922,0.));
#18981=CARTESIAN_POINT('',(-3.29956704137371,-35.2077250236291,0.));
#18982=CARTESIAN_POINT('',(-3.50724370857673,-37.4237196983922,15.));
#18983=CARTESIAN_POINT('',(-3.50724370857673,-37.4237196983922,0.));
#18984=CARTESIAN_POINT('',(-3.29956704137371,-35.2077250236291,15.));
#18985=CARTESIAN_POINT('Origin',(-6.98407602147876,-35.6951686664485,0.));
#18986=CARTESIAN_POINT('',(-6.79205809501118,-34.7137772481474,15.));
#18987=CARTESIAN_POINT('',(-7.95981717292705,-35.4762412689616,15.));
#18988=CARTESIAN_POINT('Origin',(-6.98407602147876,-35.6951686664485,15.));
#18989=CARTESIAN_POINT('',(-7.95981717292705,-35.4762412689616,0.));
#18990=CARTESIAN_POINT('',(-7.95981717292705,-35.4762412689616,0.));
#18991=CARTESIAN_POINT('',(-6.79205809501118,-34.7137772481474,0.));
#18992=CARTESIAN_POINT('Origin',(-6.98407602147876,-35.6951686664485,0.));
#18993=CARTESIAN_POINT('',(-6.79205809501118,-34.7137772481474,0.));
#18994=CARTESIAN_POINT('Origin',(-8.22897839625062,-36.6758703925241,0.));
#18995=CARTESIAN_POINT('',(-8.22897839625062,-36.6758703925241,15.));
#18996=CARTESIAN_POINT('',(-7.74171062993033,-34.5041585975144,15.));
#18997=CARTESIAN_POINT('',(-8.22897839625062,-36.6758703925241,0.));
#18998=CARTESIAN_POINT('',(-8.22897839625062,-36.6758703925241,0.));
#18999=CARTESIAN_POINT('',(-7.74171062993033,-34.5041585975144,0.));
#19000=CARTESIAN_POINT('Origin',(-15.3308575288479,-32.9831349545516,0.));
#19001=CARTESIAN_POINT('',(-14.909355892181,-32.0763073136589,0.));
#19002=CARTESIAN_POINT('',(-14.4127840596497,-33.3795452283267,0.));
#19003=CARTESIAN_POINT('Origin',(-15.3308575288479,-32.9831349545516,0.));
#19004=CARTESIAN_POINT('',(-14.4127840596497,-33.3795452283267,15.));
#19005=CARTESIAN_POINT('',(-14.4127840596497,-33.3795452283267,0.));
#19006=CARTESIAN_POINT('',(-14.909355892181,-32.0763073136589,15.));
#19007=CARTESIAN_POINT('Origin',(-15.3308575288479,-32.9831349545516,15.));
#19008=CARTESIAN_POINT('',(-14.909355892181,-32.0763073136589,0.));
#19009=CARTESIAN_POINT('Origin',(-14.0178601012327,-32.4649140177865,0.));
#19010=CARTESIAN_POINT('',(-14.9001523628048,-34.5082745737944,0.));
#19011=CARTESIAN_POINT('',(-14.0178601012327,-32.4649140177865,0.));
#19012=CARTESIAN_POINT('',(-14.9001523628048,-34.5082745737944,15.));
#19013=CARTESIAN_POINT('',(-14.9001523628048,-34.5082745737944,0.));
#19014=CARTESIAN_POINT('',(-14.0178601012327,-32.4649140177865,15.));
#19015=CARTESIAN_POINT('Origin',(-17.6726647455408,-31.7899245798369,0.));
#19016=CARTESIAN_POINT('',(-17.1867782189396,-30.9159026789286,15.));
#19017=CARTESIAN_POINT('',(-18.5329974394853,-31.280191653953,15.));
#19018=CARTESIAN_POINT('Origin',(-17.6726647455408,-31.7899245798369,15.));
#19019=CARTESIAN_POINT('',(-18.5329974394853,-31.280191653953,0.));
#19020=CARTESIAN_POINT('',(-18.5329974394853,-31.280191653953,0.));
#19021=CARTESIAN_POINT('',(-17.1867782189396,-30.9159026789286,0.));
#19022=CARTESIAN_POINT('Origin',(-17.6726647455408,-31.7899245798369,0.));
#19023=CARTESIAN_POINT('',(-17.1867782189396,-30.9159026789286,0.));
#19024=CARTESIAN_POINT('Origin',(-19.1596907609891,-32.3379313568208,0.));
#19025=CARTESIAN_POINT('',(-19.1596907609891,-32.3379313568208,15.));
#19026=CARTESIAN_POINT('',(-18.0251757251071,-30.4230847232658,15.));
#19027=CARTESIAN_POINT('',(-19.1596907609891,-32.3379313568208,0.));
#19028=CARTESIAN_POINT('',(-19.1596907609891,-32.3379313568208,0.));
#19029=CARTESIAN_POINT('',(-18.0251757251071,-30.4230847232658,0.));
#19030=CARTESIAN_POINT('Origin',(-24.7728611819223,-26.6313299116137,0.));
#19031=CARTESIAN_POINT('',(-24.0917641517363,-25.899136743473,0.));
#19032=CARTESIAN_POINT('',(-24.0222189379449,-27.2920387896808,0.));
#19033=CARTESIAN_POINT('Origin',(-24.7728611819223,-26.6313299116137,0.));
#19034=CARTESIAN_POINT('',(-24.0222189379449,-27.2920387896808,15.));
#19035=CARTESIAN_POINT('',(-24.0222189379449,-27.2920387896808,0.));
#19036=CARTESIAN_POINT('',(-24.0917641517363,-25.899136743473,15.));
#19037=CARTESIAN_POINT('Origin',(-24.7728611819223,-26.6313299116137,15.));
#19038=CARTESIAN_POINT('',(-24.0917641517363,-25.899136743473,0.));
#19039=CARTESIAN_POINT('Origin',(-23.3639873462087,-26.5442110315263,0.));
#19040=CARTESIAN_POINT('',(-24.8345302882955,-28.2149191006268,0.));
#19041=CARTESIAN_POINT('',(-23.3639873462087,-26.5442110315263,0.));
#19042=CARTESIAN_POINT('',(-24.8345302882955,-28.2149191006268,15.));
#19043=CARTESIAN_POINT('',(-24.8345302882955,-28.2149191006268,0.));
#19044=CARTESIAN_POINT('',(-23.3639873462087,-26.5442110315263,15.));
#19045=CARTESIAN_POINT('Origin',(-26.6313299116137,-24.7728611819222,0.));
#19046=CARTESIAN_POINT('',(-25.899136743473,-24.0917641517363,15.));
#19047=CARTESIAN_POINT('',(-27.2920387896808,-24.0222189379449,15.));
#19048=CARTESIAN_POINT('Origin',(-26.6313299116137,-24.7728611819222,15.));
#19049=CARTESIAN_POINT('',(-27.2920387896808,-24.0222189379449,0.));
#19050=CARTESIAN_POINT('',(-27.2920387896808,-24.0222189379449,0.));
#19051=CARTESIAN_POINT('',(-25.899136743473,-24.0917641517363,0.));
#19052=CARTESIAN_POINT('Origin',(-26.6313299116137,-24.7728611819222,0.));
#19053=CARTESIAN_POINT('',(-25.899136743473,-24.0917641517363,0.));
#19054=CARTESIAN_POINT('Origin',(-28.2149191006269,-24.8345302882955,0.));
#19055=CARTESIAN_POINT('',(-28.2149191006269,-24.8345302882955,15.));
#19056=CARTESIAN_POINT('',(-26.5442110315263,-23.3639873462087,15.));
#19057=CARTESIAN_POINT('',(-28.2149191006269,-24.8345302882955,0.));
#19058=CARTESIAN_POINT('',(-28.2149191006269,-24.8345302882955,0.));
#19059=CARTESIAN_POINT('',(-26.5442110315263,-23.3639873462087,0.));
#19060=CARTESIAN_POINT('Origin',(-31.7899245798369,-17.6726647455408,0.));
#19061=CARTESIAN_POINT('',(-30.9159026789286,-17.1867782189396,0.));
#19062=CARTESIAN_POINT('',(-31.280191653953,-18.5329974394853,0.));
#19063=CARTESIAN_POINT('Origin',(-31.7899245798369,-17.6726647455408,0.));
#19064=CARTESIAN_POINT('',(-31.280191653953,-18.5329974394853,15.));
#19065=CARTESIAN_POINT('',(-31.280191653953,-18.5329974394853,0.));
#19066=CARTESIAN_POINT('',(-30.9159026789286,-17.1867782189396,15.));
#19067=CARTESIAN_POINT('Origin',(-31.7899245798369,-17.6726647455408,15.));
#19068=CARTESIAN_POINT('',(-30.9159026789286,-17.1867782189396,0.));
#19069=CARTESIAN_POINT('Origin',(-30.4230847232658,-18.0251757251071,0.));
#19070=CARTESIAN_POINT('',(-32.3379313568208,-19.1596907609891,0.));
#19071=CARTESIAN_POINT('',(-30.4230847232658,-18.0251757251071,0.));
#19072=CARTESIAN_POINT('',(-32.3379313568208,-19.1596907609891,15.));
#19073=CARTESIAN_POINT('',(-32.3379313568208,-19.1596907609891,0.));
#19074=CARTESIAN_POINT('',(-30.4230847232658,-18.0251757251071,15.));
#19075=CARTESIAN_POINT('Origin',(-32.9831349545517,-15.3308575288479,0.));
#19076=CARTESIAN_POINT('',(-32.0763073136589,-14.909355892181,15.));
#19077=CARTESIAN_POINT('',(-33.3795452283267,-14.4127840596497,15.));
#19078=CARTESIAN_POINT('Origin',(-32.9831349545517,-15.3308575288479,15.));
#19079=CARTESIAN_POINT('',(-33.3795452283267,-14.4127840596497,0.));
#19080=CARTESIAN_POINT('',(-33.3795452283267,-14.4127840596497,0.));
#19081=CARTESIAN_POINT('',(-32.0763073136589,-14.909355892181,0.));
#19082=CARTESIAN_POINT('Origin',(-32.9831349545517,-15.3308575288479,0.));
#19083=CARTESIAN_POINT('',(-32.0763073136589,-14.909355892181,0.));
#19084=CARTESIAN_POINT('Origin',(-34.5082745737944,-14.9001523628048,0.));
#19085=CARTESIAN_POINT('',(-34.5082745737944,-14.9001523628048,15.));
#19086=CARTESIAN_POINT('',(-32.4649140177865,-14.0178601012327,15.));
#19087=CARTESIAN_POINT('',(-34.5082745737944,-14.9001523628048,0.));
#19088=CARTESIAN_POINT('',(-34.5082745737944,-14.9001523628048,0.));
#19089=CARTESIAN_POINT('',(-32.4649140177865,-14.0178601012327,0.));
#19090=CARTESIAN_POINT('Origin',(-35.6951686664485,-6.98407602147875,0.));
#19091=CARTESIAN_POINT('',(-34.7137772481474,-6.79205809501117,0.));
#19092=CARTESIAN_POINT('',(-35.4762412689616,-7.95981717292703,0.));
#19093=CARTESIAN_POINT('Origin',(-35.6951686664485,-6.98407602147875,0.));
#19094=CARTESIAN_POINT('',(-35.4762412689616,-7.95981717292703,15.));
#19095=CARTESIAN_POINT('',(-35.4762412689616,-7.95981717292703,0.));
#19096=CARTESIAN_POINT('',(-34.7137772481474,-6.79205809501117,15.));
#19097=CARTESIAN_POINT('Origin',(-35.6951686664485,-6.98407602147875,15.));
#19098=CARTESIAN_POINT('',(-34.7137772481474,-6.79205809501117,0.));
#19099=CARTESIAN_POINT('Origin',(-34.5041585975144,-7.74171062993032,0.));
#19100=CARTESIAN_POINT('',(-36.6758703925241,-8.2289783962506,0.));
#19101=CARTESIAN_POINT('',(-34.5041585975144,-7.74171062993032,0.));
#19102=CARTESIAN_POINT('',(-36.6758703925241,-8.2289783962506,15.));
#19103=CARTESIAN_POINT('',(-36.6758703925241,-8.2289783962506,0.));
#19104=CARTESIAN_POINT('',(-34.5041585975144,-7.74171062993032,15.));
#19105=CARTESIAN_POINT('Origin',(-36.1063209411239,-4.3881627244846,0.));
#19106=CARTESIAN_POINT('',(-35.1136254352094,-4.2675159983083,15.));
#19107=CARTESIAN_POINT('',(-36.199629211057,-3.39252545782466,15.));
#19108=CARTESIAN_POINT('Origin',(-36.1063209411239,-4.3881627244846,15.));
#19109=CARTESIAN_POINT('',(-36.199629211057,-3.39252545782466,0.));
#19110=CARTESIAN_POINT('',(-36.199629211057,-3.39252545782466,0.));
#19111=CARTESIAN_POINT('',(-35.1136254352094,-4.2675159983083,0.));
#19112=CARTESIAN_POINT('Origin',(-36.1063209411239,-4.3881627244846,0.));
#19113=CARTESIAN_POINT('',(-35.1136254352094,-4.2675159983083,0.));
#19114=CARTESIAN_POINT('Origin',(-37.4237196983922,-3.50724370857673,0.));
#19115=CARTESIAN_POINT('',(-37.4237196983922,-3.50724370857673,15.));
#19116=CARTESIAN_POINT('',(-35.2077250236291,-3.29956704137369,15.));
#19117=CARTESIAN_POINT('',(-37.4237196983922,-3.50724370857673,0.));
#19118=CARTESIAN_POINT('',(-37.4237196983922,-3.50724370857673,0.));
#19119=CARTESIAN_POINT('',(-35.2077250236291,-3.29956704137369,0.));
#19120=CARTESIAN_POINT('Origin',(-36.1063209411239,4.38816272448462,0.));
#19121=CARTESIAN_POINT('',(-35.1136254352094,4.26751599830831,0.));
#19122=CARTESIAN_POINT('',(-36.199629211057,3.39252545782467,0.));
#19123=CARTESIAN_POINT('Origin',(-36.1063209411239,4.38816272448462,0.));
#19124=CARTESIAN_POINT('',(-36.199629211057,3.39252545782467,15.));
#19125=CARTESIAN_POINT('',(-36.199629211057,3.39252545782467,0.));
#19126=CARTESIAN_POINT('',(-35.1136254352094,4.26751599830831,15.));
#19127=CARTESIAN_POINT('Origin',(-36.1063209411239,4.38816272448462,15.));
#19128=CARTESIAN_POINT('',(-35.1136254352094,4.26751599830831,0.));
#19129=CARTESIAN_POINT('Origin',(-35.2077250236291,3.29956704137371,0.));
#19130=CARTESIAN_POINT('',(-37.4237196983923,3.50724370857673,0.));
#19131=CARTESIAN_POINT('',(-35.2077250236291,3.29956704137371,0.));
#19132=CARTESIAN_POINT('',(-37.4237196983923,3.50724370857673,15.));
#19133=CARTESIAN_POINT('',(-37.4237196983923,3.50724370857673,0.));
#19134=CARTESIAN_POINT('',(-35.2077250236291,3.29956704137371,15.));
#19135=CARTESIAN_POINT('Origin',(-35.6951686664485,6.98407602147875,0.));
#19136=CARTESIAN_POINT('',(-34.7137772481474,6.79205809501117,15.));
#19137=CARTESIAN_POINT('',(-35.4762412689616,7.95981717292704,15.));
#19138=CARTESIAN_POINT('Origin',(-35.6951686664485,6.98407602147875,15.));
#19139=CARTESIAN_POINT('',(-35.4762412689616,7.95981717292704,0.));
#19140=CARTESIAN_POINT('',(-35.4762412689616,7.95981717292705,0.));
#19141=CARTESIAN_POINT('',(-34.7137772481474,6.79205809501117,0.));
#19142=CARTESIAN_POINT('Origin',(-35.6951686664485,6.98407602147875,0.));
#19143=CARTESIAN_POINT('',(-34.7137772481474,6.79205809501117,0.));
#19144=CARTESIAN_POINT('Origin',(-36.6758703925241,8.22897839625061,0.));
#19145=CARTESIAN_POINT('',(-36.6758703925241,8.22897839625061,15.));
#19146=CARTESIAN_POINT('',(-34.5041585975144,7.74171062993032,15.));
#19147=CARTESIAN_POINT('',(-36.6758703925241,8.22897839625061,0.));
#19148=CARTESIAN_POINT('',(-36.6758703925241,8.22897839625061,0.));
#19149=CARTESIAN_POINT('',(-34.5041585975144,7.74171062993032,0.));
#19150=CARTESIAN_POINT('Origin',(-32.9831349545516,15.3308575288479,0.));
#19151=CARTESIAN_POINT('',(-32.0763073136589,14.909355892181,0.));
#19152=CARTESIAN_POINT('',(-33.3795452283267,14.4127840596497,0.));
#19153=CARTESIAN_POINT('Origin',(-32.9831349545516,15.3308575288479,0.));
#19154=CARTESIAN_POINT('',(-33.3795452283267,14.4127840596497,15.));
#19155=CARTESIAN_POINT('',(-33.3795452283267,14.4127840596497,0.));
#19156=CARTESIAN_POINT('',(-32.0763073136589,14.909355892181,15.));
#19157=CARTESIAN_POINT('Origin',(-32.9831349545516,15.3308575288479,15.));
#19158=CARTESIAN_POINT('',(-32.0763073136589,14.909355892181,0.));
#19159=CARTESIAN_POINT('Origin',(-32.4649140177865,14.0178601012327,0.));
#19160=CARTESIAN_POINT('',(-34.5082745737944,14.9001523628048,0.));
#19161=CARTESIAN_POINT('',(-32.4649140177865,14.0178601012327,0.));
#19162=CARTESIAN_POINT('',(-34.5082745737944,14.9001523628048,15.));
#19163=CARTESIAN_POINT('',(-34.5082745737944,14.9001523628048,0.));
#19164=CARTESIAN_POINT('',(-32.4649140177865,14.0178601012327,15.));
#19165=CARTESIAN_POINT('Origin',(-31.7899245798369,17.6726647455408,0.));
#19166=CARTESIAN_POINT('',(-30.9159026789286,17.1867782189396,15.));
#19167=CARTESIAN_POINT('',(-31.280191653953,18.5329974394853,15.));
#19168=CARTESIAN_POINT('Origin',(-31.7899245798369,17.6726647455408,15.));
#19169=CARTESIAN_POINT('',(-31.280191653953,18.5329974394853,0.));
#19170=CARTESIAN_POINT('',(-31.280191653953,18.5329974394853,0.));
#19171=CARTESIAN_POINT('',(-30.9159026789286,17.1867782189396,0.));
#19172=CARTESIAN_POINT('Origin',(-31.7899245798369,17.6726647455408,0.));
#19173=CARTESIAN_POINT('',(-30.9159026789286,17.1867782189396,0.));
#19174=CARTESIAN_POINT('Origin',(-32.3379313568208,19.1596907609891,0.));
#19175=CARTESIAN_POINT('',(-32.3379313568208,19.1596907609891,15.));
#19176=CARTESIAN_POINT('',(-30.4230847232658,18.0251757251071,15.));
#19177=CARTESIAN_POINT('',(-32.3379313568208,19.1596907609891,0.));
#19178=CARTESIAN_POINT('',(-32.3379313568208,19.1596907609891,0.));
#19179=CARTESIAN_POINT('',(-30.4230847232658,18.0251757251071,0.));
#19180=CARTESIAN_POINT('Origin',(-26.6313299116137,24.7728611819222,0.));
#19181=CARTESIAN_POINT('',(-25.899136743473,24.0917641517363,0.));
#19182=CARTESIAN_POINT('',(-27.2920387896808,24.0222189379449,0.));
#19183=CARTESIAN_POINT('Origin',(-26.6313299116137,24.7728611819222,0.));
#19184=CARTESIAN_POINT('',(-27.2920387896808,24.0222189379449,15.));
#19185=CARTESIAN_POINT('',(-27.2920387896808,24.0222189379449,0.));
#19186=CARTESIAN_POINT('',(-25.899136743473,24.0917641517363,15.));
#19187=CARTESIAN_POINT('Origin',(-26.6313299116137,24.7728611819222,15.));
#19188=CARTESIAN_POINT('',(-25.899136743473,24.0917641517363,0.));
#19189=CARTESIAN_POINT('Origin',(-26.5442110315263,23.3639873462087,0.));
#19190=CARTESIAN_POINT('',(-28.2149191006268,24.8345302882955,0.));
#19191=CARTESIAN_POINT('',(-26.5442110315263,23.3639873462087,0.));
#19192=CARTESIAN_POINT('',(-28.2149191006268,24.8345302882955,15.));
#19193=CARTESIAN_POINT('',(-28.2149191006268,24.8345302882955,0.));
#19194=CARTESIAN_POINT('',(-26.5442110315263,23.3639873462087,15.));
#19195=CARTESIAN_POINT('Origin',(-24.7728611819223,26.6313299116137,0.));
#19196=CARTESIAN_POINT('',(-24.0917641517363,25.899136743473,15.));
#19197=CARTESIAN_POINT('',(-24.0222189379449,27.2920387896808,15.));
#19198=CARTESIAN_POINT('Origin',(-24.7728611819223,26.6313299116137,15.));
#19199=CARTESIAN_POINT('',(-24.0222189379449,27.2920387896808,0.));
#19200=CARTESIAN_POINT('',(-24.0222189379449,27.2920387896808,0.));
#19201=CARTESIAN_POINT('',(-24.0917641517363,25.899136743473,0.));
#19202=CARTESIAN_POINT('Origin',(-24.7728611819223,26.6313299116137,0.));
#19203=CARTESIAN_POINT('',(-24.0917641517363,25.899136743473,0.));
#19204=CARTESIAN_POINT('Origin',(-24.8345302882955,28.2149191006269,0.));
#19205=CARTESIAN_POINT('',(-24.8345302882955,28.2149191006269,15.));
#19206=CARTESIAN_POINT('',(-23.3639873462087,26.5442110315263,15.));
#19207=CARTESIAN_POINT('',(-24.8345302882955,28.2149191006269,0.));
#19208=CARTESIAN_POINT('',(-24.8345302882955,28.2149191006269,0.));
#19209=CARTESIAN_POINT('',(-23.3639873462087,26.5442110315263,0.));
#19210=CARTESIAN_POINT('Origin',(-17.6726647455408,31.7899245798369,0.));
#19211=CARTESIAN_POINT('',(-17.1867782189395,30.9159026789286,0.));
#19212=CARTESIAN_POINT('',(-18.5329974394853,31.280191653953,0.));
#19213=CARTESIAN_POINT('Origin',(-17.6726647455408,31.7899245798369,0.));
#19214=CARTESIAN_POINT('',(-18.5329974394853,31.280191653953,15.));
#19215=CARTESIAN_POINT('',(-18.5329974394853,31.280191653953,0.));
#19216=CARTESIAN_POINT('',(-17.1867782189395,30.9159026789286,15.));
#19217=CARTESIAN_POINT('Origin',(-17.6726647455408,31.7899245798369,15.));
#19218=CARTESIAN_POINT('',(-17.1867782189395,30.9159026789286,0.));
#19219=CARTESIAN_POINT('Origin',(-18.0251757251071,30.4230847232658,0.));
#19220=CARTESIAN_POINT('',(-19.1596907609891,32.3379313568208,0.));
#19221=CARTESIAN_POINT('',(-18.0251757251071,30.4230847232658,0.));
#19222=CARTESIAN_POINT('',(-19.1596907609891,32.3379313568208,15.));
#19223=CARTESIAN_POINT('',(-19.1596907609891,32.3379313568208,0.));
#19224=CARTESIAN_POINT('',(-18.0251757251071,30.4230847232658,15.));
#19225=CARTESIAN_POINT('Origin',(-15.3308575288479,32.9831349545516,0.));
#19226=CARTESIAN_POINT('',(-14.909355892181,32.0763073136589,15.));
#19227=CARTESIAN_POINT('',(-14.4127840596497,33.3795452283267,15.));
#19228=CARTESIAN_POINT('Origin',(-15.3308575288479,32.9831349545516,15.));
#19229=CARTESIAN_POINT('',(-14.4127840596497,33.3795452283267,0.));
#19230=CARTESIAN_POINT('',(-14.4127840596497,33.3795452283267,0.));
#19231=CARTESIAN_POINT('',(-14.909355892181,32.0763073136589,0.));
#19232=CARTESIAN_POINT('Origin',(-15.3308575288479,32.9831349545516,0.));
#19233=CARTESIAN_POINT('',(-14.909355892181,32.0763073136589,0.));
#19234=CARTESIAN_POINT('Origin',(-14.9001523628048,34.5082745737944,0.));
#19235=CARTESIAN_POINT('',(-14.9001523628048,34.5082745737944,15.));
#19236=CARTESIAN_POINT('',(-14.0178601012327,32.4649140177865,15.));
#19237=CARTESIAN_POINT('',(-14.9001523628048,34.5082745737944,0.));
#19238=CARTESIAN_POINT('',(-14.9001523628048,34.5082745737944,0.));
#19239=CARTESIAN_POINT('',(-14.0178601012327,32.4649140177865,0.));
#19240=CARTESIAN_POINT('Origin',(-6.98407602147875,35.6951686664485,0.));
#19241=CARTESIAN_POINT('',(-6.79205809501117,34.7137772481474,0.));
#19242=CARTESIAN_POINT('',(-7.95981717292704,35.4762412689616,0.));
#19243=CARTESIAN_POINT('Origin',(-6.98407602147875,35.6951686664485,0.));
#19244=CARTESIAN_POINT('',(-7.95981717292704,35.4762412689616,15.));
#19245=CARTESIAN_POINT('',(-7.95981717292704,35.4762412689616,0.));
#19246=CARTESIAN_POINT('',(-6.79205809501117,34.7137772481474,15.));
#19247=CARTESIAN_POINT('Origin',(-6.98407602147875,35.6951686664485,15.));
#19248=CARTESIAN_POINT('',(-6.79205809501117,34.7137772481474,0.));
#19249=CARTESIAN_POINT('Origin',(-7.74171062993032,34.5041585975144,0.));
#19250=CARTESIAN_POINT('',(-8.22897839625061,36.6758703925241,0.));
#19251=CARTESIAN_POINT('',(-7.74171062993032,34.5041585975144,0.));
#19252=CARTESIAN_POINT('',(-8.22897839625061,36.6758703925241,15.));
#19253=CARTESIAN_POINT('',(-8.22897839625061,36.6758703925241,0.));
#19254=CARTESIAN_POINT('',(-7.74171062993032,34.5041585975144,15.));
#19255=CARTESIAN_POINT('Origin',(-4.38816272448461,36.1063209411239,0.));
#19256=CARTESIAN_POINT('',(-4.26751599830831,35.1136254352094,15.));
#19257=CARTESIAN_POINT('',(-3.39252545782466,36.199629211057,15.));
#19258=CARTESIAN_POINT('Origin',(-4.38816272448461,36.1063209411239,15.));
#19259=CARTESIAN_POINT('',(-3.39252545782466,36.199629211057,0.));
#19260=CARTESIAN_POINT('',(-3.39252545782466,36.199629211057,0.));
#19261=CARTESIAN_POINT('',(-4.26751599830831,35.1136254352094,0.));
#19262=CARTESIAN_POINT('Origin',(-4.38816272448461,36.1063209411239,0.));
#19263=CARTESIAN_POINT('',(-4.26751599830831,35.1136254352094,0.));
#19264=CARTESIAN_POINT('Origin',(-3.50724370857673,37.4237196983922,0.));
#19265=CARTESIAN_POINT('',(-3.50724370857673,37.4237196983922,15.));
#19266=CARTESIAN_POINT('',(-3.2995670413737,35.2077250236291,15.));
#19267=CARTESIAN_POINT('',(-3.50724370857673,37.4237196983922,0.));
#19268=CARTESIAN_POINT('',(-3.50724370857673,37.4237196983922,0.));
#19269=CARTESIAN_POINT('',(-3.2995670413737,35.2077250236291,0.));
#19270=CARTESIAN_POINT('Origin',(4.38816272448462,36.1063209411239,0.));
#19271=CARTESIAN_POINT('',(4.26751599830831,35.1136254352094,0.));
#19272=CARTESIAN_POINT('',(3.39252545782467,36.199629211057,0.));
#19273=CARTESIAN_POINT('Origin',(4.38816272448462,36.1063209411239,0.));
#19274=CARTESIAN_POINT('',(3.39252545782467,36.199629211057,15.));
#19275=CARTESIAN_POINT('',(3.39252545782467,36.199629211057,0.));
#19276=CARTESIAN_POINT('',(4.26751599830831,35.1136254352094,15.));
#19277=CARTESIAN_POINT('Origin',(4.38816272448462,36.1063209411239,15.));
#19278=CARTESIAN_POINT('',(4.26751599830831,35.1136254352094,0.));
#19279=CARTESIAN_POINT('Origin',(3.2995670413737,35.2077250236291,0.));
#19280=CARTESIAN_POINT('',(3.50724370857673,37.4237196983923,0.));
#19281=CARTESIAN_POINT('',(3.2995670413737,35.2077250236291,0.));
#19282=CARTESIAN_POINT('',(3.50724370857673,37.4237196983923,15.));
#19283=CARTESIAN_POINT('',(3.50724370857673,37.4237196983923,0.));
#19284=CARTESIAN_POINT('',(3.2995670413737,35.2077250236291,15.));
#19285=CARTESIAN_POINT('Origin',(6.98407602147876,35.6951686664485,0.));
#19286=CARTESIAN_POINT('',(6.79205809501118,34.7137772481474,15.));
#19287=CARTESIAN_POINT('',(7.95981717292704,35.4762412689616,15.));
#19288=CARTESIAN_POINT('Origin',(6.98407602147876,35.6951686664485,15.));
#19289=CARTESIAN_POINT('',(7.95981717292704,35.4762412689616,0.));
#19290=CARTESIAN_POINT('',(7.95981717292705,35.4762412689616,0.));
#19291=CARTESIAN_POINT('',(6.79205809501118,34.7137772481474,0.));
#19292=CARTESIAN_POINT('Origin',(6.98407602147876,35.6951686664485,0.));
#19293=CARTESIAN_POINT('',(6.79205809501118,34.7137772481474,0.));
#19294=CARTESIAN_POINT('Origin',(8.22897839625062,36.6758703925241,0.));
#19295=CARTESIAN_POINT('',(8.22897839625062,36.6758703925241,15.));
#19296=CARTESIAN_POINT('',(7.74171062993033,34.5041585975144,15.));
#19297=CARTESIAN_POINT('',(8.22897839625062,36.6758703925241,0.));
#19298=CARTESIAN_POINT('',(8.22897839625062,36.6758703925241,0.));
#19299=CARTESIAN_POINT('',(7.74171062993033,34.5041585975144,0.));
#19300=CARTESIAN_POINT('Origin',(15.3308575288479,32.9831349545517,0.));
#19301=CARTESIAN_POINT('',(14.909355892181,32.0763073136589,0.));
#19302=CARTESIAN_POINT('',(14.4127840596497,33.3795452283267,0.));
#19303=CARTESIAN_POINT('Origin',(15.3308575288479,32.9831349545517,0.));
#19304=CARTESIAN_POINT('',(14.4127840596497,33.3795452283267,15.));
#19305=CARTESIAN_POINT('',(14.4127840596497,33.3795452283267,0.));
#19306=CARTESIAN_POINT('',(14.909355892181,32.0763073136589,15.));
#19307=CARTESIAN_POINT('Origin',(15.3308575288479,32.9831349545517,15.));
#19308=CARTESIAN_POINT('',(14.909355892181,32.0763073136589,0.));
#19309=CARTESIAN_POINT('Origin',(14.0178601012327,32.4649140177865,0.));
#19310=CARTESIAN_POINT('',(14.9001523628048,34.5082745737944,0.));
#19311=CARTESIAN_POINT('',(14.0178601012327,32.4649140177865,0.));
#19312=CARTESIAN_POINT('',(14.9001523628048,34.5082745737944,15.));
#19313=CARTESIAN_POINT('',(14.9001523628048,34.5082745737944,0.));
#19314=CARTESIAN_POINT('',(14.0178601012327,32.4649140177865,15.));
#19315=CARTESIAN_POINT('Origin',(17.6726647455408,31.7899245798369,0.));
#19316=CARTESIAN_POINT('',(17.1867782189396,30.9159026789286,15.));
#19317=CARTESIAN_POINT('',(18.5329974394853,31.280191653953,15.));
#19318=CARTESIAN_POINT('Origin',(17.6726647455408,31.7899245798369,15.));
#19319=CARTESIAN_POINT('',(18.5329974394853,31.280191653953,0.));
#19320=CARTESIAN_POINT('',(18.5329974394853,31.280191653953,0.));
#19321=CARTESIAN_POINT('',(17.1867782189396,30.9159026789286,0.));
#19322=CARTESIAN_POINT('Origin',(17.6726647455408,31.7899245798369,0.));
#19323=CARTESIAN_POINT('',(17.1867782189396,30.9159026789286,0.));
#19324=CARTESIAN_POINT('Origin',(19.1596907609891,32.3379313568208,0.));
#19325=CARTESIAN_POINT('',(19.1596907609891,32.3379313568208,15.));
#19326=CARTESIAN_POINT('',(18.0251757251071,30.4230847232658,15.));
#19327=CARTESIAN_POINT('',(19.1596907609891,32.3379313568208,0.));
#19328=CARTESIAN_POINT('',(19.1596907609891,32.3379313568208,0.));
#19329=CARTESIAN_POINT('',(18.0251757251071,30.4230847232658,0.));
#19330=CARTESIAN_POINT('Origin',(24.7728611819223,26.6313299116137,0.));
#19331=CARTESIAN_POINT('',(24.0917641517363,25.899136743473,0.));
#19332=CARTESIAN_POINT('',(24.0222189379449,27.2920387896808,0.));
#19333=CARTESIAN_POINT('Origin',(24.7728611819223,26.6313299116137,0.));
#19334=CARTESIAN_POINT('',(24.0222189379449,27.2920387896808,15.));
#19335=CARTESIAN_POINT('',(24.0222189379449,27.2920387896808,0.));
#19336=CARTESIAN_POINT('',(24.0917641517363,25.899136743473,15.));
#19337=CARTESIAN_POINT('Origin',(24.7728611819223,26.6313299116137,15.));
#19338=CARTESIAN_POINT('',(24.0917641517363,25.899136743473,0.));
#19339=CARTESIAN_POINT('Origin',(23.3639873462087,26.5442110315263,0.));
#19340=CARTESIAN_POINT('',(24.8345302882955,28.2149191006268,0.));
#19341=CARTESIAN_POINT('',(23.3639873462087,26.5442110315263,0.));
#19342=CARTESIAN_POINT('',(24.8345302882955,28.2149191006268,15.));
#19343=CARTESIAN_POINT('',(24.8345302882955,28.2149191006268,0.));
#19344=CARTESIAN_POINT('',(23.3639873462087,26.5442110315263,15.));
#19345=CARTESIAN_POINT('Origin',(26.6313299116137,24.7728611819223,0.));
#19346=CARTESIAN_POINT('',(25.899136743473,24.0917641517363,15.));
#19347=CARTESIAN_POINT('',(27.2920387896808,24.0222189379449,15.));
#19348=CARTESIAN_POINT('Origin',(26.6313299116137,24.7728611819223,15.));
#19349=CARTESIAN_POINT('',(27.2920387896808,24.0222189379449,0.));
#19350=CARTESIAN_POINT('',(27.2920387896808,24.0222189379449,0.));
#19351=CARTESIAN_POINT('',(25.899136743473,24.0917641517363,0.));
#19352=CARTESIAN_POINT('Origin',(26.6313299116137,24.7728611819223,0.));
#19353=CARTESIAN_POINT('',(25.899136743473,24.0917641517363,0.));
#19354=CARTESIAN_POINT('Origin',(28.2149191006269,24.8345302882955,0.));
#19355=CARTESIAN_POINT('',(28.2149191006269,24.8345302882955,15.));
#19356=CARTESIAN_POINT('',(26.5442110315263,23.3639873462087,15.));
#19357=CARTESIAN_POINT('',(28.2149191006269,24.8345302882955,0.));
#19358=CARTESIAN_POINT('',(28.2149191006269,24.8345302882955,0.));
#19359=CARTESIAN_POINT('',(26.5442110315263,23.3639873462087,0.));
#19360=CARTESIAN_POINT('Origin',(31.7899245798369,17.6726647455408,0.));
#19361=CARTESIAN_POINT('',(30.9159026789286,17.1867782189396,0.));
#19362=CARTESIAN_POINT('',(31.280191653953,18.5329974394853,0.));
#19363=CARTESIAN_POINT('Origin',(31.7899245798369,17.6726647455408,0.));
#19364=CARTESIAN_POINT('',(31.280191653953,18.5329974394853,15.));
#19365=CARTESIAN_POINT('',(31.280191653953,18.5329974394853,0.));
#19366=CARTESIAN_POINT('',(30.9159026789286,17.1867782189396,15.));
#19367=CARTESIAN_POINT('Origin',(31.7899245798369,17.6726647455408,15.));
#19368=CARTESIAN_POINT('',(30.9159026789286,17.1867782189396,0.));
#19369=CARTESIAN_POINT('Origin',(30.4230847232658,18.0251757251071,0.));
#19370=CARTESIAN_POINT('',(32.3379313568208,19.1596907609891,0.));
#19371=CARTESIAN_POINT('',(30.4230847232658,18.0251757251071,0.));
#19372=CARTESIAN_POINT('',(32.3379313568208,19.1596907609891,15.));
#19373=CARTESIAN_POINT('',(32.3379313568208,19.1596907609891,0.));
#19374=CARTESIAN_POINT('',(30.4230847232658,18.0251757251071,15.));
#19375=CARTESIAN_POINT('Origin',(32.9831349545516,15.3308575288479,0.));
#19376=CARTESIAN_POINT('',(32.0763073136589,14.909355892181,15.));
#19377=CARTESIAN_POINT('',(33.3795452283267,14.4127840596497,15.));
#19378=CARTESIAN_POINT('Origin',(32.9831349545516,15.3308575288479,15.));
#19379=CARTESIAN_POINT('',(33.3795452283267,14.4127840596497,0.));
#19380=CARTESIAN_POINT('',(33.3795452283267,14.4127840596497,0.));
#19381=CARTESIAN_POINT('',(32.0763073136589,14.909355892181,0.));
#19382=CARTESIAN_POINT('Origin',(32.9831349545516,15.3308575288479,0.));
#19383=CARTESIAN_POINT('',(32.0763073136589,14.909355892181,0.));
#19384=CARTESIAN_POINT('Origin',(34.5082745737944,14.9001523628048,0.));
#19385=CARTESIAN_POINT('',(34.5082745737944,14.9001523628048,15.));
#19386=CARTESIAN_POINT('',(32.4649140177865,14.0178601012327,15.));
#19387=CARTESIAN_POINT('',(34.5082745737944,14.9001523628048,0.));
#19388=CARTESIAN_POINT('',(34.5082745737944,14.9001523628048,0.));
#19389=CARTESIAN_POINT('',(32.4649140177865,14.0178601012327,0.));
#19390=CARTESIAN_POINT('Origin',(35.6951686664485,6.98407602147875,0.));
#19391=CARTESIAN_POINT('',(34.7137772481474,6.79205809501117,0.));
#19392=CARTESIAN_POINT('',(35.4762412689616,7.95981717292704,0.));
#19393=CARTESIAN_POINT('Origin',(35.6951686664485,6.98407602147875,0.));
#19394=CARTESIAN_POINT('',(35.4762412689616,7.95981717292704,15.));
#19395=CARTESIAN_POINT('',(35.4762412689616,7.95981717292704,0.));
#19396=CARTESIAN_POINT('',(34.7137772481474,6.79205809501117,15.));
#19397=CARTESIAN_POINT('Origin',(35.6951686664485,6.98407602147875,15.));
#19398=CARTESIAN_POINT('',(34.7137772481474,6.79205809501117,0.));
#19399=CARTESIAN_POINT('Origin',(34.5041585975144,7.74171062993032,0.));
#19400=CARTESIAN_POINT('',(36.6758703925241,8.22897839625061,0.));
#19401=CARTESIAN_POINT('',(34.5041585975144,7.74171062993032,0.));
#19402=CARTESIAN_POINT('',(36.6758703925241,8.22897839625061,15.));
#19403=CARTESIAN_POINT('',(36.6758703925241,8.22897839625061,0.));
#19404=CARTESIAN_POINT('',(34.5041585975144,7.74171062993032,15.));
#19405=CARTESIAN_POINT('Ctrl Pts',(42.2550026135057,-12.2684454652018,0.));
#19406=CARTESIAN_POINT('Ctrl Pts',(42.2550026135057,-12.2684454652018,18.));
#19407=CARTESIAN_POINT('Ctrl Pts',(42.2409327400055,-12.2530833383985,0.));
#19408=CARTESIAN_POINT('Ctrl Pts',(42.2409327400055,-12.2530833383985,18.));
#19409=CARTESIAN_POINT('Ctrl Pts',(42.2127669677092,-12.222401466668,0.));
#19410=CARTESIAN_POINT('Ctrl Pts',(42.2127669677092,-12.222401466668,18.));
#19411=CARTESIAN_POINT('Ctrl Pts',(42.1704402333854,-12.1765058047069,0.));
#19412=CARTESIAN_POINT('Ctrl Pts',(42.1704402333854,-12.1765058047069,18.));
#19413=CARTESIAN_POINT('Ctrl Pts',(42.1138483839101,-12.1155659644537,0.));
#19414=CARTESIAN_POINT('Ctrl Pts',(42.1138483839101,-12.1155659644537,18.));
#19415=CARTESIAN_POINT('Ctrl Pts',(42.0428479428228,-12.0398158079102,0.));
#19416=CARTESIAN_POINT('Ctrl Pts',(42.0428479428228,-12.0398158079102,18.));
#19417=CARTESIAN_POINT('Ctrl Pts',(41.9715865222182,-11.9644914999263,0.));
#19418=CARTESIAN_POINT('Ctrl Pts',(41.9715865222182,-11.9644914999263,18.));
#19419=CARTESIAN_POINT('Ctrl Pts',(41.9000638152266,-11.8895948153349,0.));
#19420=CARTESIAN_POINT('Ctrl Pts',(41.9000638152266,-11.8895948153349,18.));
#19421=CARTESIAN_POINT('Ctrl Pts',(41.8282796562569,-11.81512813804,0.));
#19422=CARTESIAN_POINT('Ctrl Pts',(41.8282796562569,-11.81512813804,18.));
#19423=CARTESIAN_POINT('Ctrl Pts',(41.7562341395977,-11.7410945211992,0.));
#19424=CARTESIAN_POINT('Ctrl Pts',(41.7562341395977,-11.7410945211992,18.));
#19425=CARTESIAN_POINT('Ctrl Pts',(41.6839275596248,-11.6674975352852,0.));
#19426=CARTESIAN_POINT('Ctrl Pts',(41.6839275596248,-11.6674975352852,18.));
#19427=CARTESIAN_POINT('Ctrl Pts',(41.6113603270596,-11.5943410868252,0.));
#19428=CARTESIAN_POINT('Ctrl Pts',(41.6113603270596,-11.5943410868252,18.));
#19429=CARTESIAN_POINT('Ctrl Pts',(41.5385328935506,-11.5216292382388,0.));
#19430=CARTESIAN_POINT('Ctrl Pts',(41.5385328935506,-11.5216292382388,18.));
#19431=CARTESIAN_POINT('Ctrl Pts',(41.4654456796071,-11.449366039385,0.));
#19432=CARTESIAN_POINT('Ctrl Pts',(41.4654456796071,-11.449366039385,18.));
#19433=CARTESIAN_POINT('Ctrl Pts',(41.3920989905986,-11.3775553120177,0.));
#19434=CARTESIAN_POINT('Ctrl Pts',(41.3920989905986,-11.3775553120177,18.));
#19435=CARTESIAN_POINT('Ctrl Pts',(41.3184930194148,-11.3062006993745,0.));
#19436=CARTESIAN_POINT('Ctrl Pts',(41.3184930194148,-11.3062006993745,18.));
#19437=CARTESIAN_POINT('Ctrl Pts',(41.2446278781981,-11.2353057980338,0.));
#19438=CARTESIAN_POINT('Ctrl Pts',(41.2446278781981,-11.2353057980338,18.));
#19439=CARTESIAN_POINT('Ctrl Pts',(41.1705036228854,-11.1648742640378,0.));
#19440=CARTESIAN_POINT('Ctrl Pts',(41.1705036228854,-11.1648742640378,18.));
#19441=CARTESIAN_POINT('Ctrl Pts',(41.0961202807715,-11.0949099155251,0.));
#19442=CARTESIAN_POINT('Ctrl Pts',(41.0961202807715,-11.0949099155251,18.));
#19443=CARTESIAN_POINT('Ctrl Pts',(41.0214778832142,-11.0254168609972,0.));
#19444=CARTESIAN_POINT('Ctrl Pts',(41.0214778832142,-11.0254168609972,18.));
#19445=CARTESIAN_POINT('Ctrl Pts',(40.9465764747798,-10.956399476781,0.));
#19446=CARTESIAN_POINT('Ctrl Pts',(40.9465764747798,-10.956399476781,18.));
#19447=CARTESIAN_POINT('Ctrl Pts',(40.8714161092412,-10.8878623066647,0.));
#19448=CARTESIAN_POINT('Ctrl Pts',(40.8714161092412,-10.8878623066647,18.));
#19449=CARTESIAN_POINT('Ctrl Pts',(40.7959968527561,-10.8198099757795,0.));
#19450=CARTESIAN_POINT('Ctrl Pts',(40.7959968527561,-10.8198099757795,18.));
#19451=CARTESIAN_POINT('Ctrl Pts',(40.7203187831783,-10.7522471109694,0.));
#19452=CARTESIAN_POINT('Ctrl Pts',(40.7203187831783,-10.7522471109694,18.));
#19453=CARTESIAN_POINT('Ctrl Pts',(40.6443819999244,-10.6851782157325,0.));
#19454=CARTESIAN_POINT('Ctrl Pts',(40.6443819999244,-10.6851782157325,18.));
#19455=CARTESIAN_POINT('Ctrl Pts',(40.5681866012103,-10.618607730849,0.));
#19456=CARTESIAN_POINT('Ctrl Pts',(40.5681866012103,-10.618607730849,18.));
#19457=CARTESIAN_POINT('Ctrl Pts',(40.4917326404439,-10.5525402237951,0.));
#19458=CARTESIAN_POINT('Ctrl Pts',(40.4917326404439,-10.5525402237951,18.));
#19459=CARTESIAN_POINT('Ctrl Pts',(40.4150200869536,-10.48698054978,0.));
#19460=CARTESIAN_POINT('Ctrl Pts',(40.4150200869536,-10.48698054978,18.));
#19461=CARTESIAN_POINT('Ctrl Pts',(40.3380487942952,-10.4219339932951,0.));
#19462=CARTESIAN_POINT('Ctrl Pts',(40.3380487942952,-10.4219339932951,18.));
#19463=CARTESIAN_POINT('Ctrl Pts',(40.2608184485326,-10.3574064830678,0.));
#19464=CARTESIAN_POINT('Ctrl Pts',(40.2608184485326,-10.3574064830678,18.));
#19465=CARTESIAN_POINT('Ctrl Pts',(40.1833286010098,-10.2934044990237,0.));
#19466=CARTESIAN_POINT('Ctrl Pts',(40.1833286010098,-10.2934044990237,18.));
#19467=CARTESIAN_POINT('Ctrl Pts',(40.1055787732578,-10.2299347125857,0.));
#19468=CARTESIAN_POINT('Ctrl Pts',(40.1055787732578,-10.2299347125857,18.));
#19469=CARTESIAN_POINT('Ctrl Pts',(40.0275685525923,-10.1670036683795,0.));
#19470=CARTESIAN_POINT('Ctrl Pts',(40.0275685525923,-10.1670036683795,18.));
#19471=CARTESIAN_POINT('Ctrl Pts',(39.9492976736738,-10.1046175096878,0.));
#19472=CARTESIAN_POINT('Ctrl Pts',(39.9492976736738,-10.1046175096878,18.));
#19473=CARTESIAN_POINT('Ctrl Pts',(39.8707661565233,-10.0427815229883,0.));
#19474=CARTESIAN_POINT('Ctrl Pts',(39.8707661565233,-10.0427815229883,18.));
#19475=CARTESIAN_POINT('Ctrl Pts',(39.7919742367922,-9.98150036150824,0.));
#19476=CARTESIAN_POINT('Ctrl Pts',(39.7919742367922,-9.98150036150824,18.));
#19477=CARTESIAN_POINT('Ctrl Pts',(39.712922089547,-9.92077894513193,0.));
#19478=CARTESIAN_POINT('Ctrl Pts',(39.712922089547,-9.92077894513193,18.));
#19479=CARTESIAN_POINT('Ctrl Pts',(39.6336095893767,-9.86062324242561,0.));
#19480=CARTESIAN_POINT('Ctrl Pts',(39.6336095893767,-9.86062324242561,18.));
#19481=CARTESIAN_POINT('Ctrl Pts',(39.5540361022309,-9.80104095251614,0.));
#19482=CARTESIAN_POINT('Ctrl Pts',(39.5540361022309,-9.80104095251614,18.));
#19483=CARTESIAN_POINT('Ctrl Pts',(39.4742001555227,-9.74204258152664,0.));
#19484=CARTESIAN_POINT('Ctrl Pts',(39.4742001555227,-9.74204258152664,18.));
#19485=CARTESIAN_POINT('Ctrl Pts',(39.3940995760289,-9.68364100883828,0.));
#19486=CARTESIAN_POINT('Ctrl Pts',(39.3940995760289,-9.68364100883828,18.));
#19487=CARTESIAN_POINT('Ctrl Pts',(39.3137321153686,-9.62584947846544,0.));
#19488=CARTESIAN_POINT('Ctrl Pts',(39.3137321153686,-9.62584947846544,18.));
#19489=CARTESIAN_POINT('Ctrl Pts',(39.2330959982788,-9.56867984233624,0.));
#19490=CARTESIAN_POINT('Ctrl Pts',(39.2330959982788,-9.56867984233624,18.));
#19491=CARTESIAN_POINT('Ctrl Pts',(39.1521903958955,-9.51214104535621,0.));
#19492=CARTESIAN_POINT('Ctrl Pts',(39.1521903958955,-9.51214104535621,18.));
#19493=CARTESIAN_POINT('Ctrl Pts',(39.0710161994951,-9.45623664577432,0.));
#19494=CARTESIAN_POINT('Ctrl Pts',(39.0710161994951,-9.45623664577432,18.));
#19495=CARTESIAN_POINT('Ctrl Pts',(38.9895756526779,-9.40096600877644,0.));
#19496=CARTESIAN_POINT('Ctrl Pts',(38.9895756526779,-9.40096600877644,18.));
#19497=CARTESIAN_POINT('Ctrl Pts',(38.9078708427078,-9.34632917154637,0.));
#19498=CARTESIAN_POINT('Ctrl Pts',(38.9078708427078,-9.34632917154637,18.));
#19499=CARTESIAN_POINT('Ctrl Pts',(38.8259023794241,-9.29233110570904,0.));
#19500=CARTESIAN_POINT('Ctrl Pts',(38.8259023794241,-9.29233110570904,18.));
#19501=CARTESIAN_POINT('Ctrl Pts',(38.7436682576832,-9.23898539199332,0.));
#19502=CARTESIAN_POINT('Ctrl Pts',(38.7436682576832,-9.23898539199332,18.));
#19503=CARTESIAN_POINT('Ctrl Pts',(38.6611620045193,-9.1863201939433,0.));
#19504=CARTESIAN_POINT('Ctrl Pts',(38.6611620045193,-9.1863201939433,18.));
#19505=CARTESIAN_POINT('Ctrl Pts',(38.5783736628826,-9.13437512010587,0.));
#19506=CARTESIAN_POINT('Ctrl Pts',(38.5783736628826,-9.13437512010587,18.));
#19507=CARTESIAN_POINT('Ctrl Pts',(38.4952932486131,-9.08319014288087,0.));
#19508=CARTESIAN_POINT('Ctrl Pts',(38.4952932486131,-9.08319014288087,18.));
#19509=CARTESIAN_POINT('Ctrl Pts',(38.4119138099805,-9.03279579360191,0.));
#19510=CARTESIAN_POINT('Ctrl Pts',(38.4119138099805,-9.03279579360191,18.));
#19511=CARTESIAN_POINT('Ctrl Pts',(38.3282340281403,-8.98320483785761,0.));
#19512=CARTESIAN_POINT('Ctrl Pts',(38.3282340281403,-8.98320483785761,18.));
#19513=CARTESIAN_POINT('Ctrl Pts',(38.2442625706309,-8.9343983099634,0.));
#19514=CARTESIAN_POINT('Ctrl Pts',(38.2442625706309,-8.9343983099634,18.));
#19515=CARTESIAN_POINT('Ctrl Pts',(38.1600150482528,-8.88633535238435,0.));
#19516=CARTESIAN_POINT('Ctrl Pts',(38.1600150482528,-8.88633535238435,18.));
#19517=CARTESIAN_POINT('Ctrl Pts',(38.0755058326913,-8.8389795976335,0.));
#19518=CARTESIAN_POINT('Ctrl Pts',(38.0755058326913,-8.8389795976335,18.));
#19519=CARTESIAN_POINT('Ctrl Pts',(37.9907407304174,-8.79232279131093,0.));
#19520=CARTESIAN_POINT('Ctrl Pts',(37.9907407304174,-8.79232279131093,18.));
#19521=CARTESIAN_POINT('Ctrl Pts',(37.9057107230066,-8.74640499479003,0.));
#19522=CARTESIAN_POINT('Ctrl Pts',(37.9057107230066,-8.74640499479003,18.));
#19523=CARTESIAN_POINT('Ctrl Pts',(37.8203816669031,-8.70134776631144,0.));
#19524=CARTESIAN_POINT('Ctrl Pts',(37.8203816669031,-8.70134776631144,18.));
#19525=CARTESIAN_POINT('Ctrl Pts',(37.7347032383719,-8.65732553894525,0.));
#19526=CARTESIAN_POINT('Ctrl Pts',(37.7347032383719,-8.65732553894525,18.));
#19527=CARTESIAN_POINT('Ctrl Pts',(37.6486274754754,-8.61450621749156,0.));
#19528=CARTESIAN_POINT('Ctrl Pts',(37.6486274754754,-8.61450621749156,18.));
#19529=CARTESIAN_POINT('Ctrl Pts',(37.5621256752108,-8.57299698459467,0.));
#19530=CARTESIAN_POINT('Ctrl Pts',(37.5621256752108,-8.57299698459467,18.));
#19531=CARTESIAN_POINT('Ctrl Pts',(37.4752030152968,-8.53279758643785,0.));
#19532=CARTESIAN_POINT('Ctrl Pts',(37.4752030152968,-8.53279758643785,18.));
#19533=CARTESIAN_POINT('Ctrl Pts',(37.3879218093514,-8.49372546467076,0.));
#19534=CARTESIAN_POINT('Ctrl Pts',(37.3879218093514,-8.49372546467076,18.));
#19535=CARTESIAN_POINT('Ctrl Pts',(37.3003733151561,-8.45550849433961,0.));
#19536=CARTESIAN_POINT('Ctrl Pts',(37.3003733151561,-8.45550849433961,18.));
#19537=CARTESIAN_POINT('Ctrl Pts',(37.2126332013933,-8.41793088313261,0.));
#19538=CARTESIAN_POINT('Ctrl Pts',(37.2126332013933,-8.41793088313261,18.));
#19539=CARTESIAN_POINT('Ctrl Pts',(37.1247207489179,-8.38096706211449,0.));
#19540=CARTESIAN_POINT('Ctrl Pts',(37.1247207489179,-8.38096706211449,18.));
#19541=CARTESIAN_POINT('Ctrl Pts',(37.0365602155148,-8.3449081895264,0.));
#19542=CARTESIAN_POINT('Ctrl Pts',(37.0365602155148,-8.3449081895264,18.));
#19543=CARTESIAN_POINT('Ctrl Pts',(36.9479311729484,-8.31052547794592,0.));
#19544=CARTESIAN_POINT('Ctrl Pts',(36.9479311729484,-8.31052547794592,18.));
#19545=CARTESIAN_POINT('Ctrl Pts',(36.8585291300917,-8.27886599440786,0.));
#19546=CARTESIAN_POINT('Ctrl Pts',(36.8585291300917,-8.27886599440786,18.));
#19547=CARTESIAN_POINT('Ctrl Pts',(36.7861403757604,-8.25656657451821,0.));
#19548=CARTESIAN_POINT('Ctrl Pts',(36.7861403757604,-8.25656657451821,18.));
#19549=CARTESIAN_POINT('Ctrl Pts',(36.7312504697652,-8.24192165947368,0.));
#19550=CARTESIAN_POINT('Ctrl Pts',(36.7312504697652,-8.24192165947368,18.));
#19551=CARTESIAN_POINT('Ctrl Pts',(36.6943771018148,-8.23313075335377,0.));
#19552=CARTESIAN_POINT('Ctrl Pts',(36.6943771018148,-8.23313075335377,18.));
#19553=CARTESIAN_POINT('Ctrl Pts',(36.6758703925241,-8.22897839625062,0.));
#19554=CARTESIAN_POINT('Ctrl Pts',(36.6758703925241,-8.22897839625062,18.));
#19555=CARTESIAN_POINT('',(42.2550026135057,-12.2684454652017,0.));
#19556=CARTESIAN_POINT('Ctrl Pts',(36.6758703925241,-8.22897839625062,0.));
#19557=CARTESIAN_POINT('Ctrl Pts',(36.6943771018148,-8.23313075335377,0.));
#19558=CARTESIAN_POINT('Ctrl Pts',(36.7312504697652,-8.24192165947368,0.));
#19559=CARTESIAN_POINT('Ctrl Pts',(36.7861403757604,-8.25656657451821,0.));
#19560=CARTESIAN_POINT('Ctrl Pts',(36.8585291300917,-8.27886599440786,0.));
#19561=CARTESIAN_POINT('Ctrl Pts',(36.9479311729484,-8.31052547794592,0.));
#19562=CARTESIAN_POINT('Ctrl Pts',(37.0365602155148,-8.3449081895264,0.));
#19563=CARTESIAN_POINT('Ctrl Pts',(37.1247207489179,-8.38096706211449,0.));
#19564=CARTESIAN_POINT('Ctrl Pts',(37.2126332013933,-8.41793088313261,0.));
#19565=CARTESIAN_POINT('Ctrl Pts',(37.3003733151561,-8.45550849433961,0.));
#19566=CARTESIAN_POINT('Ctrl Pts',(37.3879218093514,-8.49372546467076,0.));
#19567=CARTESIAN_POINT('Ctrl Pts',(37.4752030152968,-8.53279758643785,0.));
#19568=CARTESIAN_POINT('Ctrl Pts',(37.5621256752108,-8.57299698459467,0.));
#19569=CARTESIAN_POINT('Ctrl Pts',(37.6486274754754,-8.61450621749156,0.));
#19570=CARTESIAN_POINT('Ctrl Pts',(37.7347032383719,-8.65732553894525,0.));
#19571=CARTESIAN_POINT('Ctrl Pts',(37.8203816669031,-8.70134776631144,0.));
#19572=CARTESIAN_POINT('Ctrl Pts',(37.9057107230066,-8.74640499479003,0.));
#19573=CARTESIAN_POINT('Ctrl Pts',(37.9907407304174,-8.79232279131093,0.));
#19574=CARTESIAN_POINT('Ctrl Pts',(38.0755058326913,-8.8389795976335,0.));
#19575=CARTESIAN_POINT('Ctrl Pts',(38.1600150482528,-8.88633535238435,0.));
#19576=CARTESIAN_POINT('Ctrl Pts',(38.2442625706309,-8.9343983099634,0.));
#19577=CARTESIAN_POINT('Ctrl Pts',(38.3282340281403,-8.98320483785761,0.));
#19578=CARTESIAN_POINT('Ctrl Pts',(38.4119138099805,-9.03279579360191,0.));
#19579=CARTESIAN_POINT('Ctrl Pts',(38.4952932486131,-9.08319014288087,0.));
#19580=CARTESIAN_POINT('Ctrl Pts',(38.5783736628826,-9.13437512010587,0.));
#19581=CARTESIAN_POINT('Ctrl Pts',(38.6611620045193,-9.1863201939433,0.));
#19582=CARTESIAN_POINT('Ctrl Pts',(38.7436682576832,-9.23898539199332,0.));
#19583=CARTESIAN_POINT('Ctrl Pts',(38.8259023794241,-9.29233110570904,0.));
#19584=CARTESIAN_POINT('Ctrl Pts',(38.9078708427078,-9.34632917154637,0.));
#19585=CARTESIAN_POINT('Ctrl Pts',(38.9895756526779,-9.40096600877644,0.));
#19586=CARTESIAN_POINT('Ctrl Pts',(39.0710161994951,-9.45623664577432,0.));
#19587=CARTESIAN_POINT('Ctrl Pts',(39.1521903958955,-9.51214104535621,0.));
#19588=CARTESIAN_POINT('Ctrl Pts',(39.2330959982788,-9.56867984233624,0.));
#19589=CARTESIAN_POINT('Ctrl Pts',(39.3137321153686,-9.62584947846544,0.));
#19590=CARTESIAN_POINT('Ctrl Pts',(39.3940995760289,-9.68364100883828,0.));
#19591=CARTESIAN_POINT('Ctrl Pts',(39.4742001555227,-9.74204258152664,0.));
#19592=CARTESIAN_POINT('Ctrl Pts',(39.5540361022309,-9.80104095251614,0.));
#19593=CARTESIAN_POINT('Ctrl Pts',(39.6336095893767,-9.86062324242561,0.));
#19594=CARTESIAN_POINT('Ctrl Pts',(39.712922089547,-9.92077894513193,0.));
#19595=CARTESIAN_POINT('Ctrl Pts',(39.7919742367922,-9.98150036150824,0.));
#19596=CARTESIAN_POINT('Ctrl Pts',(39.8707661565233,-10.0427815229883,0.));
#19597=CARTESIAN_POINT('Ctrl Pts',(39.9492976736738,-10.1046175096878,0.));
#19598=CARTESIAN_POINT('Ctrl Pts',(40.0275685525923,-10.1670036683795,0.));
#19599=CARTESIAN_POINT('Ctrl Pts',(40.1055787732578,-10.2299347125857,0.));
#19600=CARTESIAN_POINT('Ctrl Pts',(40.1833286010098,-10.2934044990237,0.));
#19601=CARTESIAN_POINT('Ctrl Pts',(40.2608184485326,-10.3574064830678,0.));
#19602=CARTESIAN_POINT('Ctrl Pts',(40.3380487942952,-10.4219339932951,0.));
#19603=CARTESIAN_POINT('Ctrl Pts',(40.4150200869536,-10.48698054978,0.));
#19604=CARTESIAN_POINT('Ctrl Pts',(40.4917326404439,-10.5525402237951,0.));
#19605=CARTESIAN_POINT('Ctrl Pts',(40.5681866012103,-10.618607730849,0.));
#19606=CARTESIAN_POINT('Ctrl Pts',(40.6443819999244,-10.6851782157325,0.));
#19607=CARTESIAN_POINT('Ctrl Pts',(40.7203187831783,-10.7522471109694,0.));
#19608=CARTESIAN_POINT('Ctrl Pts',(40.7959968527561,-10.8198099757795,0.));
#19609=CARTESIAN_POINT('Ctrl Pts',(40.8714161092412,-10.8878623066647,0.));
#19610=CARTESIAN_POINT('Ctrl Pts',(40.9465764747798,-10.956399476781,0.));
#19611=CARTESIAN_POINT('Ctrl Pts',(41.0214778832142,-11.0254168609972,0.));
#19612=CARTESIAN_POINT('Ctrl Pts',(41.0961202807715,-11.0949099155251,0.));
#19613=CARTESIAN_POINT('Ctrl Pts',(41.1705036228854,-11.1648742640378,0.));
#19614=CARTESIAN_POINT('Ctrl Pts',(41.2446278781981,-11.2353057980338,0.));
#19615=CARTESIAN_POINT('Ctrl Pts',(41.3184930194148,-11.3062006993745,0.));
#19616=CARTESIAN_POINT('Ctrl Pts',(41.3920989905986,-11.3775553120177,0.));
#19617=CARTESIAN_POINT('Ctrl Pts',(41.4654456796071,-11.449366039385,0.));
#19618=CARTESIAN_POINT('Ctrl Pts',(41.5385328935506,-11.5216292382388,0.));
#19619=CARTESIAN_POINT('Ctrl Pts',(41.6113603270596,-11.5943410868252,0.));
#19620=CARTESIAN_POINT('Ctrl Pts',(41.6839275596248,-11.6674975352852,0.));
#19621=CARTESIAN_POINT('Ctrl Pts',(41.7562341395977,-11.7410945211992,0.));
#19622=CARTESIAN_POINT('Ctrl Pts',(41.8282796562569,-11.81512813804,0.));
#19623=CARTESIAN_POINT('Ctrl Pts',(41.9000638152266,-11.8895948153349,0.));
#19624=CARTESIAN_POINT('Ctrl Pts',(41.9715865222182,-11.9644914999263,0.));
#19625=CARTESIAN_POINT('Ctrl Pts',(42.0571002269437,-12.054880669507,0.));
#19626=CARTESIAN_POINT('Ctrl Pts',(42.1280354231517,-12.1307372881904,0.));
#19627=CARTESIAN_POINT('Ctrl Pts',(42.18457517013,-12.1917619768791,0.));
#19628=CARTESIAN_POINT('Ctrl Pts',(42.2268628664988,-12.2377212115625,0.));
#19629=CARTESIAN_POINT('Ctrl Pts',(42.2550026135057,-12.2684454652018,0.));
#19630=CARTESIAN_POINT('',(42.2550026135057,-12.2684454652017,15.));
#19631=CARTESIAN_POINT('Ctrl Pts',(42.2550026135057,-12.2684454652018,15.));
#19632=CARTESIAN_POINT('Ctrl Pts',(42.2409327400055,-12.2530833383985,15.));
#19633=CARTESIAN_POINT('Ctrl Pts',(42.2127669677092,-12.222401466668,15.));
#19634=CARTESIAN_POINT('Ctrl Pts',(42.1704402333854,-12.1765058047069,15.));
#19635=CARTESIAN_POINT('Ctrl Pts',(42.1138483839101,-12.1155659644537,15.));
#19636=CARTESIAN_POINT('Ctrl Pts',(42.0428479428228,-12.0398158079102,15.));
#19637=CARTESIAN_POINT('Ctrl Pts',(41.9715865222182,-11.9644914999263,15.));
#19638=CARTESIAN_POINT('Ctrl Pts',(41.9000638152266,-11.8895948153349,15.));
#19639=CARTESIAN_POINT('Ctrl Pts',(41.8282796562569,-11.81512813804,15.));
#19640=CARTESIAN_POINT('Ctrl Pts',(41.7562341395977,-11.7410945211992,15.));
#19641=CARTESIAN_POINT('Ctrl Pts',(41.6839275596248,-11.6674975352852,15.));
#19642=CARTESIAN_POINT('Ctrl Pts',(41.6113603270596,-11.5943410868252,15.));
#19643=CARTESIAN_POINT('Ctrl Pts',(41.5385328935506,-11.5216292382388,15.));
#19644=CARTESIAN_POINT('Ctrl Pts',(41.4654456796071,-11.449366039385,15.));
#19645=CARTESIAN_POINT('Ctrl Pts',(41.3920989905986,-11.3775553120177,15.));
#19646=CARTESIAN_POINT('Ctrl Pts',(41.3184930194148,-11.3062006993745,15.));
#19647=CARTESIAN_POINT('Ctrl Pts',(41.2446278781981,-11.2353057980338,15.));
#19648=CARTESIAN_POINT('Ctrl Pts',(41.1705036228854,-11.1648742640378,15.));
#19649=CARTESIAN_POINT('Ctrl Pts',(41.0961202807715,-11.0949099155251,15.));
#19650=CARTESIAN_POINT('Ctrl Pts',(41.0214778832142,-11.0254168609972,15.));
#19651=CARTESIAN_POINT('Ctrl Pts',(40.9465764747798,-10.956399476781,15.));
#19652=CARTESIAN_POINT('Ctrl Pts',(40.8714161092412,-10.8878623066647,15.));
#19653=CARTESIAN_POINT('Ctrl Pts',(40.7959968527561,-10.8198099757795,15.));
#19654=CARTESIAN_POINT('Ctrl Pts',(40.7203187831783,-10.7522471109694,15.));
#19655=CARTESIAN_POINT('Ctrl Pts',(40.6443819999244,-10.6851782157325,15.));
#19656=CARTESIAN_POINT('Ctrl Pts',(40.5681866012103,-10.618607730849,15.));
#19657=CARTESIAN_POINT('Ctrl Pts',(40.4917326404439,-10.5525402237951,15.));
#19658=CARTESIAN_POINT('Ctrl Pts',(40.4150200869536,-10.48698054978,15.));
#19659=CARTESIAN_POINT('Ctrl Pts',(40.3380487942952,-10.4219339932951,15.));
#19660=CARTESIAN_POINT('Ctrl Pts',(40.2608184485326,-10.3574064830678,15.));
#19661=CARTESIAN_POINT('Ctrl Pts',(40.1833286010098,-10.2934044990237,15.));
#19662=CARTESIAN_POINT('Ctrl Pts',(40.1055787732578,-10.2299347125857,15.));
#19663=CARTESIAN_POINT('Ctrl Pts',(40.0275685525923,-10.1670036683795,15.));
#19664=CARTESIAN_POINT('Ctrl Pts',(39.9492976736738,-10.1046175096878,15.));
#19665=CARTESIAN_POINT('Ctrl Pts',(39.8707661565233,-10.0427815229883,15.));
#19666=CARTESIAN_POINT('Ctrl Pts',(39.7919742367922,-9.98150036150824,15.));
#19667=CARTESIAN_POINT('Ctrl Pts',(39.712922089547,-9.92077894513193,15.));
#19668=CARTESIAN_POINT('Ctrl Pts',(39.6336095893767,-9.86062324242561,15.));
#19669=CARTESIAN_POINT('Ctrl Pts',(39.5540361022309,-9.80104095251614,15.));
#19670=CARTESIAN_POINT('Ctrl Pts',(39.4742001555227,-9.74204258152664,15.));
#19671=CARTESIAN_POINT('Ctrl Pts',(39.3940995760289,-9.68364100883828,15.));
#19672=CARTESIAN_POINT('Ctrl Pts',(39.3137321153686,-9.62584947846544,15.));
#19673=CARTESIAN_POINT('Ctrl Pts',(39.2330959982788,-9.56867984233624,15.));
#19674=CARTESIAN_POINT('Ctrl Pts',(39.1521903958955,-9.51214104535621,15.));
#19675=CARTESIAN_POINT('Ctrl Pts',(39.0710161994951,-9.45623664577432,15.));
#19676=CARTESIAN_POINT('Ctrl Pts',(38.9895756526779,-9.40096600877644,15.));
#19677=CARTESIAN_POINT('Ctrl Pts',(38.9078708427078,-9.34632917154637,15.));
#19678=CARTESIAN_POINT('Ctrl Pts',(38.8259023794241,-9.29233110570904,15.));
#19679=CARTESIAN_POINT('Ctrl Pts',(38.7436682576832,-9.23898539199332,15.));
#19680=CARTESIAN_POINT('Ctrl Pts',(38.6611620045193,-9.1863201939433,15.));
#19681=CARTESIAN_POINT('Ctrl Pts',(38.5783736628826,-9.13437512010587,15.));
#19682=CARTESIAN_POINT('Ctrl Pts',(38.4952932486131,-9.08319014288087,15.));
#19683=CARTESIAN_POINT('Ctrl Pts',(38.4119138099805,-9.03279579360191,15.));
#19684=CARTESIAN_POINT('Ctrl Pts',(38.3282340281403,-8.98320483785761,15.));
#19685=CARTESIAN_POINT('Ctrl Pts',(38.2442625706309,-8.9343983099634,15.));
#19686=CARTESIAN_POINT('Ctrl Pts',(38.1600150482528,-8.88633535238435,15.));
#19687=CARTESIAN_POINT('Ctrl Pts',(38.0755058326913,-8.8389795976335,15.));
#19688=CARTESIAN_POINT('Ctrl Pts',(37.9907407304174,-8.79232279131093,15.));
#19689=CARTESIAN_POINT('Ctrl Pts',(37.9057107230066,-8.74640499479003,15.));
#19690=CARTESIAN_POINT('Ctrl Pts',(37.8203816669031,-8.70134776631144,15.));
#19691=CARTESIAN_POINT('Ctrl Pts',(37.7347032383719,-8.65732553894525,15.));
#19692=CARTESIAN_POINT('Ctrl Pts',(37.6486274754754,-8.61450621749156,15.));
#19693=CARTESIAN_POINT('Ctrl Pts',(37.5621256752108,-8.57299698459467,15.));
#19694=CARTESIAN_POINT('Ctrl Pts',(37.4752030152968,-8.53279758643785,15.));
#19695=CARTESIAN_POINT('Ctrl Pts',(37.3879218093514,-8.49372546467076,15.));
#19696=CARTESIAN_POINT('Ctrl Pts',(37.3003733151561,-8.45550849433961,15.));
#19697=CARTESIAN_POINT('Ctrl Pts',(37.2126332013933,-8.41793088313261,15.));
#19698=CARTESIAN_POINT('Ctrl Pts',(37.1247207489179,-8.38096706211449,15.));
#19699=CARTESIAN_POINT('Ctrl Pts',(37.0365602155148,-8.3449081895264,15.));
#19700=CARTESIAN_POINT('Ctrl Pts',(36.9479311729484,-8.31052547794592,15.));
#19701=CARTESIAN_POINT('Ctrl Pts',(36.8585291300917,-8.27886599440786,15.));
#19702=CARTESIAN_POINT('Ctrl Pts',(36.7861403757604,-8.25656657451821,15.));
#19703=CARTESIAN_POINT('Ctrl Pts',(36.7312504697652,-8.24192165947368,15.));
#19704=CARTESIAN_POINT('Ctrl Pts',(36.6943771018148,-8.23313075335377,15.));
#19705=CARTESIAN_POINT('Ctrl Pts',(36.6758703925241,-8.22897839625062,15.));
#19706=CARTESIAN_POINT('',(42.2550026135057,-12.2684454652017,0.));
#19707=CARTESIAN_POINT('Origin',(1.07784724682657E-11,-3.50213800024364E-12,
0.));
#19708=CARTESIAN_POINT('',(41.396226524684,-14.911486495888,0.));
#19709=CARTESIAN_POINT('Origin',(1.07784724682657E-11,-3.50213800024364E-12,
0.));
#19710=CARTESIAN_POINT('',(41.396226524684,-14.911486495888,15.));
#19711=CARTESIAN_POINT('Origin',(1.07784724682657E-11,-3.50213800024364E-12,
15.));
#19712=CARTESIAN_POINT('',(41.396226524684,-14.911486495888,0.));
#19713=CARTESIAN_POINT('Ctrl Pts',(34.5082745737944,-14.9001523628048,0.));
#19714=CARTESIAN_POINT('Ctrl Pts',(34.5082745737944,-14.9001523628048,18.));
#19715=CARTESIAN_POINT('Ctrl Pts',(34.525687510388,-14.9076710061311,0.));
#19716=CARTESIAN_POINT('Ctrl Pts',(34.525687510388,-14.9076710061311,18.));
#19717=CARTESIAN_POINT('Ctrl Pts',(34.5606858566713,-14.9222326355678,0.));
#19718=CARTESIAN_POINT('Ctrl Pts',(34.5606858566713,-14.9222326355678,18.));
#19719=CARTESIAN_POINT('Ctrl Pts',(34.6137007885254,-14.9426481276593,0.));
#19720=CARTESIAN_POINT('Ctrl Pts',(34.6137007885254,-14.9426481276593,18.));
#19721=CARTESIAN_POINT('Ctrl Pts',(34.6853717911268,-14.9671565602316,0.));
#19722=CARTESIAN_POINT('Ctrl Pts',(34.6853717911268,-14.9671565602316,18.));
#19723=CARTESIAN_POINT('Ctrl Pts',(34.7763085406486,-14.9940927023322,0.));
#19724=CARTESIAN_POINT('Ctrl Pts',(34.7763085406486,-14.9940927023322,18.));
#19725=CARTESIAN_POINT('Ctrl Pts',(34.8682205930809,-15.0183713484962,0.));
#19726=CARTESIAN_POINT('Ctrl Pts',(34.8682205930809,-15.0183713484962,18.));
#19727=CARTESIAN_POINT('Ctrl Pts',(34.9607388363587,-15.041018569143,0.));
#19728=CARTESIAN_POINT('Ctrl Pts',(34.9607388363587,-15.041018569143,18.));
#19729=CARTESIAN_POINT('Ctrl Pts',(35.0535882932913,-15.0627878528202,0.));
#19730=CARTESIAN_POINT('Ctrl Pts',(35.0535882932913,-15.0627878528202,18.));
#19731=CARTESIAN_POINT('Ctrl Pts',(35.1466591020976,-15.08395927165,0.));
#19732=CARTESIAN_POINT('Ctrl Pts',(35.1466591020976,-15.08395927165,18.));
#19733=CARTESIAN_POINT('Ctrl Pts',(35.2399506932815,-15.104500806927,0.));
#19734=CARTESIAN_POINT('Ctrl Pts',(35.2399506932815,-15.104500806927,18.));
#19735=CARTESIAN_POINT('Ctrl Pts',(35.3335286891314,-15.1241934020682,0.));
#19736=CARTESIAN_POINT('Ctrl Pts',(35.3335286891314,-15.1241934020682,18.));
#19737=CARTESIAN_POINT('Ctrl Pts',(35.4274792115856,-15.1427632633831,0.));
#19738=CARTESIAN_POINT('Ctrl Pts',(35.4274792115856,-15.1427632633831,18.));
#19739=CARTESIAN_POINT('Ctrl Pts',(35.5218591529745,-15.1600260710384,0.));
#19740=CARTESIAN_POINT('Ctrl Pts',(35.5218591529745,-15.1600260710384,18.));
#19741=CARTESIAN_POINT('Ctrl Pts',(35.6166644736253,-15.1759785763051,0.));
#19742=CARTESIAN_POINT('Ctrl Pts',(35.6166644736253,-15.1759785763051,18.));
#19743=CARTESIAN_POINT('Ctrl Pts',(35.7118553943773,-15.1907243629659,0.));
#19744=CARTESIAN_POINT('Ctrl Pts',(35.7118553943773,-15.1907243629659,18.));
#19745=CARTESIAN_POINT('Ctrl Pts',(35.8073720252878,-15.2044274601769,0.));
#19746=CARTESIAN_POINT('Ctrl Pts',(35.8073720252878,-15.2044274601769,18.));
#19747=CARTESIAN_POINT('Ctrl Pts',(35.9031525499277,-15.2172585668056,0.));
#19748=CARTESIAN_POINT('Ctrl Pts',(35.9031525499277,-15.2172585668056,18.));
#19749=CARTESIAN_POINT('Ctrl Pts',(35.9991531408727,-15.2293360946131,0.));
#19750=CARTESIAN_POINT('Ctrl Pts',(35.9991531408727,-15.2293360946131,18.));
#19751=CARTESIAN_POINT('Ctrl Pts',(36.095357546697,-15.240697754828,0.));
#19752=CARTESIAN_POINT('Ctrl Pts',(36.095357546697,-15.240697754828,18.));
#19753=CARTESIAN_POINT('Ctrl Pts',(36.1917659216814,-15.2513334565427,0.));
#19754=CARTESIAN_POINT('Ctrl Pts',(36.1917659216814,-15.2513334565427,18.));
#19755=CARTESIAN_POINT('Ctrl Pts',(36.2883880151607,-15.2612053303774,0.));
#19756=CARTESIAN_POINT('Ctrl Pts',(36.2883880151607,-15.2612053303774,18.));
#19757=CARTESIAN_POINT('Ctrl Pts',(36.3852352131887,-15.2702711460937,0.));
#19758=CARTESIAN_POINT('Ctrl Pts',(36.3852352131887,-15.2702711460937,18.));
#19759=CARTESIAN_POINT('Ctrl Pts',(36.4823116513289,-15.2785104654792,0.));
#19760=CARTESIAN_POINT('Ctrl Pts',(36.4823116513289,-15.2785104654792,18.));
#19761=CARTESIAN_POINT('Ctrl Pts',(36.5796108931244,-15.2859343913094,0.));
#19762=CARTESIAN_POINT('Ctrl Pts',(36.5796108931244,-15.2859343913094,18.));
#19763=CARTESIAN_POINT('Ctrl Pts',(36.6771206167755,-15.2925717100767,0.));
#19764=CARTESIAN_POINT('Ctrl Pts',(36.6771206167755,-15.2925717100767,18.));
#19765=CARTESIAN_POINT('Ctrl Pts',(36.7748254044502,-15.2984606286738,0.));
#19766=CARTESIAN_POINT('Ctrl Pts',(36.7748254044502,-15.2984606286738,18.));
#19767=CARTESIAN_POINT('Ctrl Pts',(36.8727100302512,-15.3036390436952,0.));
#19768=CARTESIAN_POINT('Ctrl Pts',(36.8727100302512,-15.3036390436952,18.));
#19769=CARTESIAN_POINT('Ctrl Pts',(36.970763176802,-15.3081335446406,0.));
#19770=CARTESIAN_POINT('Ctrl Pts',(36.970763176802,-15.3081335446406,18.));
#19771=CARTESIAN_POINT('Ctrl Pts',(37.0689784837457,-15.3119562971444,0.));
#19772=CARTESIAN_POINT('Ctrl Pts',(37.0689784837457,-15.3119562971444,18.));
#19773=CARTESIAN_POINT('Ctrl Pts',(37.1673525354641,-15.3151109648809,0.));
#19774=CARTESIAN_POINT('Ctrl Pts',(37.1673525354641,-15.3151109648809,18.));
#19775=CARTESIAN_POINT('Ctrl Pts',(37.2658836214694,-15.3175963510698,0.));
#19776=CARTESIAN_POINT('Ctrl Pts',(37.2658836214694,-15.3175963510698,18.));
#19777=CARTESIAN_POINT('Ctrl Pts',(37.3645702997848,-15.3194106233802,0.));
#19778=CARTESIAN_POINT('Ctrl Pts',(37.3645702997848,-15.3194106233802,18.));
#19779=CARTESIAN_POINT('Ctrl Pts',(37.4634097578665,-15.3205561366169,0.));
#19780=CARTESIAN_POINT('Ctrl Pts',(37.4634097578665,-15.3205561366169,18.));
#19781=CARTESIAN_POINT('Ctrl Pts',(37.562397408596,-15.3210406145546,0.));
#19782=CARTESIAN_POINT('Ctrl Pts',(37.562397408596,-15.3210406145546,18.));
#19783=CARTESIAN_POINT('Ctrl Pts',(37.6615277218027,-15.3208746890781,0.));
#19784=CARTESIAN_POINT('Ctrl Pts',(37.6615277218027,-15.3208746890781,18.));
#19785=CARTESIAN_POINT('Ctrl Pts',(37.7607947318286,-15.320070396385,0.));
#19786=CARTESIAN_POINT('Ctrl Pts',(37.7607947318286,-15.320070396385,18.));
#19787=CARTESIAN_POINT('Ctrl Pts',(37.8601926265378,-15.3186394335023,0.));
#19788=CARTESIAN_POINT('Ctrl Pts',(37.8601926265378,-15.3186394335023,18.));
#19789=CARTESIAN_POINT('Ctrl Pts',(37.959716421934,-15.3165911656268,0.));
#19790=CARTESIAN_POINT('Ctrl Pts',(37.959716421934,-15.3165911656268,18.));
#19791=CARTESIAN_POINT('Ctrl Pts',(38.0593621055415,-15.3139321941687,0.));
#19792=CARTESIAN_POINT('Ctrl Pts',(38.0593621055415,-15.3139321941687,18.));
#19793=CARTESIAN_POINT('Ctrl Pts',(38.1591262705847,-15.310667421514,0.));
#19794=CARTESIAN_POINT('Ctrl Pts',(38.1591262705847,-15.310667421514,18.));
#19795=CARTESIAN_POINT('Ctrl Pts',(38.2590058835965,-15.3068007250314,0.));
#19796=CARTESIAN_POINT('Ctrl Pts',(38.2590058835965,-15.3068007250314,18.));
#19797=CARTESIAN_POINT('Ctrl Pts',(38.3589980188324,-15.3023357307483,0.));
#19798=CARTESIAN_POINT('Ctrl Pts',(38.3589980188324,-15.3023357307483,18.));
#19799=CARTESIAN_POINT('Ctrl Pts',(38.4590995527814,-15.297276703747,0.));
#19800=CARTESIAN_POINT('Ctrl Pts',(38.4590995527814,-15.297276703747,18.));
#19801=CARTESIAN_POINT('Ctrl Pts',(38.5593070891769,-15.2916287700102,0.));
#19802=CARTESIAN_POINT('Ctrl Pts',(38.5593070891769,-15.2916287700102,18.));
#19803=CARTESIAN_POINT('Ctrl Pts',(38.659617115053,-15.2853974668211,0.));
#19804=CARTESIAN_POINT('Ctrl Pts',(38.659617115053,-15.2853974668211,18.));
#19805=CARTESIAN_POINT('Ctrl Pts',(38.7600260961351,-15.2785884727112,0.));
#19806=CARTESIAN_POINT('Ctrl Pts',(38.7600260961351,-15.2785884727112,18.));
#19807=CARTESIAN_POINT('Ctrl Pts',(38.860530586589,-15.2712072937639,0.));
#19808=CARTESIAN_POINT('Ctrl Pts',(38.860530586589,-15.2712072937639,18.));
#19809=CARTESIAN_POINT('Ctrl Pts',(38.9611273555758,-15.2632589109473,0.));
#19810=CARTESIAN_POINT('Ctrl Pts',(38.9611273555758,-15.2632589109473,18.));
#19811=CARTESIAN_POINT('Ctrl Pts',(39.061813415425,-15.2547476855825,0.));
#19812=CARTESIAN_POINT('Ctrl Pts',(39.061813415425,-15.2547476855825,18.));
#19813=CARTESIAN_POINT('Ctrl Pts',(39.1625859371304,-15.2456775636447,0.));
#19814=CARTESIAN_POINT('Ctrl Pts',(39.1625859371304,-15.2456775636447,18.));
#19815=CARTESIAN_POINT('Ctrl Pts',(39.2634421927888,-15.2360522089072,0.));
#19816=CARTESIAN_POINT('Ctrl Pts',(39.2634421927888,-15.2360522089072,18.));
#19817=CARTESIAN_POINT('Ctrl Pts',(39.3643794927167,-15.225875156307,0.));
#19818=CARTESIAN_POINT('Ctrl Pts',(39.3643794927167,-15.225875156307,18.));
#19819=CARTESIAN_POINT('Ctrl Pts',(39.4653951093947,-15.2151499908149,0.));
#19820=CARTESIAN_POINT('Ctrl Pts',(39.4653951093947,-15.2151499908149,18.));
#19821=CARTESIAN_POINT('Ctrl Pts',(39.5664862602472,-15.2038804098649,0.));
#19822=CARTESIAN_POINT('Ctrl Pts',(39.5664862602472,-15.2038804098649,18.));
#19823=CARTESIAN_POINT('Ctrl Pts',(39.6676501731673,-15.1920701163804,0.));
#19824=CARTESIAN_POINT('Ctrl Pts',(39.6676501731673,-15.1920701163804,18.));
#19825=CARTESIAN_POINT('Ctrl Pts',(39.7688841338802,-15.1797227547562,0.));
#19826=CARTESIAN_POINT('Ctrl Pts',(39.7688841338802,-15.1797227547562,18.));
#19827=CARTESIAN_POINT('Ctrl Pts',(39.8701855339908,-15.1668418393198,0.));
#19828=CARTESIAN_POINT('Ctrl Pts',(39.8701855339908,-15.1668418393198,18.));
#19829=CARTESIAN_POINT('Ctrl Pts',(39.9715519332134,-15.1534306754871,0.));
#19830=CARTESIAN_POINT('Ctrl Pts',(39.9715519332134,-15.1534306754871,18.));
#19831=CARTESIAN_POINT('Ctrl Pts',(40.0729810652204,-15.1394923361537,0.));
#19832=CARTESIAN_POINT('Ctrl Pts',(40.0729810652204,-15.1394923361537,18.));
#19833=CARTESIAN_POINT('Ctrl Pts',(40.1744707357902,-15.1250297462408,0.));
#19834=CARTESIAN_POINT('Ctrl Pts',(40.1744707357902,-15.1250297462408,18.));
#19835=CARTESIAN_POINT('Ctrl Pts',(40.2760187401821,-15.1100457495259,0.));
#19836=CARTESIAN_POINT('Ctrl Pts',(40.2760187401821,-15.1100457495259,18.));
#19837=CARTESIAN_POINT('Ctrl Pts',(40.3776227809037,-15.0945431800724,0.));
#19838=CARTESIAN_POINT('Ctrl Pts',(40.3776227809037,-15.0945431800724,18.));
#19839=CARTESIAN_POINT('Ctrl Pts',(40.4792803645352,-15.0785249502524,0.));
#19840=CARTESIAN_POINT('Ctrl Pts',(40.4792803645352,-15.0785249502524,18.));
#19841=CARTESIAN_POINT('Ctrl Pts',(40.58098877043,-15.0619940893017,0.));
#19842=CARTESIAN_POINT('Ctrl Pts',(40.58098877043,-15.0619940893017,18.));
#19843=CARTESIAN_POINT('Ctrl Pts',(40.6827452453667,-15.0449536183143,0.));
#19844=CARTESIAN_POINT('Ctrl Pts',(40.6827452453667,-15.0449536183143,18.));
#19845=CARTESIAN_POINT('Ctrl Pts',(40.7845471608654,-15.0274064563211,0.));
#19846=CARTESIAN_POINT('Ctrl Pts',(40.7845471608654,-15.0274064563211,18.));
#19847=CARTESIAN_POINT('Ctrl Pts',(40.8863921801,-15.0093553188655,0.));
#19848=CARTESIAN_POINT('Ctrl Pts',(40.8863921801,-15.0093553188655,18.));
#19849=CARTESIAN_POINT('Ctrl Pts',(40.9882784321884,-14.9908026205824,0.));
#19850=CARTESIAN_POINT('Ctrl Pts',(40.9882784321884,-14.9908026205824,18.));
#19851=CARTESIAN_POINT('Ctrl Pts',(41.0902046498729,-14.9717503874227,0.));
#19852=CARTESIAN_POINT('Ctrl Pts',(41.0902046498729,-14.9717503874227,18.));
#19853=CARTESIAN_POINT('Ctrl Pts',(41.1921700381957,-14.9522002356298,0.));
#19854=CARTESIAN_POINT('Ctrl Pts',(41.1921700381957,-14.9522002356298,18.));
#19855=CARTESIAN_POINT('Ctrl Pts',(41.2737733455422,-14.936162723752,0.));
#19856=CARTESIAN_POINT('Ctrl Pts',(41.2737733455422,-14.936162723752,18.));
#19857=CARTESIAN_POINT('Ctrl Pts',(41.3349931861715,-14.9239113834707,0.));
#19858=CARTESIAN_POINT('Ctrl Pts',(41.3349931861715,-14.9239113834707,18.));
#19859=CARTESIAN_POINT('Ctrl Pts',(41.3758141263348,-14.9156446533966,0.));
#19860=CARTESIAN_POINT('Ctrl Pts',(41.3758141263348,-14.9156446533966,18.));
#19861=CARTESIAN_POINT('Ctrl Pts',(41.396226524684,-14.911486495888,0.));
#19862=CARTESIAN_POINT('Ctrl Pts',(41.396226524684,-14.911486495888,18.));
#19863=CARTESIAN_POINT('Ctrl Pts',(34.5082745737944,-14.9001523628048,0.));
#19864=CARTESIAN_POINT('Ctrl Pts',(34.525687510388,-14.9076710061311,0.));
#19865=CARTESIAN_POINT('Ctrl Pts',(34.5606858566713,-14.9222326355678,0.));
#19866=CARTESIAN_POINT('Ctrl Pts',(34.6137007885254,-14.9426481276593,0.));
#19867=CARTESIAN_POINT('Ctrl Pts',(34.6853717911268,-14.9671565602316,0.));
#19868=CARTESIAN_POINT('Ctrl Pts',(34.7763085406486,-14.9940927023322,0.));
#19869=CARTESIAN_POINT('Ctrl Pts',(34.8682205930809,-15.0183713484962,0.));
#19870=CARTESIAN_POINT('Ctrl Pts',(34.9607388363587,-15.041018569143,0.));
#19871=CARTESIAN_POINT('Ctrl Pts',(35.0535882932913,-15.0627878528202,0.));
#19872=CARTESIAN_POINT('Ctrl Pts',(35.1466591020976,-15.08395927165,0.));
#19873=CARTESIAN_POINT('Ctrl Pts',(35.2399506932815,-15.104500806927,0.));
#19874=CARTESIAN_POINT('Ctrl Pts',(35.3335286891314,-15.1241934020682,0.));
#19875=CARTESIAN_POINT('Ctrl Pts',(35.4274792115856,-15.1427632633831,0.));
#19876=CARTESIAN_POINT('Ctrl Pts',(35.5218591529745,-15.1600260710384,0.));
#19877=CARTESIAN_POINT('Ctrl Pts',(35.6166644736253,-15.1759785763051,0.));
#19878=CARTESIAN_POINT('Ctrl Pts',(35.7118553943773,-15.1907243629659,0.));
#19879=CARTESIAN_POINT('Ctrl Pts',(35.8073720252878,-15.2044274601769,0.));
#19880=CARTESIAN_POINT('Ctrl Pts',(35.9031525499277,-15.2172585668056,0.));
#19881=CARTESIAN_POINT('Ctrl Pts',(35.9991531408727,-15.2293360946131,0.));
#19882=CARTESIAN_POINT('Ctrl Pts',(36.095357546697,-15.240697754828,0.));
#19883=CARTESIAN_POINT('Ctrl Pts',(36.1917659216814,-15.2513334565427,0.));
#19884=CARTESIAN_POINT('Ctrl Pts',(36.2883880151607,-15.2612053303774,0.));
#19885=CARTESIAN_POINT('Ctrl Pts',(36.3852352131887,-15.2702711460937,0.));
#19886=CARTESIAN_POINT('Ctrl Pts',(36.4823116513289,-15.2785104654792,0.));
#19887=CARTESIAN_POINT('Ctrl Pts',(36.5796108931244,-15.2859343913094,0.));
#19888=CARTESIAN_POINT('Ctrl Pts',(36.6771206167755,-15.2925717100767,0.));
#19889=CARTESIAN_POINT('Ctrl Pts',(36.7748254044502,-15.2984606286738,0.));
#19890=CARTESIAN_POINT('Ctrl Pts',(36.8727100302512,-15.3036390436952,0.));
#19891=CARTESIAN_POINT('Ctrl Pts',(36.970763176802,-15.3081335446406,0.));
#19892=CARTESIAN_POINT('Ctrl Pts',(37.0689784837457,-15.3119562971444,0.));
#19893=CARTESIAN_POINT('Ctrl Pts',(37.1673525354641,-15.3151109648809,0.));
#19894=CARTESIAN_POINT('Ctrl Pts',(37.2658836214694,-15.3175963510698,0.));
#19895=CARTESIAN_POINT('Ctrl Pts',(37.3645702997848,-15.3194106233802,0.));
#19896=CARTESIAN_POINT('Ctrl Pts',(37.4634097578665,-15.3205561366169,0.));
#19897=CARTESIAN_POINT('Ctrl Pts',(37.562397408596,-15.3210406145546,0.));
#19898=CARTESIAN_POINT('Ctrl Pts',(37.6615277218027,-15.3208746890781,0.));
#19899=CARTESIAN_POINT('Ctrl Pts',(37.7607947318286,-15.320070396385,0.));
#19900=CARTESIAN_POINT('Ctrl Pts',(37.8601926265378,-15.3186394335023,0.));
#19901=CARTESIAN_POINT('Ctrl Pts',(37.959716421934,-15.3165911656268,0.));
#19902=CARTESIAN_POINT('Ctrl Pts',(38.0593621055415,-15.3139321941687,0.));
#19903=CARTESIAN_POINT('Ctrl Pts',(38.1591262705847,-15.310667421514,0.));
#19904=CARTESIAN_POINT('Ctrl Pts',(38.2590058835965,-15.3068007250314,0.));
#19905=CARTESIAN_POINT('Ctrl Pts',(38.3589980188324,-15.3023357307483,0.));
#19906=CARTESIAN_POINT('Ctrl Pts',(38.4590995527814,-15.297276703747,0.));
#19907=CARTESIAN_POINT('Ctrl Pts',(38.5593070891769,-15.2916287700102,0.));
#19908=CARTESIAN_POINT('Ctrl Pts',(38.659617115053,-15.2853974668211,0.));
#19909=CARTESIAN_POINT('Ctrl Pts',(38.7600260961351,-15.2785884727112,0.));
#19910=CARTESIAN_POINT('Ctrl Pts',(38.860530586589,-15.2712072937639,0.));
#19911=CARTESIAN_POINT('Ctrl Pts',(38.9611273555758,-15.2632589109473,0.));
#19912=CARTESIAN_POINT('Ctrl Pts',(39.061813415425,-15.2547476855825,0.));
#19913=CARTESIAN_POINT('Ctrl Pts',(39.1625859371304,-15.2456775636447,0.));
#19914=CARTESIAN_POINT('Ctrl Pts',(39.2634421927888,-15.2360522089072,0.));
#19915=CARTESIAN_POINT('Ctrl Pts',(39.3643794927167,-15.225875156307,0.));
#19916=CARTESIAN_POINT('Ctrl Pts',(39.4653951093947,-15.2151499908149,0.));
#19917=CARTESIAN_POINT('Ctrl Pts',(39.5664862602472,-15.2038804098649,0.));
#19918=CARTESIAN_POINT('Ctrl Pts',(39.6676501731673,-15.1920701163804,0.));
#19919=CARTESIAN_POINT('Ctrl Pts',(39.7688841338802,-15.1797227547562,0.));
#19920=CARTESIAN_POINT('Ctrl Pts',(39.8701855339908,-15.1668418393198,0.));
#19921=CARTESIAN_POINT('Ctrl Pts',(39.9715519332134,-15.1534306754871,0.));
#19922=CARTESIAN_POINT('Ctrl Pts',(40.0729810652204,-15.1394923361537,0.));
#19923=CARTESIAN_POINT('Ctrl Pts',(40.1744707357902,-15.1250297462408,0.));
#19924=CARTESIAN_POINT('Ctrl Pts',(40.2760187401821,-15.1100457495259,0.));
#19925=CARTESIAN_POINT('Ctrl Pts',(40.3776227809037,-15.0945431800724,0.));
#19926=CARTESIAN_POINT('Ctrl Pts',(40.4792803645352,-15.0785249502524,0.));
#19927=CARTESIAN_POINT('Ctrl Pts',(40.58098877043,-15.0619940893017,0.));
#19928=CARTESIAN_POINT('Ctrl Pts',(40.6827452453667,-15.0449536183143,0.));
#19929=CARTESIAN_POINT('Ctrl Pts',(40.7845471608654,-15.0274064563211,0.));
#19930=CARTESIAN_POINT('Ctrl Pts',(40.8863921801,-15.0093553188655,0.));
#19931=CARTESIAN_POINT('Ctrl Pts',(40.9882784321884,-14.9908026205824,0.));
#19932=CARTESIAN_POINT('Ctrl Pts',(41.1105898934098,-14.9679399407908,0.));
#19933=CARTESIAN_POINT('Ctrl Pts',(41.2125650743922,-14.9482653093396,0.));
#19934=CARTESIAN_POINT('Ctrl Pts',(41.2941761025922,-14.9321285285561,0.));
#19935=CARTESIAN_POINT('Ctrl Pts',(41.3554017279611,-14.919802810928,0.));
#19936=CARTESIAN_POINT('Ctrl Pts',(41.396226524684,-14.911486495888,0.));
#19937=CARTESIAN_POINT('Ctrl Pts',(34.5082745737944,-14.9001523628048,15.));
#19938=CARTESIAN_POINT('Ctrl Pts',(34.525687510388,-14.9076710061311,15.));
#19939=CARTESIAN_POINT('Ctrl Pts',(34.5606858566713,-14.9222326355678,15.));
#19940=CARTESIAN_POINT('Ctrl Pts',(34.6137007885254,-14.9426481276593,15.));
#19941=CARTESIAN_POINT('Ctrl Pts',(34.6853717911268,-14.9671565602316,15.));
#19942=CARTESIAN_POINT('Ctrl Pts',(34.7763085406486,-14.9940927023322,15.));
#19943=CARTESIAN_POINT('Ctrl Pts',(34.8682205930809,-15.0183713484962,15.));
#19944=CARTESIAN_POINT('Ctrl Pts',(34.9607388363587,-15.041018569143,15.));
#19945=CARTESIAN_POINT('Ctrl Pts',(35.0535882932913,-15.0627878528202,15.));
#19946=CARTESIAN_POINT('Ctrl Pts',(35.1466591020976,-15.08395927165,15.));
#19947=CARTESIAN_POINT('Ctrl Pts',(35.2399506932815,-15.104500806927,15.));
#19948=CARTESIAN_POINT('Ctrl Pts',(35.3335286891314,-15.1241934020682,15.));
#19949=CARTESIAN_POINT('Ctrl Pts',(35.4274792115856,-15.1427632633831,15.));
#19950=CARTESIAN_POINT('Ctrl Pts',(35.5218591529745,-15.1600260710384,15.));
#19951=CARTESIAN_POINT('Ctrl Pts',(35.6166644736253,-15.1759785763051,15.));
#19952=CARTESIAN_POINT('Ctrl Pts',(35.7118553943773,-15.1907243629659,15.));
#19953=CARTESIAN_POINT('Ctrl Pts',(35.8073720252878,-15.2044274601769,15.));
#19954=CARTESIAN_POINT('Ctrl Pts',(35.9031525499277,-15.2172585668056,15.));
#19955=CARTESIAN_POINT('Ctrl Pts',(35.9991531408727,-15.2293360946131,15.));
#19956=CARTESIAN_POINT('Ctrl Pts',(36.095357546697,-15.240697754828,15.));
#19957=CARTESIAN_POINT('Ctrl Pts',(36.1917659216814,-15.2513334565427,15.));
#19958=CARTESIAN_POINT('Ctrl Pts',(36.2883880151607,-15.2612053303774,15.));
#19959=CARTESIAN_POINT('Ctrl Pts',(36.3852352131887,-15.2702711460937,15.));
#19960=CARTESIAN_POINT('Ctrl Pts',(36.4823116513289,-15.2785104654792,15.));
#19961=CARTESIAN_POINT('Ctrl Pts',(36.5796108931244,-15.2859343913094,15.));
#19962=CARTESIAN_POINT('Ctrl Pts',(36.6771206167755,-15.2925717100767,15.));
#19963=CARTESIAN_POINT('Ctrl Pts',(36.7748254044502,-15.2984606286738,15.));
#19964=CARTESIAN_POINT('Ctrl Pts',(36.8727100302512,-15.3036390436952,15.));
#19965=CARTESIAN_POINT('Ctrl Pts',(36.970763176802,-15.3081335446406,15.));
#19966=CARTESIAN_POINT('Ctrl Pts',(37.0689784837457,-15.3119562971444,15.));
#19967=CARTESIAN_POINT('Ctrl Pts',(37.1673525354641,-15.3151109648809,15.));
#19968=CARTESIAN_POINT('Ctrl Pts',(37.2658836214694,-15.3175963510698,15.));
#19969=CARTESIAN_POINT('Ctrl Pts',(37.3645702997848,-15.3194106233802,15.));
#19970=CARTESIAN_POINT('Ctrl Pts',(37.4634097578665,-15.3205561366169,15.));
#19971=CARTESIAN_POINT('Ctrl Pts',(37.562397408596,-15.3210406145546,15.));
#19972=CARTESIAN_POINT('Ctrl Pts',(37.6615277218027,-15.3208746890781,15.));
#19973=CARTESIAN_POINT('Ctrl Pts',(37.7607947318286,-15.320070396385,15.));
#19974=CARTESIAN_POINT('Ctrl Pts',(37.8601926265378,-15.3186394335023,15.));
#19975=CARTESIAN_POINT('Ctrl Pts',(37.959716421934,-15.3165911656268,15.));
#19976=CARTESIAN_POINT('Ctrl Pts',(38.0593621055415,-15.3139321941687,15.));
#19977=CARTESIAN_POINT('Ctrl Pts',(38.1591262705847,-15.310667421514,15.));
#19978=CARTESIAN_POINT('Ctrl Pts',(38.2590058835965,-15.3068007250314,15.));
#19979=CARTESIAN_POINT('Ctrl Pts',(38.3589980188324,-15.3023357307483,15.));
#19980=CARTESIAN_POINT('Ctrl Pts',(38.4590995527814,-15.297276703747,15.));
#19981=CARTESIAN_POINT('Ctrl Pts',(38.5593070891769,-15.2916287700102,15.));
#19982=CARTESIAN_POINT('Ctrl Pts',(38.659617115053,-15.2853974668211,15.));
#19983=CARTESIAN_POINT('Ctrl Pts',(38.7600260961351,-15.2785884727112,15.));
#19984=CARTESIAN_POINT('Ctrl Pts',(38.860530586589,-15.2712072937639,15.));
#19985=CARTESIAN_POINT('Ctrl Pts',(38.9611273555758,-15.2632589109473,15.));
#19986=CARTESIAN_POINT('Ctrl Pts',(39.061813415425,-15.2547476855825,15.));
#19987=CARTESIAN_POINT('Ctrl Pts',(39.1625859371304,-15.2456775636447,15.));
#19988=CARTESIAN_POINT('Ctrl Pts',(39.2634421927888,-15.2360522089072,15.));
#19989=CARTESIAN_POINT('Ctrl Pts',(39.3643794927167,-15.225875156307,15.));
#19990=CARTESIAN_POINT('Ctrl Pts',(39.4653951093947,-15.2151499908149,15.));
#19991=CARTESIAN_POINT('Ctrl Pts',(39.5664862602472,-15.2038804098649,15.));
#19992=CARTESIAN_POINT('Ctrl Pts',(39.6676501731673,-15.1920701163804,15.));
#19993=CARTESIAN_POINT('Ctrl Pts',(39.7688841338802,-15.1797227547562,15.));
#19994=CARTESIAN_POINT('Ctrl Pts',(39.8701855339908,-15.1668418393198,15.));
#19995=CARTESIAN_POINT('Ctrl Pts',(39.9715519332134,-15.1534306754871,15.));
#19996=CARTESIAN_POINT('Ctrl Pts',(40.0729810652204,-15.1394923361537,15.));
#19997=CARTESIAN_POINT('Ctrl Pts',(40.1744707357902,-15.1250297462408,15.));
#19998=CARTESIAN_POINT('Ctrl Pts',(40.2760187401821,-15.1100457495259,15.));
#19999=CARTESIAN_POINT('Ctrl Pts',(40.3776227809037,-15.0945431800724,15.));
#20000=CARTESIAN_POINT('Ctrl Pts',(40.4792803645352,-15.0785249502524,15.));
#20001=CARTESIAN_POINT('Ctrl Pts',(40.58098877043,-15.0619940893017,15.));
#20002=CARTESIAN_POINT('Ctrl Pts',(40.6827452453667,-15.0449536183143,15.));
#20003=CARTESIAN_POINT('Ctrl Pts',(40.7845471608654,-15.0274064563211,15.));
#20004=CARTESIAN_POINT('Ctrl Pts',(40.8863921801,-15.0093553188655,15.));
#20005=CARTESIAN_POINT('Ctrl Pts',(40.9882784321884,-14.9908026205824,15.));
#20006=CARTESIAN_POINT('Ctrl Pts',(41.1105898934098,-14.9679399407908,15.));
#20007=CARTESIAN_POINT('Ctrl Pts',(41.2125650743922,-14.9482653093396,15.));
#20008=CARTESIAN_POINT('Ctrl Pts',(41.2941761025922,-14.9321285285561,15.));
#20009=CARTESIAN_POINT('Ctrl Pts',(41.3554017279611,-14.919802810928,15.));
#20010=CARTESIAN_POINT('Ctrl Pts',(41.396226524684,-14.911486495888,15.));
#20011=CARTESIAN_POINT('Ctrl Pts',(36.3957374383337,-24.725498909423,0.));
#20012=CARTESIAN_POINT('Ctrl Pts',(36.3957374383337,-24.725498909423,18.));
#20013=CARTESIAN_POINT('Ctrl Pts',(36.3871033517098,-24.7065408286023,0.));
#20014=CARTESIAN_POINT('Ctrl Pts',(36.3871033517098,-24.7065408286023,18.));
#20015=CARTESIAN_POINT('Ctrl Pts',(36.369797330215,-24.6686569322616,0.));
#20016=CARTESIAN_POINT('Ctrl Pts',(36.369797330215,-24.6686569322616,18.));
#20017=CARTESIAN_POINT('Ctrl Pts',(36.3437247532368,-24.6119278836614,0.));
#20018=CARTESIAN_POINT('Ctrl Pts',(36.3437247532368,-24.6119278836614,18.));
#20019=CARTESIAN_POINT('Ctrl Pts',(36.3087341522969,-24.5364828082556,0.));
#20020=CARTESIAN_POINT('Ctrl Pts',(36.3087341522969,-24.5364828082556,18.));
#20021=CARTESIAN_POINT('Ctrl Pts',(36.2646168058395,-24.4424997853605,0.));
#20022=CARTESIAN_POINT('Ctrl Pts',(36.2646168058395,-24.4424997853605,18.));
#20023=CARTESIAN_POINT('Ctrl Pts',(36.2201196586696,-24.3488411214068,0.));
#20024=CARTESIAN_POINT('Ctrl Pts',(36.2201196586696,-24.3488411214068,18.));
#20025=CARTESIAN_POINT('Ctrl Pts',(36.1752418704833,-24.2555084095332,0.));
#20026=CARTESIAN_POINT('Ctrl Pts',(36.1752418704833,-24.2555084095332,18.));
#20027=CARTESIAN_POINT('Ctrl Pts',(36.1299825471271,-24.1625038657964,0.));
#20028=CARTESIAN_POINT('Ctrl Pts',(36.1299825471271,-24.1625038657964,18.));
#20029=CARTESIAN_POINT('Ctrl Pts',(36.0843408347974,-24.0698304230588,0.));
#20030=CARTESIAN_POINT('Ctrl Pts',(36.0843408347974,-24.0698304230588,18.));
#20031=CARTESIAN_POINT('Ctrl Pts',(36.0383159101253,-23.9774915680089,0.));
#20032=CARTESIAN_POINT('Ctrl Pts',(36.0383159101253,-23.9774915680089,18.));
#20033=CARTESIAN_POINT('Ctrl Pts',(35.9919069565469,-23.8854911428947,0.));
#20034=CARTESIAN_POINT('Ctrl Pts',(35.9919069565469,-23.8854911428947,18.));
#20035=CARTESIAN_POINT('Ctrl Pts',(35.9451131482488,-23.7938331508737,0.));
#20036=CARTESIAN_POINT('Ctrl Pts',(35.9451131482488,-23.7938331508737,18.));
#20037=CARTESIAN_POINT('Ctrl Pts',(35.8979336336837,-23.7025215735353,0.));
#20038=CARTESIAN_POINT('Ctrl Pts',(35.8979336336837,-23.7025215735353,18.));
#20039=CARTESIAN_POINT('Ctrl Pts',(35.8503675222884,-23.611560139948,0.));
#20040=CARTESIAN_POINT('Ctrl Pts',(35.8503675222884,-23.611560139948,18.));
#20041=CARTESIAN_POINT('Ctrl Pts',(35.8024138716896,-23.5209523746427,0.));
#20042=CARTESIAN_POINT('Ctrl Pts',(35.8024138716896,-23.5209523746427,18.));
#20043=CARTESIAN_POINT('Ctrl Pts',(35.7540716771372,-23.4307017328227,0.));
#20044=CARTESIAN_POINT('Ctrl Pts',(35.7540716771372,-23.4307017328227,18.));
#20045=CARTESIAN_POINT('Ctrl Pts',(35.7053398620512,-23.3408117088762,0.));
#20046=CARTESIAN_POINT('Ctrl Pts',(35.7053398620512,-23.3408117088762,18.));
#20047=CARTESIAN_POINT('Ctrl Pts',(35.6562172725207,-23.2512859425032,0.));
#20048=CARTESIAN_POINT('Ctrl Pts',(35.6562172725207,-23.2512859425032,18.));
#20049=CARTESIAN_POINT('Ctrl Pts',(35.6067026687722,-23.1621283508111,0.));
#20050=CARTESIAN_POINT('Ctrl Pts',(35.6067026687722,-23.1621283508111,18.));
#20051=CARTESIAN_POINT('Ctrl Pts',(35.5567947408311,-23.0733431097058,0.));
#20052=CARTESIAN_POINT('Ctrl Pts',(35.5567947408311,-23.0733431097058,18.));
#20053=CARTESIAN_POINT('Ctrl Pts',(35.5064921357308,-22.9849345572033,0.));
#20054=CARTESIAN_POINT('Ctrl Pts',(35.5064921357308,-22.9849345572033,18.));
#20055=CARTESIAN_POINT('Ctrl Pts',(35.4557934871468,-22.8969071125089,0.));
#20056=CARTESIAN_POINT('Ctrl Pts',(35.4557934871468,-22.8969071125089,18.));
#20057=CARTESIAN_POINT('Ctrl Pts',(35.4046974393492,-22.8092652000707,0.));
#20058=CARTESIAN_POINT('Ctrl Pts',(35.4046974393492,-22.8092652000707,18.));
#20059=CARTESIAN_POINT('Ctrl Pts',(35.3532026952313,-22.7220131336913,0.));
#20060=CARTESIAN_POINT('Ctrl Pts',(35.3532026952313,-22.7220131336913,18.));
#20061=CARTESIAN_POINT('Ctrl Pts',(35.3013079759252,-22.635155167154,0.));
#20062=CARTESIAN_POINT('Ctrl Pts',(35.3013079759252,-22.635155167154,18.));
#20063=CARTESIAN_POINT('Ctrl Pts',(35.2490119207975,-22.548695660891,0.));
#20064=CARTESIAN_POINT('Ctrl Pts',(35.2490119207975,-22.548695660891,18.));
#20065=CARTESIAN_POINT('Ctrl Pts',(35.1963130003352,-22.4626392230023,0.));
#20066=CARTESIAN_POINT('Ctrl Pts',(35.1963130003352,-22.4626392230023,18.));
#20067=CARTESIAN_POINT('Ctrl Pts',(35.1432094422642,-22.3769908340843,0.));
#20068=CARTESIAN_POINT('Ctrl Pts',(35.1432094422642,-22.3769908340843,18.));
#20069=CARTESIAN_POINT('Ctrl Pts',(35.0896991159359,-22.2917560356803,0.));
#20070=CARTESIAN_POINT('Ctrl Pts',(35.0896991159359,-22.2917560356803,18.));
#20071=CARTESIAN_POINT('Ctrl Pts',(35.0357795922459,-22.2069408519233,0.));
#20072=CARTESIAN_POINT('Ctrl Pts',(35.0357795922459,-22.2069408519233,18.));
#20073=CARTESIAN_POINT('Ctrl Pts',(34.9814483545602,-22.1225514798584,0.));
#20074=CARTESIAN_POINT('Ctrl Pts',(34.9814483545602,-22.1225514798584,18.));
#20075=CARTESIAN_POINT('Ctrl Pts',(34.9267029879922,-22.0385940162683,0.));
#20076=CARTESIAN_POINT('Ctrl Pts',(34.9267029879922,-22.0385940162683,18.));
#20077=CARTESIAN_POINT('Ctrl Pts',(34.8715413418101,-21.9550742217675,0.));
#20078=CARTESIAN_POINT('Ctrl Pts',(34.8715413418101,-21.9550742217675,18.));
#20079=CARTESIAN_POINT('Ctrl Pts',(34.8159618014436,-21.8719971302818,0.));
#20080=CARTESIAN_POINT('Ctrl Pts',(34.8159618014436,-21.8719971302818,18.));
#20081=CARTESIAN_POINT('Ctrl Pts',(34.7599631530844,-21.7893672401137,0.));
#20082=CARTESIAN_POINT('Ctrl Pts',(34.7599631530844,-21.7893672401137,18.));
#20083=CARTESIAN_POINT('Ctrl Pts',(34.7035440429025,-21.7071892844497,0.));
#20084=CARTESIAN_POINT('Ctrl Pts',(34.7035440429025,-21.7071892844497,18.));
#20085=CARTESIAN_POINT('Ctrl Pts',(34.6467025072367,-21.6254689009796,0.));
#20086=CARTESIAN_POINT('Ctrl Pts',(34.6467025072367,-21.6254689009796,18.));
#20087=CARTESIAN_POINT('Ctrl Pts',(34.5894355639082,-21.5442132160757,0.));
#20088=CARTESIAN_POINT('Ctrl Pts',(34.5894355639082,-21.5442132160757,18.));
#20089=CARTESIAN_POINT('Ctrl Pts',(34.5317385658329,-21.4634317666005,0.));
#20090=CARTESIAN_POINT('Ctrl Pts',(34.5317385658329,-21.4634317666005,18.));
#20091=CARTESIAN_POINT('Ctrl Pts',(34.4736054662052,-21.3831361300104,0.));
#20092=CARTESIAN_POINT('Ctrl Pts',(34.4736054662052,-21.3831361300104,18.));
#20093=CARTESIAN_POINT('Ctrl Pts',(34.4150300340623,-21.3033382073239,0.));
#20094=CARTESIAN_POINT('Ctrl Pts',(34.4150300340623,-21.3033382073239,18.));
#20095=CARTESIAN_POINT('Ctrl Pts',(34.3560069185815,-21.2240487218079,0.));
#20096=CARTESIAN_POINT('Ctrl Pts',(34.3560069185815,-21.2240487218079,18.));
#20097=CARTESIAN_POINT('Ctrl Pts',(34.2965325673384,-21.14527592444,0.));
#20098=CARTESIAN_POINT('Ctrl Pts',(34.2965325673384,-21.14527592444,18.));
#20099=CARTESIAN_POINT('Ctrl Pts',(34.2366067284279,-21.0670234747355,0.));
#20100=CARTESIAN_POINT('Ctrl Pts',(34.2366067284279,-21.0670234747355,18.));
#20101=CARTESIAN_POINT('Ctrl Pts',(34.176231731809,-20.9892914622612,0.));
#20102=CARTESIAN_POINT('Ctrl Pts',(34.176231731809,-20.9892914622612,18.));
#20103=CARTESIAN_POINT('Ctrl Pts',(34.1154095510973,-20.9120805673809,0.));
#20104=CARTESIAN_POINT('Ctrl Pts',(34.1154095510973,-20.9120805673809,18.));
#20105=CARTESIAN_POINT('Ctrl Pts',(34.0541392299678,-20.8353957068415,0.));
#20106=CARTESIAN_POINT('Ctrl Pts',(34.0541392299678,-20.8353957068415,18.));
#20107=CARTESIAN_POINT('Ctrl Pts',(33.9924146647395,-20.7592491770603,0.));
#20108=CARTESIAN_POINT('Ctrl Pts',(33.9924146647395,-20.7592491770603,18.));
#20109=CARTESIAN_POINT('Ctrl Pts',(33.9302209962425,-20.683665762903,0.));
#20110=CARTESIAN_POINT('Ctrl Pts',(33.9302209962425,-20.683665762903,18.));
#20111=CARTESIAN_POINT('Ctrl Pts',(33.8675365150454,-20.6086800574386,0.));
#20112=CARTESIAN_POINT('Ctrl Pts',(33.8675365150454,-20.6086800574386,18.));
#20113=CARTESIAN_POINT('Ctrl Pts',(33.8043393734971,-20.5343269914034,0.));
#20114=CARTESIAN_POINT('Ctrl Pts',(33.8043393734971,-20.5343269914034,18.));
#20115=CARTESIAN_POINT('Ctrl Pts',(33.7406135254082,-20.4606334536183,0.));
#20116=CARTESIAN_POINT('Ctrl Pts',(33.7406135254082,-20.4606334536183,18.));
#20117=CARTESIAN_POINT('Ctrl Pts',(33.6763537716992,-20.3876111773341,0.));
#20118=CARTESIAN_POINT('Ctrl Pts',(33.6763537716992,-20.3876111773341,18.));
#20119=CARTESIAN_POINT('Ctrl Pts',(33.6115742164079,-20.3152448035298,0.));
#20120=CARTESIAN_POINT('Ctrl Pts',(33.6115742164079,-20.3152448035298,18.));
#20121=CARTESIAN_POINT('Ctrl Pts',(33.5463023319603,-20.243500298383,0.));
#20122=CARTESIAN_POINT('Ctrl Pts',(33.5463023319603,-20.243500298383,18.));
#20123=CARTESIAN_POINT('Ctrl Pts',(33.480563024813,-20.1723475154533,0.));
#20124=CARTESIAN_POINT('Ctrl Pts',(33.480563024813,-20.1723475154533,18.));
#20125=CARTESIAN_POINT('Ctrl Pts',(33.4143643679979,-20.1017803986381,0.));
#20126=CARTESIAN_POINT('Ctrl Pts',(33.4143643679979,-20.1017803986381,18.));
#20127=CARTESIAN_POINT('Ctrl Pts',(33.3476854048385,-20.0318342617213,0.));
#20128=CARTESIAN_POINT('Ctrl Pts',(33.3476854048385,-20.0318342617213,18.));
#20129=CARTESIAN_POINT('Ctrl Pts',(33.2804560993213,-19.9626141625206,0.));
#20130=CARTESIAN_POINT('Ctrl Pts',(33.2804560993213,-19.9626141625206,18.));
#20131=CARTESIAN_POINT('Ctrl Pts',(33.2125746879471,-19.8942704458546,0.));
#20132=CARTESIAN_POINT('Ctrl Pts',(33.2125746879471,-19.8942704458546,18.));
#20133=CARTESIAN_POINT('Ctrl Pts',(33.1439436707661,-19.8269479776239,0.));
#20134=CARTESIAN_POINT('Ctrl Pts',(33.1439436707661,-19.8269479776239,18.));
#20135=CARTESIAN_POINT('Ctrl Pts',(33.0745026283418,-19.7607398248651,0.));
#20136=CARTESIAN_POINT('Ctrl Pts',(33.0745026283418,-19.7607398248651,18.));
#20137=CARTESIAN_POINT('Ctrl Pts',(33.004256563411,-19.6956473461873,0.));
#20138=CARTESIAN_POINT('Ctrl Pts',(33.004256563411,-19.6956473461873,18.));
#20139=CARTESIAN_POINT('Ctrl Pts',(32.9333211533788,-19.6315161742485,0.));
#20140=CARTESIAN_POINT('Ctrl Pts',(32.9333211533788,-19.6315161742485,18.));
#20141=CARTESIAN_POINT('Ctrl Pts',(32.8618672807884,-19.5681157030437,0.));
#20142=CARTESIAN_POINT('Ctrl Pts',(32.8618672807884,-19.5681157030437,18.));
#20143=CARTESIAN_POINT('Ctrl Pts',(32.7900335943248,-19.5052640847974,0.));
#20144=CARTESIAN_POINT('Ctrl Pts',(32.7900335943248,-19.5052640847974,18.));
#20145=CARTESIAN_POINT('Ctrl Pts',(32.7178463324062,-19.4429429601189,0.));
#20146=CARTESIAN_POINT('Ctrl Pts',(32.7178463324062,-19.4429429601189,18.));
#20147=CARTESIAN_POINT('Ctrl Pts',(32.6451434870609,-19.381405831319,0.));
#20148=CARTESIAN_POINT('Ctrl Pts',(32.6451434870609,-19.381405831319,18.));
#20149=CARTESIAN_POINT('Ctrl Pts',(32.5714771007861,-19.3213180490743,0.));
#20150=CARTESIAN_POINT('Ctrl Pts',(32.5714771007861,-19.3213180490743,18.));
#20151=CARTESIAN_POINT('Ctrl Pts',(32.4962340238036,-19.2635813403783,0.));
#20152=CARTESIAN_POINT('Ctrl Pts',(32.4962340238036,-19.2635813403783,18.));
#20153=CARTESIAN_POINT('Ctrl Pts',(32.4342791270009,-19.2200039764927,0.));
#20154=CARTESIAN_POINT('Ctrl Pts',(32.4342791270009,-19.2200039764927,18.));
#20155=CARTESIAN_POINT('Ctrl Pts',(32.3866012518553,-19.1891139208368,0.));
#20156=CARTESIAN_POINT('Ctrl Pts',(32.3866012518553,-19.1891139208368,18.));
#20157=CARTESIAN_POINT('Ctrl Pts',(32.3542491343753,-19.1693587749508,0.));
#20158=CARTESIAN_POINT('Ctrl Pts',(32.3542491343753,-19.1693587749508,18.));
#20159=CARTESIAN_POINT('Ctrl Pts',(32.3379313568208,-19.1596907609891,0.));
#20160=CARTESIAN_POINT('Ctrl Pts',(32.3379313568208,-19.1596907609891,18.));
#20161=CARTESIAN_POINT('',(36.3957374383337,-24.7254989094229,0.));
#20162=CARTESIAN_POINT('Ctrl Pts',(32.3379313568208,-19.1596907609891,0.));
#20163=CARTESIAN_POINT('Ctrl Pts',(32.3542491343753,-19.1693587749508,0.));
#20164=CARTESIAN_POINT('Ctrl Pts',(32.3866012518553,-19.1891139208368,0.));
#20165=CARTESIAN_POINT('Ctrl Pts',(32.4342791270009,-19.2200039764927,0.));
#20166=CARTESIAN_POINT('Ctrl Pts',(32.4962340238036,-19.2635813403783,0.));
#20167=CARTESIAN_POINT('Ctrl Pts',(32.5714771007861,-19.3213180490743,0.));
#20168=CARTESIAN_POINT('Ctrl Pts',(32.6451434870609,-19.381405831319,0.));
#20169=CARTESIAN_POINT('Ctrl Pts',(32.7178463324062,-19.4429429601189,0.));
#20170=CARTESIAN_POINT('Ctrl Pts',(32.7900335943248,-19.5052640847974,0.));
#20171=CARTESIAN_POINT('Ctrl Pts',(32.8618672807884,-19.5681157030437,0.));
#20172=CARTESIAN_POINT('Ctrl Pts',(32.9333211533788,-19.6315161742485,0.));
#20173=CARTESIAN_POINT('Ctrl Pts',(33.004256563411,-19.6956473461873,0.));
#20174=CARTESIAN_POINT('Ctrl Pts',(33.0745026283418,-19.7607398248651,0.));
#20175=CARTESIAN_POINT('Ctrl Pts',(33.1439436707661,-19.8269479776239,0.));
#20176=CARTESIAN_POINT('Ctrl Pts',(33.2125746879471,-19.8942704458546,0.));
#20177=CARTESIAN_POINT('Ctrl Pts',(33.2804560993213,-19.9626141625206,0.));
#20178=CARTESIAN_POINT('Ctrl Pts',(33.3476854048385,-20.0318342617213,0.));
#20179=CARTESIAN_POINT('Ctrl Pts',(33.4143643679979,-20.1017803986381,0.));
#20180=CARTESIAN_POINT('Ctrl Pts',(33.480563024813,-20.1723475154533,0.));
#20181=CARTESIAN_POINT('Ctrl Pts',(33.5463023319603,-20.243500298383,0.));
#20182=CARTESIAN_POINT('Ctrl Pts',(33.6115742164079,-20.3152448035298,0.));
#20183=CARTESIAN_POINT('Ctrl Pts',(33.6763537716992,-20.3876111773341,0.));
#20184=CARTESIAN_POINT('Ctrl Pts',(33.7406135254082,-20.4606334536183,0.));
#20185=CARTESIAN_POINT('Ctrl Pts',(33.8043393734971,-20.5343269914034,0.));
#20186=CARTESIAN_POINT('Ctrl Pts',(33.8675365150454,-20.6086800574386,0.));
#20187=CARTESIAN_POINT('Ctrl Pts',(33.9302209962425,-20.683665762903,0.));
#20188=CARTESIAN_POINT('Ctrl Pts',(33.9924146647395,-20.7592491770603,0.));
#20189=CARTESIAN_POINT('Ctrl Pts',(34.0541392299678,-20.8353957068415,0.));
#20190=CARTESIAN_POINT('Ctrl Pts',(34.1154095510973,-20.9120805673809,0.));
#20191=CARTESIAN_POINT('Ctrl Pts',(34.176231731809,-20.9892914622612,0.));
#20192=CARTESIAN_POINT('Ctrl Pts',(34.2366067284279,-21.0670234747355,0.));
#20193=CARTESIAN_POINT('Ctrl Pts',(34.2965325673384,-21.14527592444,0.));
#20194=CARTESIAN_POINT('Ctrl Pts',(34.3560069185815,-21.2240487218079,0.));
#20195=CARTESIAN_POINT('Ctrl Pts',(34.4150300340623,-21.3033382073239,0.));
#20196=CARTESIAN_POINT('Ctrl Pts',(34.4736054662052,-21.3831361300104,0.));
#20197=CARTESIAN_POINT('Ctrl Pts',(34.5317385658329,-21.4634317666005,0.));
#20198=CARTESIAN_POINT('Ctrl Pts',(34.5894355639082,-21.5442132160757,0.));
#20199=CARTESIAN_POINT('Ctrl Pts',(34.6467025072367,-21.6254689009796,0.));
#20200=CARTESIAN_POINT('Ctrl Pts',(34.7035440429025,-21.7071892844497,0.));
#20201=CARTESIAN_POINT('Ctrl Pts',(34.7599631530844,-21.7893672401137,0.));
#20202=CARTESIAN_POINT('Ctrl Pts',(34.8159618014436,-21.8719971302818,0.));
#20203=CARTESIAN_POINT('Ctrl Pts',(34.8715413418101,-21.9550742217675,0.));
#20204=CARTESIAN_POINT('Ctrl Pts',(34.9267029879922,-22.0385940162683,0.));
#20205=CARTESIAN_POINT('Ctrl Pts',(34.9814483545602,-22.1225514798584,0.));
#20206=CARTESIAN_POINT('Ctrl Pts',(35.0357795922459,-22.2069408519233,0.));
#20207=CARTESIAN_POINT('Ctrl Pts',(35.0896991159359,-22.2917560356803,0.));
#20208=CARTESIAN_POINT('Ctrl Pts',(35.1432094422642,-22.3769908340843,0.));
#20209=CARTESIAN_POINT('Ctrl Pts',(35.1963130003352,-22.4626392230023,0.));
#20210=CARTESIAN_POINT('Ctrl Pts',(35.2490119207975,-22.548695660891,0.));
#20211=CARTESIAN_POINT('Ctrl Pts',(35.3013079759252,-22.635155167154,0.));
#20212=CARTESIAN_POINT('Ctrl Pts',(35.3532026952313,-22.7220131336913,0.));
#20213=CARTESIAN_POINT('Ctrl Pts',(35.4046974393492,-22.8092652000707,0.));
#20214=CARTESIAN_POINT('Ctrl Pts',(35.4557934871468,-22.8969071125089,0.));
#20215=CARTESIAN_POINT('Ctrl Pts',(35.5064921357308,-22.9849345572033,0.));
#20216=CARTESIAN_POINT('Ctrl Pts',(35.5567947408311,-23.0733431097058,0.));
#20217=CARTESIAN_POINT('Ctrl Pts',(35.6067026687722,-23.1621283508111,0.));
#20218=CARTESIAN_POINT('Ctrl Pts',(35.6562172725207,-23.2512859425032,0.));
#20219=CARTESIAN_POINT('Ctrl Pts',(35.7053398620512,-23.3408117088762,0.));
#20220=CARTESIAN_POINT('Ctrl Pts',(35.7540716771372,-23.4307017328227,0.));
#20221=CARTESIAN_POINT('Ctrl Pts',(35.8024138716896,-23.5209523746427,0.));
#20222=CARTESIAN_POINT('Ctrl Pts',(35.8503675222884,-23.611560139948,0.));
#20223=CARTESIAN_POINT('Ctrl Pts',(35.8979336336837,-23.7025215735353,0.));
#20224=CARTESIAN_POINT('Ctrl Pts',(35.9451131482488,-23.7938331508737,0.));
#20225=CARTESIAN_POINT('Ctrl Pts',(35.9919069565469,-23.8854911428947,0.));
#20226=CARTESIAN_POINT('Ctrl Pts',(36.0383159101253,-23.9774915680089,0.));
#20227=CARTESIAN_POINT('Ctrl Pts',(36.0843408347974,-24.0698304230588,0.));
#20228=CARTESIAN_POINT('Ctrl Pts',(36.1299825471271,-24.1625038657964,0.));
#20229=CARTESIAN_POINT('Ctrl Pts',(36.1752418704833,-24.2555084095332,0.));
#20230=CARTESIAN_POINT('Ctrl Pts',(36.2201196586696,-24.3488411214068,0.));
#20231=CARTESIAN_POINT('Ctrl Pts',(36.2735162352735,-24.4612315181512,0.));
#20232=CARTESIAN_POINT('Ctrl Pts',(36.3175386315528,-24.5552956307817,0.));
#20233=CARTESIAN_POINT('Ctrl Pts',(36.3524534604648,-24.630805301288,0.));
#20234=CARTESIAN_POINT('Ctrl Pts',(36.3784692650901,-24.6875827477484,0.));
#20235=CARTESIAN_POINT('Ctrl Pts',(36.3957374383337,-24.725498909423,0.));
#20236=CARTESIAN_POINT('',(36.3957374383337,-24.7254989094229,15.));
#20237=CARTESIAN_POINT('Ctrl Pts',(36.3957374383337,-24.725498909423,15.));
#20238=CARTESIAN_POINT('Ctrl Pts',(36.3871033517098,-24.7065408286023,15.));
#20239=CARTESIAN_POINT('Ctrl Pts',(36.369797330215,-24.6686569322616,15.));
#20240=CARTESIAN_POINT('Ctrl Pts',(36.3437247532368,-24.6119278836614,15.));
#20241=CARTESIAN_POINT('Ctrl Pts',(36.3087341522969,-24.5364828082556,15.));
#20242=CARTESIAN_POINT('Ctrl Pts',(36.2646168058395,-24.4424997853605,15.));
#20243=CARTESIAN_POINT('Ctrl Pts',(36.2201196586696,-24.3488411214068,15.));
#20244=CARTESIAN_POINT('Ctrl Pts',(36.1752418704833,-24.2555084095332,15.));
#20245=CARTESIAN_POINT('Ctrl Pts',(36.1299825471271,-24.1625038657964,15.));
#20246=CARTESIAN_POINT('Ctrl Pts',(36.0843408347974,-24.0698304230588,15.));
#20247=CARTESIAN_POINT('Ctrl Pts',(36.0383159101253,-23.9774915680089,15.));
#20248=CARTESIAN_POINT('Ctrl Pts',(35.9919069565469,-23.8854911428947,15.));
#20249=CARTESIAN_POINT('Ctrl Pts',(35.9451131482488,-23.7938331508737,15.));
#20250=CARTESIAN_POINT('Ctrl Pts',(35.8979336336837,-23.7025215735353,15.));
#20251=CARTESIAN_POINT('Ctrl Pts',(35.8503675222884,-23.611560139948,15.));
#20252=CARTESIAN_POINT('Ctrl Pts',(35.8024138716896,-23.5209523746427,15.));
#20253=CARTESIAN_POINT('Ctrl Pts',(35.7540716771372,-23.4307017328227,15.));
#20254=CARTESIAN_POINT('Ctrl Pts',(35.7053398620512,-23.3408117088762,15.));
#20255=CARTESIAN_POINT('Ctrl Pts',(35.6562172725207,-23.2512859425032,15.));
#20256=CARTESIAN_POINT('Ctrl Pts',(35.6067026687722,-23.1621283508111,15.));
#20257=CARTESIAN_POINT('Ctrl Pts',(35.5567947408311,-23.0733431097058,15.));
#20258=CARTESIAN_POINT('Ctrl Pts',(35.5064921357308,-22.9849345572033,15.));
#20259=CARTESIAN_POINT('Ctrl Pts',(35.4557934871468,-22.8969071125089,15.));
#20260=CARTESIAN_POINT('Ctrl Pts',(35.4046974393492,-22.8092652000707,15.));
#20261=CARTESIAN_POINT('Ctrl Pts',(35.3532026952313,-22.7220131336913,15.));
#20262=CARTESIAN_POINT('Ctrl Pts',(35.3013079759252,-22.635155167154,15.));
#20263=CARTESIAN_POINT('Ctrl Pts',(35.2490119207975,-22.548695660891,15.));
#20264=CARTESIAN_POINT('Ctrl Pts',(35.1963130003352,-22.4626392230023,15.));
#20265=CARTESIAN_POINT('Ctrl Pts',(35.1432094422642,-22.3769908340843,15.));
#20266=CARTESIAN_POINT('Ctrl Pts',(35.0896991159359,-22.2917560356803,15.));
#20267=CARTESIAN_POINT('Ctrl Pts',(35.0357795922459,-22.2069408519233,15.));
#20268=CARTESIAN_POINT('Ctrl Pts',(34.9814483545602,-22.1225514798584,15.));
#20269=CARTESIAN_POINT('Ctrl Pts',(34.9267029879922,-22.0385940162683,15.));
#20270=CARTESIAN_POINT('Ctrl Pts',(34.8715413418101,-21.9550742217675,15.));
#20271=CARTESIAN_POINT('Ctrl Pts',(34.8159618014436,-21.8719971302818,15.));
#20272=CARTESIAN_POINT('Ctrl Pts',(34.7599631530844,-21.7893672401137,15.));
#20273=CARTESIAN_POINT('Ctrl Pts',(34.7035440429025,-21.7071892844497,15.));
#20274=CARTESIAN_POINT('Ctrl Pts',(34.6467025072367,-21.6254689009796,15.));
#20275=CARTESIAN_POINT('Ctrl Pts',(34.5894355639082,-21.5442132160757,15.));
#20276=CARTESIAN_POINT('Ctrl Pts',(34.5317385658329,-21.4634317666005,15.));
#20277=CARTESIAN_POINT('Ctrl Pts',(34.4736054662052,-21.3831361300104,15.));
#20278=CARTESIAN_POINT('Ctrl Pts',(34.4150300340623,-21.3033382073239,15.));
#20279=CARTESIAN_POINT('Ctrl Pts',(34.3560069185815,-21.2240487218079,15.));
#20280=CARTESIAN_POINT('Ctrl Pts',(34.2965325673384,-21.14527592444,15.));
#20281=CARTESIAN_POINT('Ctrl Pts',(34.2366067284279,-21.0670234747355,15.));
#20282=CARTESIAN_POINT('Ctrl Pts',(34.176231731809,-20.9892914622612,15.));
#20283=CARTESIAN_POINT('Ctrl Pts',(34.1154095510973,-20.9120805673809,15.));
#20284=CARTESIAN_POINT('Ctrl Pts',(34.0541392299678,-20.8353957068415,15.));
#20285=CARTESIAN_POINT('Ctrl Pts',(33.9924146647395,-20.7592491770603,15.));
#20286=CARTESIAN_POINT('Ctrl Pts',(33.9302209962425,-20.683665762903,15.));
#20287=CARTESIAN_POINT('Ctrl Pts',(33.8675365150454,-20.6086800574386,15.));
#20288=CARTESIAN_POINT('Ctrl Pts',(33.8043393734971,-20.5343269914034,15.));
#20289=CARTESIAN_POINT('Ctrl Pts',(33.7406135254082,-20.4606334536183,15.));
#20290=CARTESIAN_POINT('Ctrl Pts',(33.6763537716992,-20.3876111773341,15.));
#20291=CARTESIAN_POINT('Ctrl Pts',(33.6115742164079,-20.3152448035298,15.));
#20292=CARTESIAN_POINT('Ctrl Pts',(33.5463023319603,-20.243500298383,15.));
#20293=CARTESIAN_POINT('Ctrl Pts',(33.480563024813,-20.1723475154533,15.));
#20294=CARTESIAN_POINT('Ctrl Pts',(33.4143643679979,-20.1017803986381,15.));
#20295=CARTESIAN_POINT('Ctrl Pts',(33.3476854048385,-20.0318342617213,15.));
#20296=CARTESIAN_POINT('Ctrl Pts',(33.2804560993213,-19.9626141625206,15.));
#20297=CARTESIAN_POINT('Ctrl Pts',(33.2125746879471,-19.8942704458546,15.));
#20298=CARTESIAN_POINT('Ctrl Pts',(33.1439436707661,-19.8269479776239,15.));
#20299=CARTESIAN_POINT('Ctrl Pts',(33.0745026283418,-19.7607398248651,15.));
#20300=CARTESIAN_POINT('Ctrl Pts',(33.004256563411,-19.6956473461873,15.));
#20301=CARTESIAN_POINT('Ctrl Pts',(32.9333211533788,-19.6315161742485,15.));
#20302=CARTESIAN_POINT('Ctrl Pts',(32.8618672807884,-19.5681157030437,15.));
#20303=CARTESIAN_POINT('Ctrl Pts',(32.7900335943248,-19.5052640847974,15.));
#20304=CARTESIAN_POINT('Ctrl Pts',(32.7178463324062,-19.4429429601189,15.));
#20305=CARTESIAN_POINT('Ctrl Pts',(32.6451434870609,-19.381405831319,15.));
#20306=CARTESIAN_POINT('Ctrl Pts',(32.5714771007861,-19.3213180490743,15.));
#20307=CARTESIAN_POINT('Ctrl Pts',(32.4962340238036,-19.2635813403783,15.));
#20308=CARTESIAN_POINT('Ctrl Pts',(32.4342791270009,-19.2200039764927,15.));
#20309=CARTESIAN_POINT('Ctrl Pts',(32.3866012518553,-19.1891139208368,15.));
#20310=CARTESIAN_POINT('Ctrl Pts',(32.3542491343753,-19.1693587749508,15.));
#20311=CARTESIAN_POINT('Ctrl Pts',(32.3379313568208,-19.1596907609891,15.));
#20312=CARTESIAN_POINT('',(36.3957374383337,-24.7254989094229,0.));
#20313=CARTESIAN_POINT('Origin',(9.16871631793044E-12,-6.66146233219319E-12,
0.));
#20314=CARTESIAN_POINT('',(34.762248247709,-26.9738038986838,0.));
#20315=CARTESIAN_POINT('Origin',(9.16871631793044E-12,-6.66146233219319E-12,
0.));
#20316=CARTESIAN_POINT('',(34.762248247709,-26.9738038986838,15.));
#20317=CARTESIAN_POINT('Origin',(9.16871631793044E-12,-6.66146233219319E-12,
15.));
#20318=CARTESIAN_POINT('',(34.762248247709,-26.9738038986838,0.));
#20319=CARTESIAN_POINT('Ctrl Pts',(28.2149191006268,-24.8345302882955,0.));
#20320=CARTESIAN_POINT('Ctrl Pts',(28.2149191006268,-24.8345302882955,18.));
#20321=CARTESIAN_POINT('Ctrl Pts',(28.2291563988795,-24.8470618363541,0.));
#20322=CARTESIAN_POINT('Ctrl Pts',(28.2291563988795,-24.8470618363541,18.));
#20323=CARTESIAN_POINT('Ctrl Pts',(28.2579420132101,-24.8717258526943,0.));
#20324=CARTESIAN_POINT('Ctrl Pts',(28.2579420132101,-24.8717258526943,18.));
#20325=CARTESIAN_POINT('Ctrl Pts',(28.3020534756061,-24.9075246543798,0.));
#20326=CARTESIAN_POINT('Ctrl Pts',(28.3020534756061,-24.9075246543798,18.));
#20327=CARTESIAN_POINT('Ctrl Pts',(28.3626431274892,-24.9529811166897,0.));
#20328=CARTESIAN_POINT('Ctrl Pts',(28.3626431274892,-24.9529811166897,18.));
#20329=CARTESIAN_POINT('Ctrl Pts',(28.4408053900206,-25.0066999111736,0.));
#20330=CARTESIAN_POINT('Ctrl Pts',(28.4408053900206,-25.0066999111736,18.));
#20331=CARTESIAN_POINT('Ctrl Pts',(28.5207164321473,-25.0581926620043,0.));
#20332=CARTESIAN_POINT('Ctrl Pts',(28.5207164321473,-25.0581926620043,18.));
#20333=CARTESIAN_POINT('Ctrl Pts',(28.6017081342376,-25.108321158239,0.));
#20334=CARTESIAN_POINT('Ctrl Pts',(28.6017081342376,-25.108321158239,18.));
#20335=CARTESIAN_POINT('Ctrl Pts',(28.6832861366762,-25.1577170374459,0.));
#20336=CARTESIAN_POINT('Ctrl Pts',(28.6832861366762,-25.1577170374459,18.));
#20337=CARTESIAN_POINT('Ctrl Pts',(28.7652594076549,-25.2066127148845,0.));
#20338=CARTESIAN_POINT('Ctrl Pts',(28.7652594076549,-25.2066127148845,18.));
#20339=CARTESIAN_POINT('Ctrl Pts',(28.8476372998748,-25.2549775629725,0.));
#20340=CARTESIAN_POINT('Ctrl Pts',(28.8476372998748,-25.2549775629725,18.));
#20341=CARTESIAN_POINT('Ctrl Pts',(28.9305499160476,-25.3026235249214,0.));
#20342=CARTESIAN_POINT('Ctrl Pts',(28.9305499160476,-25.3026235249214,18.));
#20343=CARTESIAN_POINT('Ctrl Pts',(29.0141637699076,-25.3493168206005,0.));
#20344=CARTESIAN_POINT('Ctrl Pts',(29.0141637699076,-25.3493168206005,18.));
#20345=CARTESIAN_POINT('Ctrl Pts',(29.098589927237,-25.3948997321279,0.));
#20346=CARTESIAN_POINT('Ctrl Pts',(29.098589927237,-25.3948997321279,18.));
#20347=CARTESIAN_POINT('Ctrl Pts',(29.183825549991,-25.4393679214513,0.));
#20348=CARTESIAN_POINT('Ctrl Pts',(29.183825549991,-25.4393679214513,18.));
#20349=CARTESIAN_POINT('Ctrl Pts',(29.2698007967907,-25.4828076101654,0.));
#20350=CARTESIAN_POINT('Ctrl Pts',(29.2698007967907,-25.4828076101654,18.));
#20351=CARTESIAN_POINT('Ctrl Pts',(29.356408021119,-25.5253562922582,0.));
#20352=CARTESIAN_POINT('Ctrl Pts',(29.356408021119,-25.5253562922582,18.));
#20353=CARTESIAN_POINT('Ctrl Pts',(29.443535683207,-25.5671572096726,0.));
#20354=CARTESIAN_POINT('Ctrl Pts',(29.443535683207,-25.5671572096726,18.));
#20355=CARTESIAN_POINT('Ctrl Pts',(29.5311055094509,-25.6083094352667,0.));
#20356=CARTESIAN_POINT('Ctrl Pts',(29.5311055094509,-25.6083094352667,18.));
#20357=CARTESIAN_POINT('Ctrl Pts',(29.6190903904157,-25.6488438125835,0.));
#20358=CARTESIAN_POINT('Ctrl Pts',(29.6190903904157,-25.6488438125835,18.));
#20359=CARTESIAN_POINT('Ctrl Pts',(29.7074935910931,-25.6887507922749,0.));
#20360=CARTESIAN_POINT('Ctrl Pts',(29.7074935910931,-25.6887507922749,18.));
#20361=CARTESIAN_POINT('Ctrl Pts',(29.7963360859334,-25.7279973711305,0.));
#20362=CARTESIAN_POINT('Ctrl Pts',(29.7963360859334,-25.7279973711305,18.));
#20363=CARTESIAN_POINT('Ctrl Pts',(29.8856417535786,-25.7665469042913,0.));
#20364=CARTESIAN_POINT('Ctrl Pts',(29.8856417535786,-25.7665469042913,18.));
#20365=CARTESIAN_POINT('Ctrl Pts',(29.9754208429384,-25.8043812318215,0.));
#20366=CARTESIAN_POINT('Ctrl Pts',(29.9754208429384,-25.8043812318215,18.));
#20367=CARTESIAN_POINT('Ctrl Pts',(30.0656638016321,-25.8415089241134,0.));
#20368=CARTESIAN_POINT('Ctrl Pts',(30.0656638016321,-25.8415089241134,18.));
#20369=CARTESIAN_POINT('Ctrl Pts',(30.1563500154165,-25.8779535511028,0.));
#20370=CARTESIAN_POINT('Ctrl Pts',(30.1563500154165,-25.8779535511028,18.));
#20371=CARTESIAN_POINT('Ctrl Pts',(30.2474530144827,-25.9137466853317,0.));
#20372=CARTESIAN_POINT('Ctrl Pts',(30.2474530144827,-25.9137466853317,18.));
#20373=CARTESIAN_POINT('Ctrl Pts',(30.3389466074503,-25.9489196635424,0.));
#20374=CARTESIAN_POINT('Ctrl Pts',(30.3389466074503,-25.9489196635424,18.));
#20375=CARTESIAN_POINT('Ctrl Pts',(30.4308118142473,-25.9834942765902,0.));
#20376=CARTESIAN_POINT('Ctrl Pts',(30.4308118142473,-25.9834942765902,18.));
#20377=CARTESIAN_POINT('Ctrl Pts',(30.5230388264271,-26.0174801292225,0.));
#20378=CARTESIAN_POINT('Ctrl Pts',(30.5230388264271,-26.0174801292225,18.));
#20379=CARTESIAN_POINT('Ctrl Pts',(30.6156232634061,-26.0508796503166,0.));
#20380=CARTESIAN_POINT('Ctrl Pts',(30.6156232634061,-26.0508796503166,18.));
#20381=CARTESIAN_POINT('Ctrl Pts',(30.7085638682391,-26.0836911730968,0.));
#20382=CARTESIAN_POINT('Ctrl Pts',(30.7085638682391,-26.0836911730968,18.));
#20383=CARTESIAN_POINT('Ctrl Pts',(30.8018598357461,-26.1159125093178,0.));
#20384=CARTESIAN_POINT('Ctrl Pts',(30.8018598357461,-26.1159125093178,18.));
#20385=CARTESIAN_POINT('Ctrl Pts',(30.8955077633644,-26.1475450294082,0.));
#20386=CARTESIAN_POINT('Ctrl Pts',(30.8955077633644,-26.1475450294082,18.));
#20387=CARTESIAN_POINT('Ctrl Pts',(30.9895009017072,-26.1785946616165,0.));
#20388=CARTESIAN_POINT('Ctrl Pts',(30.9895009017072,-26.1785946616165,18.));
#20389=CARTESIAN_POINT('Ctrl Pts',(31.0838307058369,-26.2090698085494,0.));
#20390=CARTESIAN_POINT('Ctrl Pts',(31.0838307058369,-26.2090698085494,18.));
#20391=CARTESIAN_POINT('Ctrl Pts',(31.1784877826858,-26.2389800738215,0.));
#20392=CARTESIAN_POINT('Ctrl Pts',(31.1784877826858,-26.2389800738215,18.));
#20393=CARTESIAN_POINT('Ctrl Pts',(31.2734629900041,-26.2683347859175,0.));
#20394=CARTESIAN_POINT('Ctrl Pts',(31.2734629900041,-26.2683347859175,18.));
#20395=CARTESIAN_POINT('Ctrl Pts',(31.3687486937246,-26.2971413115295,0.));
#20396=CARTESIAN_POINT('Ctrl Pts',(31.3687486937246,-26.2971413115295,18.));
#20397=CARTESIAN_POINT('Ctrl Pts',(31.4643390378083,-26.3254046890485,0.));
#20398=CARTESIAN_POINT('Ctrl Pts',(31.4643390378083,-26.3254046890485,18.));
#20399=CARTESIAN_POINT('Ctrl Pts',(31.5602292672984,-26.353128528169,0.));
#20400=CARTESIAN_POINT('Ctrl Pts',(31.5602292672984,-26.353128528169,18.));
#20401=CARTESIAN_POINT('Ctrl Pts',(31.6564152990236,-26.3803155790949,0.));
#20402=CARTESIAN_POINT('Ctrl Pts',(31.6564152990236,-26.3803155790949,18.));
#20403=CARTESIAN_POINT('Ctrl Pts',(31.7528932299312,-26.4069683862785,0.));
#20404=CARTESIAN_POINT('Ctrl Pts',(31.7528932299312,-26.4069683862785,18.));
#20405=CARTESIAN_POINT('Ctrl Pts',(31.849658771403,-26.433090040836,0.));
#20406=CARTESIAN_POINT('Ctrl Pts',(31.849658771403,-26.433090040836,18.));
#20407=CARTESIAN_POINT('Ctrl Pts',(31.9467071093816,-26.4586843683627,0.));
#20408=CARTESIAN_POINT('Ctrl Pts',(31.9467071093816,-26.4586843683627,18.));
#20409=CARTESIAN_POINT('Ctrl Pts',(32.0440331917233,-26.4837555495616,0.));
#20410=CARTESIAN_POINT('Ctrl Pts',(32.0440331917233,-26.4837555495616,18.));
#20411=CARTESIAN_POINT('Ctrl Pts',(32.1416319023705,-26.5083078928862,0.));
#20412=CARTESIAN_POINT('Ctrl Pts',(32.1416319023705,-26.5083078928862,18.));
#20413=CARTESIAN_POINT('Ctrl Pts',(32.2394982626669,-26.5323455701117,0.));
#20414=CARTESIAN_POINT('Ctrl Pts',(32.2394982626669,-26.5323455701117,18.));
#20415=CARTESIAN_POINT('Ctrl Pts',(32.3376276606981,-26.5558723200361,0.));
#20416=CARTESIAN_POINT('Ctrl Pts',(32.3376276606981,-26.5558723200361,18.));
#20417=CARTESIAN_POINT('Ctrl Pts',(32.4360159072985,-26.5788913672813,0.));
#20418=CARTESIAN_POINT('Ctrl Pts',(32.4360159072985,-26.5788913672813,18.));
#20419=CARTESIAN_POINT('Ctrl Pts',(32.5346590925498,-26.6014055904817,0.));
#20420=CARTESIAN_POINT('Ctrl Pts',(32.5346590925498,-26.6014055904817,18.));
#20421=CARTESIAN_POINT('Ctrl Pts',(32.6335534898935,-26.6234176311245,0.));
#20422=CARTESIAN_POINT('Ctrl Pts',(32.6335534898935,-26.6234176311245,18.));
#20423=CARTESIAN_POINT('Ctrl Pts',(32.7326954489334,-26.6449300199764,0.));
#20424=CARTESIAN_POINT('Ctrl Pts',(32.7326954489334,-26.6449300199764,18.));
#20425=CARTESIAN_POINT('Ctrl Pts',(32.8320812678271,-26.6659453236976,0.));
#20426=CARTESIAN_POINT('Ctrl Pts',(32.8320812678271,-26.6659453236976,18.));
#20427=CARTESIAN_POINT('Ctrl Pts',(32.9317071576181,-26.6864661988935,0.));
#20428=CARTESIAN_POINT('Ctrl Pts',(32.9317071576181,-26.6864661988935,18.));
#20429=CARTESIAN_POINT('Ctrl Pts',(33.03156933761,-26.7064953106254,0.));
#20430=CARTESIAN_POINT('Ctrl Pts',(33.03156933761,-26.7064953106254,18.));
#20431=CARTESIAN_POINT('Ctrl Pts',(33.131664100194,-26.7260352861619,0.));
#20432=CARTESIAN_POINT('Ctrl Pts',(33.131664100194,-26.7260352861619,18.));
#20433=CARTESIAN_POINT('Ctrl Pts',(33.2319878786519,-26.7450886617884,0.));
#20434=CARTESIAN_POINT('Ctrl Pts',(33.2319878786519,-26.7450886617884,18.));
#20435=CARTESIAN_POINT('Ctrl Pts',(33.3325373307046,-26.7636578270526,0.));
#20436=CARTESIAN_POINT('Ctrl Pts',(33.3325373307046,-26.7636578270526,18.));
#20437=CARTESIAN_POINT('Ctrl Pts',(33.4333093513694,-26.7817450041181,0.));
#20438=CARTESIAN_POINT('Ctrl Pts',(33.4333093513694,-26.7817450041181,18.));
#20439=CARTESIAN_POINT('Ctrl Pts',(33.5343009499673,-26.7993522966985,0.));
#20440=CARTESIAN_POINT('Ctrl Pts',(33.5343009499673,-26.7993522966985,18.));
#20441=CARTESIAN_POINT('Ctrl Pts',(33.6355091508895,-26.8164817280846,0.));
#20442=CARTESIAN_POINT('Ctrl Pts',(33.6355091508895,-26.8164817280846,18.));
#20443=CARTESIAN_POINT('Ctrl Pts',(33.7369308933173,-26.8331352836667,0.));
#20444=CARTESIAN_POINT('Ctrl Pts',(33.7369308933173,-26.8331352836667,18.));
#20445=CARTESIAN_POINT('Ctrl Pts',(33.838562905895,-26.8493149627661,0.));
#20446=CARTESIAN_POINT('Ctrl Pts',(33.838562905895,-26.8493149627661,18.));
#20447=CARTESIAN_POINT('Ctrl Pts',(33.9404016650487,-26.8650228056313,0.));
#20448=CARTESIAN_POINT('Ctrl Pts',(33.9404016650487,-26.8650228056313,18.));
#20449=CARTESIAN_POINT('Ctrl Pts',(34.0424436187397,-26.880260834701,0.));
#20450=CARTESIAN_POINT('Ctrl Pts',(34.0424436187397,-26.880260834701,18.));
#20451=CARTESIAN_POINT('Ctrl Pts',(34.1446853651051,-26.895031013894,0.));
#20452=CARTESIAN_POINT('Ctrl Pts',(34.1446853651051,-26.895031013894,18.));
#20453=CARTESIAN_POINT('Ctrl Pts',(34.2471238425419,-26.9093352037262,0.));
#20454=CARTESIAN_POINT('Ctrl Pts',(34.2471238425419,-26.9093352037262,18.));
#20455=CARTESIAN_POINT('Ctrl Pts',(34.3497565255724,-26.9231751225177,0.));
#20456=CARTESIAN_POINT('Ctrl Pts',(34.3497565255724,-26.9231751225177,18.));
#20457=CARTESIAN_POINT('Ctrl Pts',(34.4525815829097,-26.9365523054581,0.));
#20458=CARTESIAN_POINT('Ctrl Pts',(34.4525815829097,-26.9365523054581,18.));
#20459=CARTESIAN_POINT('Ctrl Pts',(34.5555977590573,-26.9494680440307,0.));
#20460=CARTESIAN_POINT('Ctrl Pts',(34.5555977590573,-26.9494680440307,18.));
#20461=CARTESIAN_POINT('Ctrl Pts',(34.6381629799782,-26.9594322726214,0.));
#20462=CARTESIAN_POINT('Ctrl Pts',(34.6381629799782,-26.9594322726214,18.));
#20463=CARTESIAN_POINT('Ctrl Pts',(34.700172380686,-26.9666985267609,0.));
#20464=CARTESIAN_POINT('Ctrl Pts',(34.700172380686,-26.9666985267609,18.));
#20465=CARTESIAN_POINT('Ctrl Pts',(34.7415499619104,-26.9714507634923,0.));
#20466=CARTESIAN_POINT('Ctrl Pts',(34.7415499619104,-26.9714507634923,18.));
#20467=CARTESIAN_POINT('Ctrl Pts',(34.7622482477091,-26.9738038986838,0.));
#20468=CARTESIAN_POINT('Ctrl Pts',(34.7622482477091,-26.9738038986838,18.));
#20469=CARTESIAN_POINT('Ctrl Pts',(28.2149191006268,-24.8345302882955,0.));
#20470=CARTESIAN_POINT('Ctrl Pts',(28.2291563988795,-24.8470618363541,0.));
#20471=CARTESIAN_POINT('Ctrl Pts',(28.2579420132101,-24.8717258526943,0.));
#20472=CARTESIAN_POINT('Ctrl Pts',(28.3020534756061,-24.9075246543798,0.));
#20473=CARTESIAN_POINT('Ctrl Pts',(28.3626431274892,-24.9529811166897,0.));
#20474=CARTESIAN_POINT('Ctrl Pts',(28.4408053900206,-25.0066999111736,0.));
#20475=CARTESIAN_POINT('Ctrl Pts',(28.5207164321473,-25.0581926620043,0.));
#20476=CARTESIAN_POINT('Ctrl Pts',(28.6017081342376,-25.108321158239,0.));
#20477=CARTESIAN_POINT('Ctrl Pts',(28.6832861366762,-25.1577170374459,0.));
#20478=CARTESIAN_POINT('Ctrl Pts',(28.7652594076549,-25.2066127148845,0.));
#20479=CARTESIAN_POINT('Ctrl Pts',(28.8476372998748,-25.2549775629725,0.));
#20480=CARTESIAN_POINT('Ctrl Pts',(28.9305499160476,-25.3026235249214,0.));
#20481=CARTESIAN_POINT('Ctrl Pts',(29.0141637699076,-25.3493168206005,0.));
#20482=CARTESIAN_POINT('Ctrl Pts',(29.098589927237,-25.3948997321279,0.));
#20483=CARTESIAN_POINT('Ctrl Pts',(29.183825549991,-25.4393679214513,0.));
#20484=CARTESIAN_POINT('Ctrl Pts',(29.2698007967907,-25.4828076101654,0.));
#20485=CARTESIAN_POINT('Ctrl Pts',(29.356408021119,-25.5253562922582,0.));
#20486=CARTESIAN_POINT('Ctrl Pts',(29.443535683207,-25.5671572096726,0.));
#20487=CARTESIAN_POINT('Ctrl Pts',(29.5311055094509,-25.6083094352667,0.));
#20488=CARTESIAN_POINT('Ctrl Pts',(29.6190903904157,-25.6488438125835,0.));
#20489=CARTESIAN_POINT('Ctrl Pts',(29.7074935910931,-25.6887507922749,0.));
#20490=CARTESIAN_POINT('Ctrl Pts',(29.7963360859334,-25.7279973711305,0.));
#20491=CARTESIAN_POINT('Ctrl Pts',(29.8856417535786,-25.7665469042913,0.));
#20492=CARTESIAN_POINT('Ctrl Pts',(29.9754208429384,-25.8043812318215,0.));
#20493=CARTESIAN_POINT('Ctrl Pts',(30.0656638016321,-25.8415089241134,0.));
#20494=CARTESIAN_POINT('Ctrl Pts',(30.1563500154165,-25.8779535511028,0.));
#20495=CARTESIAN_POINT('Ctrl Pts',(30.2474530144827,-25.9137466853317,0.));
#20496=CARTESIAN_POINT('Ctrl Pts',(30.3389466074503,-25.9489196635424,0.));
#20497=CARTESIAN_POINT('Ctrl Pts',(30.4308118142473,-25.9834942765902,0.));
#20498=CARTESIAN_POINT('Ctrl Pts',(30.5230388264271,-26.0174801292225,0.));
#20499=CARTESIAN_POINT('Ctrl Pts',(30.6156232634061,-26.0508796503166,0.));
#20500=CARTESIAN_POINT('Ctrl Pts',(30.7085638682391,-26.0836911730968,0.));
#20501=CARTESIAN_POINT('Ctrl Pts',(30.8018598357461,-26.1159125093178,0.));
#20502=CARTESIAN_POINT('Ctrl Pts',(30.8955077633644,-26.1475450294082,0.));
#20503=CARTESIAN_POINT('Ctrl Pts',(30.9895009017072,-26.1785946616165,0.));
#20504=CARTESIAN_POINT('Ctrl Pts',(31.0838307058369,-26.2090698085494,0.));
#20505=CARTESIAN_POINT('Ctrl Pts',(31.1784877826858,-26.2389800738215,0.));
#20506=CARTESIAN_POINT('Ctrl Pts',(31.2734629900041,-26.2683347859175,0.));
#20507=CARTESIAN_POINT('Ctrl Pts',(31.3687486937246,-26.2971413115295,0.));
#20508=CARTESIAN_POINT('Ctrl Pts',(31.4643390378083,-26.3254046890485,0.));
#20509=CARTESIAN_POINT('Ctrl Pts',(31.5602292672984,-26.353128528169,0.));
#20510=CARTESIAN_POINT('Ctrl Pts',(31.6564152990236,-26.3803155790949,0.));
#20511=CARTESIAN_POINT('Ctrl Pts',(31.7528932299312,-26.4069683862785,0.));
#20512=CARTESIAN_POINT('Ctrl Pts',(31.849658771403,-26.433090040836,0.));
#20513=CARTESIAN_POINT('Ctrl Pts',(31.9467071093816,-26.4586843683627,0.));
#20514=CARTESIAN_POINT('Ctrl Pts',(32.0440331917233,-26.4837555495616,0.));
#20515=CARTESIAN_POINT('Ctrl Pts',(32.1416319023705,-26.5083078928862,0.));
#20516=CARTESIAN_POINT('Ctrl Pts',(32.2394982626669,-26.5323455701117,0.));
#20517=CARTESIAN_POINT('Ctrl Pts',(32.3376276606981,-26.5558723200361,0.));
#20518=CARTESIAN_POINT('Ctrl Pts',(32.4360159072985,-26.5788913672813,0.));
#20519=CARTESIAN_POINT('Ctrl Pts',(32.5346590925498,-26.6014055904817,0.));
#20520=CARTESIAN_POINT('Ctrl Pts',(32.6335534898935,-26.6234176311245,0.));
#20521=CARTESIAN_POINT('Ctrl Pts',(32.7326954489334,-26.6449300199764,0.));
#20522=CARTESIAN_POINT('Ctrl Pts',(32.8320812678271,-26.6659453236976,0.));
#20523=CARTESIAN_POINT('Ctrl Pts',(32.9317071576181,-26.6864661988935,0.));
#20524=CARTESIAN_POINT('Ctrl Pts',(33.03156933761,-26.7064953106254,0.));
#20525=CARTESIAN_POINT('Ctrl Pts',(33.131664100194,-26.7260352861619,0.));
#20526=CARTESIAN_POINT('Ctrl Pts',(33.2319878786519,-26.7450886617884,0.));
#20527=CARTESIAN_POINT('Ctrl Pts',(33.3325373307046,-26.7636578270526,0.));
#20528=CARTESIAN_POINT('Ctrl Pts',(33.4333093513694,-26.7817450041181,0.));
#20529=CARTESIAN_POINT('Ctrl Pts',(33.5343009499673,-26.7993522966985,0.));
#20530=CARTESIAN_POINT('Ctrl Pts',(33.6355091508895,-26.8164817280846,0.));
#20531=CARTESIAN_POINT('Ctrl Pts',(33.7369308933173,-26.8331352836667,0.));
#20532=CARTESIAN_POINT('Ctrl Pts',(33.838562905895,-26.8493149627661,0.));
#20533=CARTESIAN_POINT('Ctrl Pts',(33.9404016650487,-26.8650228056313,0.));
#20534=CARTESIAN_POINT('Ctrl Pts',(34.0424436187397,-26.880260834701,0.));
#20535=CARTESIAN_POINT('Ctrl Pts',(34.1446853651051,-26.895031013894,0.));
#20536=CARTESIAN_POINT('Ctrl Pts',(34.2471238425419,-26.9093352037262,0.));
#20537=CARTESIAN_POINT('Ctrl Pts',(34.3497565255724,-26.9231751225177,0.));
#20538=CARTESIAN_POINT('Ctrl Pts',(34.4731465943772,-26.9392277420462,0.));
#20539=CARTESIAN_POINT('Ctrl Pts',(34.5762105502273,-26.9520281195268,0.));
#20540=CARTESIAN_POINT('Ctrl Pts',(34.6588137898952,-26.9619003236529,0.));
#20541=CARTESIAN_POINT('Ctrl Pts',(34.7208516760814,-26.9690976283149,0.));
#20542=CARTESIAN_POINT('Ctrl Pts',(34.7622482477091,-26.9738038986838,0.));
#20543=CARTESIAN_POINT('Ctrl Pts',(28.2149191006268,-24.8345302882955,15.));
#20544=CARTESIAN_POINT('Ctrl Pts',(28.2291563988795,-24.8470618363541,15.));
#20545=CARTESIAN_POINT('Ctrl Pts',(28.2579420132101,-24.8717258526943,15.));
#20546=CARTESIAN_POINT('Ctrl Pts',(28.3020534756061,-24.9075246543798,15.));
#20547=CARTESIAN_POINT('Ctrl Pts',(28.3626431274892,-24.9529811166897,15.));
#20548=CARTESIAN_POINT('Ctrl Pts',(28.4408053900206,-25.0066999111736,15.));
#20549=CARTESIAN_POINT('Ctrl Pts',(28.5207164321473,-25.0581926620043,15.));
#20550=CARTESIAN_POINT('Ctrl Pts',(28.6017081342376,-25.108321158239,15.));
#20551=CARTESIAN_POINT('Ctrl Pts',(28.6832861366762,-25.1577170374459,15.));
#20552=CARTESIAN_POINT('Ctrl Pts',(28.7652594076549,-25.2066127148845,15.));
#20553=CARTESIAN_POINT('Ctrl Pts',(28.8476372998748,-25.2549775629725,15.));
#20554=CARTESIAN_POINT('Ctrl Pts',(28.9305499160476,-25.3026235249214,15.));
#20555=CARTESIAN_POINT('Ctrl Pts',(29.0141637699076,-25.3493168206005,15.));
#20556=CARTESIAN_POINT('Ctrl Pts',(29.098589927237,-25.3948997321279,15.));
#20557=CARTESIAN_POINT('Ctrl Pts',(29.183825549991,-25.4393679214513,15.));
#20558=CARTESIAN_POINT('Ctrl Pts',(29.2698007967907,-25.4828076101654,15.));
#20559=CARTESIAN_POINT('Ctrl Pts',(29.356408021119,-25.5253562922582,15.));
#20560=CARTESIAN_POINT('Ctrl Pts',(29.443535683207,-25.5671572096726,15.));
#20561=CARTESIAN_POINT('Ctrl Pts',(29.5311055094509,-25.6083094352667,15.));
#20562=CARTESIAN_POINT('Ctrl Pts',(29.6190903904157,-25.6488438125835,15.));
#20563=CARTESIAN_POINT('Ctrl Pts',(29.7074935910931,-25.6887507922749,15.));
#20564=CARTESIAN_POINT('Ctrl Pts',(29.7963360859334,-25.7279973711305,15.));
#20565=CARTESIAN_POINT('Ctrl Pts',(29.8856417535786,-25.7665469042913,15.));
#20566=CARTESIAN_POINT('Ctrl Pts',(29.9754208429384,-25.8043812318215,15.));
#20567=CARTESIAN_POINT('Ctrl Pts',(30.0656638016321,-25.8415089241134,15.));
#20568=CARTESIAN_POINT('Ctrl Pts',(30.1563500154165,-25.8779535511028,15.));
#20569=CARTESIAN_POINT('Ctrl Pts',(30.2474530144827,-25.9137466853317,15.));
#20570=CARTESIAN_POINT('Ctrl Pts',(30.3389466074503,-25.9489196635424,15.));
#20571=CARTESIAN_POINT('Ctrl Pts',(30.4308118142473,-25.9834942765902,15.));
#20572=CARTESIAN_POINT('Ctrl Pts',(30.5230388264271,-26.0174801292225,15.));
#20573=CARTESIAN_POINT('Ctrl Pts',(30.6156232634061,-26.0508796503166,15.));
#20574=CARTESIAN_POINT('Ctrl Pts',(30.7085638682391,-26.0836911730968,15.));
#20575=CARTESIAN_POINT('Ctrl Pts',(30.8018598357461,-26.1159125093178,15.));
#20576=CARTESIAN_POINT('Ctrl Pts',(30.8955077633644,-26.1475450294082,15.));
#20577=CARTESIAN_POINT('Ctrl Pts',(30.9895009017072,-26.1785946616165,15.));
#20578=CARTESIAN_POINT('Ctrl Pts',(31.0838307058369,-26.2090698085494,15.));
#20579=CARTESIAN_POINT('Ctrl Pts',(31.1784877826858,-26.2389800738215,15.));
#20580=CARTESIAN_POINT('Ctrl Pts',(31.2734629900041,-26.2683347859175,15.));
#20581=CARTESIAN_POINT('Ctrl Pts',(31.3687486937246,-26.2971413115295,15.));
#20582=CARTESIAN_POINT('Ctrl Pts',(31.4643390378083,-26.3254046890485,15.));
#20583=CARTESIAN_POINT('Ctrl Pts',(31.5602292672984,-26.353128528169,15.));
#20584=CARTESIAN_POINT('Ctrl Pts',(31.6564152990236,-26.3803155790949,15.));
#20585=CARTESIAN_POINT('Ctrl Pts',(31.7528932299312,-26.4069683862785,15.));
#20586=CARTESIAN_POINT('Ctrl Pts',(31.849658771403,-26.433090040836,15.));
#20587=CARTESIAN_POINT('Ctrl Pts',(31.9467071093816,-26.4586843683627,15.));
#20588=CARTESIAN_POINT('Ctrl Pts',(32.0440331917233,-26.4837555495616,15.));
#20589=CARTESIAN_POINT('Ctrl Pts',(32.1416319023705,-26.5083078928862,15.));
#20590=CARTESIAN_POINT('Ctrl Pts',(32.2394982626669,-26.5323455701117,15.));
#20591=CARTESIAN_POINT('Ctrl Pts',(32.3376276606981,-26.5558723200361,15.));
#20592=CARTESIAN_POINT('Ctrl Pts',(32.4360159072985,-26.5788913672813,15.));
#20593=CARTESIAN_POINT('Ctrl Pts',(32.5346590925498,-26.6014055904817,15.));
#20594=CARTESIAN_POINT('Ctrl Pts',(32.6335534898935,-26.6234176311245,15.));
#20595=CARTESIAN_POINT('Ctrl Pts',(32.7326954489334,-26.6449300199764,15.));
#20596=CARTESIAN_POINT('Ctrl Pts',(32.8320812678271,-26.6659453236976,15.));
#20597=CARTESIAN_POINT('Ctrl Pts',(32.9317071576181,-26.6864661988935,15.));
#20598=CARTESIAN_POINT('Ctrl Pts',(33.03156933761,-26.7064953106254,15.));
#20599=CARTESIAN_POINT('Ctrl Pts',(33.131664100194,-26.7260352861619,15.));
#20600=CARTESIAN_POINT('Ctrl Pts',(33.2319878786519,-26.7450886617884,15.));
#20601=CARTESIAN_POINT('Ctrl Pts',(33.3325373307046,-26.7636578270526,15.));
#20602=CARTESIAN_POINT('Ctrl Pts',(33.4333093513694,-26.7817450041181,15.));
#20603=CARTESIAN_POINT('Ctrl Pts',(33.5343009499673,-26.7993522966985,15.));
#20604=CARTESIAN_POINT('Ctrl Pts',(33.6355091508895,-26.8164817280846,15.));
#20605=CARTESIAN_POINT('Ctrl Pts',(33.7369308933173,-26.8331352836667,15.));
#20606=CARTESIAN_POINT('Ctrl Pts',(33.838562905895,-26.8493149627661,15.));
#20607=CARTESIAN_POINT('Ctrl Pts',(33.9404016650487,-26.8650228056313,15.));
#20608=CARTESIAN_POINT('Ctrl Pts',(34.0424436187397,-26.880260834701,15.));
#20609=CARTESIAN_POINT('Ctrl Pts',(34.1446853651051,-26.895031013894,15.));
#20610=CARTESIAN_POINT('Ctrl Pts',(34.2471238425419,-26.9093352037262,15.));
#20611=CARTESIAN_POINT('Ctrl Pts',(34.3497565255724,-26.9231751225177,15.));
#20612=CARTESIAN_POINT('Ctrl Pts',(34.4731465943772,-26.9392277420462,15.));
#20613=CARTESIAN_POINT('Ctrl Pts',(34.5762105502273,-26.9520281195268,15.));
#20614=CARTESIAN_POINT('Ctrl Pts',(34.6588137898952,-26.9619003236529,15.));
#20615=CARTESIAN_POINT('Ctrl Pts',(34.7208516760814,-26.9690976283149,15.));
#20616=CARTESIAN_POINT('Ctrl Pts',(34.7622482477091,-26.9738038986838,15.));
#20617=CARTESIAN_POINT('Ctrl Pts',(26.9738038986838,-34.7622482477091,0.));
#20618=CARTESIAN_POINT('Ctrl Pts',(26.9738038986838,-34.7622482477091,18.));
#20619=CARTESIAN_POINT('Ctrl Pts',(26.9714507634922,-34.7415499619104,0.));
#20620=CARTESIAN_POINT('Ctrl Pts',(26.9714507634922,-34.7415499619104,18.));
#20621=CARTESIAN_POINT('Ctrl Pts',(26.9666985267608,-34.700172380686,0.));
#20622=CARTESIAN_POINT('Ctrl Pts',(26.9666985267608,-34.700172380686,18.));
#20623=CARTESIAN_POINT('Ctrl Pts',(26.9594322726214,-34.6381629799782,0.));
#20624=CARTESIAN_POINT('Ctrl Pts',(26.9594322726214,-34.6381629799782,18.));
#20625=CARTESIAN_POINT('Ctrl Pts',(26.9494680440307,-34.5555977590573,0.));
#20626=CARTESIAN_POINT('Ctrl Pts',(26.9494680440307,-34.5555977590573,18.));
#20627=CARTESIAN_POINT('Ctrl Pts',(26.936552305458,-34.4525815829097,0.));
#20628=CARTESIAN_POINT('Ctrl Pts',(26.936552305458,-34.4525815829097,18.));
#20629=CARTESIAN_POINT('Ctrl Pts',(26.9231751225177,-34.3497565255724,0.));
#20630=CARTESIAN_POINT('Ctrl Pts',(26.9231751225177,-34.3497565255724,18.));
#20631=CARTESIAN_POINT('Ctrl Pts',(26.9093352037262,-34.2471238425419,0.));
#20632=CARTESIAN_POINT('Ctrl Pts',(26.9093352037262,-34.2471238425419,18.));
#20633=CARTESIAN_POINT('Ctrl Pts',(26.8950310138939,-34.1446853651051,0.));
#20634=CARTESIAN_POINT('Ctrl Pts',(26.8950310138939,-34.1446853651051,18.));
#20635=CARTESIAN_POINT('Ctrl Pts',(26.880260834701,-34.0424436187397,0.));
#20636=CARTESIAN_POINT('Ctrl Pts',(26.880260834701,-34.0424436187397,18.));
#20637=CARTESIAN_POINT('Ctrl Pts',(26.8650228056313,-33.9404016650487,0.));
#20638=CARTESIAN_POINT('Ctrl Pts',(26.8650228056313,-33.9404016650487,18.));
#20639=CARTESIAN_POINT('Ctrl Pts',(26.8493149627661,-33.838562905895,0.));
#20640=CARTESIAN_POINT('Ctrl Pts',(26.8493149627661,-33.838562905895,18.));
#20641=CARTESIAN_POINT('Ctrl Pts',(26.8331352836666,-33.7369308933173,0.));
#20642=CARTESIAN_POINT('Ctrl Pts',(26.8331352836666,-33.7369308933173,18.));
#20643=CARTESIAN_POINT('Ctrl Pts',(26.8164817280846,-33.6355091508895,0.));
#20644=CARTESIAN_POINT('Ctrl Pts',(26.8164817280846,-33.6355091508895,18.));
#20645=CARTESIAN_POINT('Ctrl Pts',(26.7993522966985,-33.5343009499673,0.));
#20646=CARTESIAN_POINT('Ctrl Pts',(26.7993522966985,-33.5343009499673,18.));
#20647=CARTESIAN_POINT('Ctrl Pts',(26.7817450041181,-33.4333093513694,0.));
#20648=CARTESIAN_POINT('Ctrl Pts',(26.7817450041181,-33.4333093513694,18.));
#20649=CARTESIAN_POINT('Ctrl Pts',(26.7636578270526,-33.3325373307046,0.));
#20650=CARTESIAN_POINT('Ctrl Pts',(26.7636578270526,-33.3325373307046,18.));
#20651=CARTESIAN_POINT('Ctrl Pts',(26.7450886617884,-33.231987878652,0.));
#20652=CARTESIAN_POINT('Ctrl Pts',(26.7450886617884,-33.231987878652,18.));
#20653=CARTESIAN_POINT('Ctrl Pts',(26.7260352861618,-33.131664100194,0.));
#20654=CARTESIAN_POINT('Ctrl Pts',(26.7260352861618,-33.131664100194,18.));
#20655=CARTESIAN_POINT('Ctrl Pts',(26.7064953106254,-33.03156933761,0.));
#20656=CARTESIAN_POINT('Ctrl Pts',(26.7064953106254,-33.03156933761,18.));
#20657=CARTESIAN_POINT('Ctrl Pts',(26.6864661988934,-32.9317071576181,0.));
#20658=CARTESIAN_POINT('Ctrl Pts',(26.6864661988934,-32.9317071576181,18.));
#20659=CARTESIAN_POINT('Ctrl Pts',(26.6659453236976,-32.8320812678271,0.));
#20660=CARTESIAN_POINT('Ctrl Pts',(26.6659453236976,-32.8320812678271,18.));
#20661=CARTESIAN_POINT('Ctrl Pts',(26.6449300199763,-32.7326954489334,0.));
#20662=CARTESIAN_POINT('Ctrl Pts',(26.6449300199763,-32.7326954489334,18.));
#20663=CARTESIAN_POINT('Ctrl Pts',(26.6234176311244,-32.6335534898936,0.));
#20664=CARTESIAN_POINT('Ctrl Pts',(26.6234176311244,-32.6335534898936,18.));
#20665=CARTESIAN_POINT('Ctrl Pts',(26.6014055904817,-32.5346590925498,0.));
#20666=CARTESIAN_POINT('Ctrl Pts',(26.6014055904817,-32.5346590925498,18.));
#20667=CARTESIAN_POINT('Ctrl Pts',(26.5788913672813,-32.4360159072985,0.));
#20668=CARTESIAN_POINT('Ctrl Pts',(26.5788913672813,-32.4360159072985,18.));
#20669=CARTESIAN_POINT('Ctrl Pts',(26.555872320036,-32.3376276606981,0.));
#20670=CARTESIAN_POINT('Ctrl Pts',(26.555872320036,-32.3376276606981,18.));
#20671=CARTESIAN_POINT('Ctrl Pts',(26.5323455701117,-32.2394982626669,0.));
#20672=CARTESIAN_POINT('Ctrl Pts',(26.5323455701117,-32.2394982626669,18.));
#20673=CARTESIAN_POINT('Ctrl Pts',(26.5083078928862,-32.1416319023705,0.));
#20674=CARTESIAN_POINT('Ctrl Pts',(26.5083078928862,-32.1416319023705,18.));
#20675=CARTESIAN_POINT('Ctrl Pts',(26.4837555495616,-32.0440331917233,0.));
#20676=CARTESIAN_POINT('Ctrl Pts',(26.4837555495616,-32.0440331917233,18.));
#20677=CARTESIAN_POINT('Ctrl Pts',(26.4586843683627,-31.9467071093816,0.));
#20678=CARTESIAN_POINT('Ctrl Pts',(26.4586843683627,-31.9467071093816,18.));
#20679=CARTESIAN_POINT('Ctrl Pts',(26.433090040836,-31.849658771403,0.));
#20680=CARTESIAN_POINT('Ctrl Pts',(26.433090040836,-31.849658771403,18.));
#20681=CARTESIAN_POINT('Ctrl Pts',(26.4069683862784,-31.7528932299312,0.));
#20682=CARTESIAN_POINT('Ctrl Pts',(26.4069683862784,-31.7528932299312,18.));
#20683=CARTESIAN_POINT('Ctrl Pts',(26.3803155790949,-31.6564152990236,0.));
#20684=CARTESIAN_POINT('Ctrl Pts',(26.3803155790949,-31.6564152990236,18.));
#20685=CARTESIAN_POINT('Ctrl Pts',(26.353128528169,-31.5602292672984,0.));
#20686=CARTESIAN_POINT('Ctrl Pts',(26.353128528169,-31.5602292672984,18.));
#20687=CARTESIAN_POINT('Ctrl Pts',(26.3254046890485,-31.4643390378084,0.));
#20688=CARTESIAN_POINT('Ctrl Pts',(26.3254046890485,-31.4643390378084,18.));
#20689=CARTESIAN_POINT('Ctrl Pts',(26.2971413115295,-31.3687486937246,0.));
#20690=CARTESIAN_POINT('Ctrl Pts',(26.2971413115295,-31.3687486937246,18.));
#20691=CARTESIAN_POINT('Ctrl Pts',(26.2683347859175,-31.2734629900041,0.));
#20692=CARTESIAN_POINT('Ctrl Pts',(26.2683347859175,-31.2734629900041,18.));
#20693=CARTESIAN_POINT('Ctrl Pts',(26.2389800738214,-31.1784877826858,0.));
#20694=CARTESIAN_POINT('Ctrl Pts',(26.2389800738214,-31.1784877826858,18.));
#20695=CARTESIAN_POINT('Ctrl Pts',(26.2090698085494,-31.0838307058369,0.));
#20696=CARTESIAN_POINT('Ctrl Pts',(26.2090698085494,-31.0838307058369,18.));
#20697=CARTESIAN_POINT('Ctrl Pts',(26.1785946616165,-30.9895009017073,0.));
#20698=CARTESIAN_POINT('Ctrl Pts',(26.1785946616165,-30.9895009017073,18.));
#20699=CARTESIAN_POINT('Ctrl Pts',(26.1475450294082,-30.8955077633644,0.));
#20700=CARTESIAN_POINT('Ctrl Pts',(26.1475450294082,-30.8955077633644,18.));
#20701=CARTESIAN_POINT('Ctrl Pts',(26.1159125093178,-30.8018598357461,0.));
#20702=CARTESIAN_POINT('Ctrl Pts',(26.1159125093178,-30.8018598357461,18.));
#20703=CARTESIAN_POINT('Ctrl Pts',(26.0836911730968,-30.7085638682391,0.));
#20704=CARTESIAN_POINT('Ctrl Pts',(26.0836911730968,-30.7085638682391,18.));
#20705=CARTESIAN_POINT('Ctrl Pts',(26.0508796503166,-30.6156232634061,0.));
#20706=CARTESIAN_POINT('Ctrl Pts',(26.0508796503166,-30.6156232634061,18.));
#20707=CARTESIAN_POINT('Ctrl Pts',(26.0174801292225,-30.5230388264271,0.));
#20708=CARTESIAN_POINT('Ctrl Pts',(26.0174801292225,-30.5230388264271,18.));
#20709=CARTESIAN_POINT('Ctrl Pts',(25.9834942765902,-30.4308118142473,0.));
#20710=CARTESIAN_POINT('Ctrl Pts',(25.9834942765902,-30.4308118142473,18.));
#20711=CARTESIAN_POINT('Ctrl Pts',(25.9489196635424,-30.3389466074503,0.));
#20712=CARTESIAN_POINT('Ctrl Pts',(25.9489196635424,-30.3389466074503,18.));
#20713=CARTESIAN_POINT('Ctrl Pts',(25.9137466853317,-30.2474530144827,0.));
#20714=CARTESIAN_POINT('Ctrl Pts',(25.9137466853317,-30.2474530144827,18.));
#20715=CARTESIAN_POINT('Ctrl Pts',(25.8779535511027,-30.1563500154165,0.));
#20716=CARTESIAN_POINT('Ctrl Pts',(25.8779535511027,-30.1563500154165,18.));
#20717=CARTESIAN_POINT('Ctrl Pts',(25.8415089241134,-30.0656638016321,0.));
#20718=CARTESIAN_POINT('Ctrl Pts',(25.8415089241134,-30.0656638016321,18.));
#20719=CARTESIAN_POINT('Ctrl Pts',(25.8043812318214,-29.9754208429384,0.));
#20720=CARTESIAN_POINT('Ctrl Pts',(25.8043812318214,-29.9754208429384,18.));
#20721=CARTESIAN_POINT('Ctrl Pts',(25.7665469042913,-29.8856417535786,0.));
#20722=CARTESIAN_POINT('Ctrl Pts',(25.7665469042913,-29.8856417535786,18.));
#20723=CARTESIAN_POINT('Ctrl Pts',(25.7279973711305,-29.7963360859334,0.));
#20724=CARTESIAN_POINT('Ctrl Pts',(25.7279973711305,-29.7963360859334,18.));
#20725=CARTESIAN_POINT('Ctrl Pts',(25.6887507922748,-29.7074935910931,0.));
#20726=CARTESIAN_POINT('Ctrl Pts',(25.6887507922748,-29.7074935910931,18.));
#20727=CARTESIAN_POINT('Ctrl Pts',(25.6488438125835,-29.6190903904157,0.));
#20728=CARTESIAN_POINT('Ctrl Pts',(25.6488438125835,-29.6190903904157,18.));
#20729=CARTESIAN_POINT('Ctrl Pts',(25.6083094352667,-29.5311055094509,0.));
#20730=CARTESIAN_POINT('Ctrl Pts',(25.6083094352667,-29.5311055094509,18.));
#20731=CARTESIAN_POINT('Ctrl Pts',(25.5671572096726,-29.443535683207,0.));
#20732=CARTESIAN_POINT('Ctrl Pts',(25.5671572096726,-29.443535683207,18.));
#20733=CARTESIAN_POINT('Ctrl Pts',(25.5253562922582,-29.356408021119,0.));
#20734=CARTESIAN_POINT('Ctrl Pts',(25.5253562922582,-29.356408021119,18.));
#20735=CARTESIAN_POINT('Ctrl Pts',(25.4828076101654,-29.2698007967907,0.));
#20736=CARTESIAN_POINT('Ctrl Pts',(25.4828076101654,-29.2698007967907,18.));
#20737=CARTESIAN_POINT('Ctrl Pts',(25.4393679214513,-29.183825549991,0.));
#20738=CARTESIAN_POINT('Ctrl Pts',(25.4393679214513,-29.183825549991,18.));
#20739=CARTESIAN_POINT('Ctrl Pts',(25.3948997321278,-29.098589927237,0.));
#20740=CARTESIAN_POINT('Ctrl Pts',(25.3948997321278,-29.098589927237,18.));
#20741=CARTESIAN_POINT('Ctrl Pts',(25.3493168206005,-29.0141637699076,0.));
#20742=CARTESIAN_POINT('Ctrl Pts',(25.3493168206005,-29.0141637699076,18.));
#20743=CARTESIAN_POINT('Ctrl Pts',(25.3026235249214,-28.9305499160476,0.));
#20744=CARTESIAN_POINT('Ctrl Pts',(25.3026235249214,-28.9305499160476,18.));
#20745=CARTESIAN_POINT('Ctrl Pts',(25.2549775629725,-28.8476372998748,0.));
#20746=CARTESIAN_POINT('Ctrl Pts',(25.2549775629725,-28.8476372998748,18.));
#20747=CARTESIAN_POINT('Ctrl Pts',(25.2066127148845,-28.7652594076549,0.));
#20748=CARTESIAN_POINT('Ctrl Pts',(25.2066127148845,-28.7652594076549,18.));
#20749=CARTESIAN_POINT('Ctrl Pts',(25.1577170374459,-28.6832861366762,0.));
#20750=CARTESIAN_POINT('Ctrl Pts',(25.1577170374459,-28.6832861366762,18.));
#20751=CARTESIAN_POINT('Ctrl Pts',(25.1083211582389,-28.6017081342376,0.));
#20752=CARTESIAN_POINT('Ctrl Pts',(25.1083211582389,-28.6017081342376,18.));
#20753=CARTESIAN_POINT('Ctrl Pts',(25.0581926620043,-28.5207164321473,0.));
#20754=CARTESIAN_POINT('Ctrl Pts',(25.0581926620043,-28.5207164321473,18.));
#20755=CARTESIAN_POINT('Ctrl Pts',(25.0066999111736,-28.4408053900206,0.));
#20756=CARTESIAN_POINT('Ctrl Pts',(25.0066999111736,-28.4408053900206,18.));
#20757=CARTESIAN_POINT('Ctrl Pts',(24.9529811166897,-28.3626431274892,0.));
#20758=CARTESIAN_POINT('Ctrl Pts',(24.9529811166897,-28.3626431274892,18.));
#20759=CARTESIAN_POINT('Ctrl Pts',(24.9075246543798,-28.3020534756061,0.));
#20760=CARTESIAN_POINT('Ctrl Pts',(24.9075246543798,-28.3020534756061,18.));
#20761=CARTESIAN_POINT('Ctrl Pts',(24.8717258526943,-28.2579420132101,0.));
#20762=CARTESIAN_POINT('Ctrl Pts',(24.8717258526943,-28.2579420132101,18.));
#20763=CARTESIAN_POINT('Ctrl Pts',(24.8470618363541,-28.2291563988796,0.));
#20764=CARTESIAN_POINT('Ctrl Pts',(24.8470618363541,-28.2291563988796,18.));
#20765=CARTESIAN_POINT('Ctrl Pts',(24.8345302882955,-28.2149191006269,0.));
#20766=CARTESIAN_POINT('Ctrl Pts',(24.8345302882955,-28.2149191006269,18.));
#20767=CARTESIAN_POINT('',(26.9738038986839,-34.762248247709,0.));
#20768=CARTESIAN_POINT('Ctrl Pts',(24.8345302882955,-28.2149191006269,0.));
#20769=CARTESIAN_POINT('Ctrl Pts',(24.8470618363541,-28.2291563988796,0.));
#20770=CARTESIAN_POINT('Ctrl Pts',(24.8717258526943,-28.2579420132101,0.));
#20771=CARTESIAN_POINT('Ctrl Pts',(24.9075246543798,-28.3020534756061,0.));
#20772=CARTESIAN_POINT('Ctrl Pts',(24.9529811166897,-28.3626431274892,0.));
#20773=CARTESIAN_POINT('Ctrl Pts',(25.0066999111736,-28.4408053900206,0.));
#20774=CARTESIAN_POINT('Ctrl Pts',(25.0581926620043,-28.5207164321473,0.));
#20775=CARTESIAN_POINT('Ctrl Pts',(25.1083211582389,-28.6017081342376,0.));
#20776=CARTESIAN_POINT('Ctrl Pts',(25.1577170374459,-28.6832861366762,0.));
#20777=CARTESIAN_POINT('Ctrl Pts',(25.2066127148845,-28.7652594076549,0.));
#20778=CARTESIAN_POINT('Ctrl Pts',(25.2549775629725,-28.8476372998748,0.));
#20779=CARTESIAN_POINT('Ctrl Pts',(25.3026235249214,-28.9305499160476,0.));
#20780=CARTESIAN_POINT('Ctrl Pts',(25.3493168206005,-29.0141637699076,0.));
#20781=CARTESIAN_POINT('Ctrl Pts',(25.3948997321278,-29.098589927237,0.));
#20782=CARTESIAN_POINT('Ctrl Pts',(25.4393679214513,-29.183825549991,0.));
#20783=CARTESIAN_POINT('Ctrl Pts',(25.4828076101654,-29.2698007967907,0.));
#20784=CARTESIAN_POINT('Ctrl Pts',(25.5253562922582,-29.356408021119,0.));
#20785=CARTESIAN_POINT('Ctrl Pts',(25.5671572096726,-29.443535683207,0.));
#20786=CARTESIAN_POINT('Ctrl Pts',(25.6083094352667,-29.5311055094509,0.));
#20787=CARTESIAN_POINT('Ctrl Pts',(25.6488438125835,-29.6190903904157,0.));
#20788=CARTESIAN_POINT('Ctrl Pts',(25.6887507922748,-29.7074935910931,0.));
#20789=CARTESIAN_POINT('Ctrl Pts',(25.7279973711305,-29.7963360859334,0.));
#20790=CARTESIAN_POINT('Ctrl Pts',(25.7665469042913,-29.8856417535786,0.));
#20791=CARTESIAN_POINT('Ctrl Pts',(25.8043812318214,-29.9754208429384,0.));
#20792=CARTESIAN_POINT('Ctrl Pts',(25.8415089241134,-30.0656638016321,0.));
#20793=CARTESIAN_POINT('Ctrl Pts',(25.8779535511027,-30.1563500154165,0.));
#20794=CARTESIAN_POINT('Ctrl Pts',(25.9137466853317,-30.2474530144827,0.));
#20795=CARTESIAN_POINT('Ctrl Pts',(25.9489196635424,-30.3389466074503,0.));
#20796=CARTESIAN_POINT('Ctrl Pts',(25.9834942765902,-30.4308118142473,0.));
#20797=CARTESIAN_POINT('Ctrl Pts',(26.0174801292225,-30.5230388264271,0.));
#20798=CARTESIAN_POINT('Ctrl Pts',(26.0508796503166,-30.6156232634061,0.));
#20799=CARTESIAN_POINT('Ctrl Pts',(26.0836911730968,-30.7085638682391,0.));
#20800=CARTESIAN_POINT('Ctrl Pts',(26.1159125093178,-30.8018598357461,0.));
#20801=CARTESIAN_POINT('Ctrl Pts',(26.1475450294082,-30.8955077633644,0.));
#20802=CARTESIAN_POINT('Ctrl Pts',(26.1785946616165,-30.9895009017073,0.));
#20803=CARTESIAN_POINT('Ctrl Pts',(26.2090698085494,-31.0838307058369,0.));
#20804=CARTESIAN_POINT('Ctrl Pts',(26.2389800738214,-31.1784877826858,0.));
#20805=CARTESIAN_POINT('Ctrl Pts',(26.2683347859175,-31.2734629900041,0.));
#20806=CARTESIAN_POINT('Ctrl Pts',(26.2971413115295,-31.3687486937246,0.));
#20807=CARTESIAN_POINT('Ctrl Pts',(26.3254046890485,-31.4643390378084,0.));
#20808=CARTESIAN_POINT('Ctrl Pts',(26.353128528169,-31.5602292672984,0.));
#20809=CARTESIAN_POINT('Ctrl Pts',(26.3803155790949,-31.6564152990236,0.));
#20810=CARTESIAN_POINT('Ctrl Pts',(26.4069683862784,-31.7528932299312,0.));
#20811=CARTESIAN_POINT('Ctrl Pts',(26.433090040836,-31.849658771403,0.));
#20812=CARTESIAN_POINT('Ctrl Pts',(26.4586843683627,-31.9467071093816,0.));
#20813=CARTESIAN_POINT('Ctrl Pts',(26.4837555495616,-32.0440331917233,0.));
#20814=CARTESIAN_POINT('Ctrl Pts',(26.5083078928862,-32.1416319023705,0.));
#20815=CARTESIAN_POINT('Ctrl Pts',(26.5323455701117,-32.2394982626669,0.));
#20816=CARTESIAN_POINT('Ctrl Pts',(26.555872320036,-32.3376276606981,0.));
#20817=CARTESIAN_POINT('Ctrl Pts',(26.5788913672813,-32.4360159072985,0.));
#20818=CARTESIAN_POINT('Ctrl Pts',(26.6014055904817,-32.5346590925498,0.));
#20819=CARTESIAN_POINT('Ctrl Pts',(26.6234176311244,-32.6335534898936,0.));
#20820=CARTESIAN_POINT('Ctrl Pts',(26.6449300199763,-32.7326954489334,0.));
#20821=CARTESIAN_POINT('Ctrl Pts',(26.6659453236976,-32.8320812678271,0.));
#20822=CARTESIAN_POINT('Ctrl Pts',(26.6864661988934,-32.9317071576181,0.));
#20823=CARTESIAN_POINT('Ctrl Pts',(26.7064953106254,-33.03156933761,0.));
#20824=CARTESIAN_POINT('Ctrl Pts',(26.7260352861618,-33.131664100194,0.));
#20825=CARTESIAN_POINT('Ctrl Pts',(26.7450886617884,-33.231987878652,0.));
#20826=CARTESIAN_POINT('Ctrl Pts',(26.7636578270526,-33.3325373307046,0.));
#20827=CARTESIAN_POINT('Ctrl Pts',(26.7817450041181,-33.4333093513694,0.));
#20828=CARTESIAN_POINT('Ctrl Pts',(26.7993522966985,-33.5343009499673,0.));
#20829=CARTESIAN_POINT('Ctrl Pts',(26.8164817280846,-33.6355091508895,0.));
#20830=CARTESIAN_POINT('Ctrl Pts',(26.8331352836666,-33.7369308933173,0.));
#20831=CARTESIAN_POINT('Ctrl Pts',(26.8493149627661,-33.838562905895,0.));
#20832=CARTESIAN_POINT('Ctrl Pts',(26.8650228056313,-33.9404016650487,0.));
#20833=CARTESIAN_POINT('Ctrl Pts',(26.880260834701,-34.0424436187397,0.));
#20834=CARTESIAN_POINT('Ctrl Pts',(26.8950310138939,-34.1446853651051,0.));
#20835=CARTESIAN_POINT('Ctrl Pts',(26.9093352037262,-34.2471238425419,0.));
#20836=CARTESIAN_POINT('Ctrl Pts',(26.9231751225177,-34.3497565255724,0.));
#20837=CARTESIAN_POINT('Ctrl Pts',(26.9392277420461,-34.4731465943772,0.));
#20838=CARTESIAN_POINT('Ctrl Pts',(26.9520281195269,-34.5762105502273,0.));
#20839=CARTESIAN_POINT('Ctrl Pts',(26.9619003236529,-34.6588137898952,0.));
#20840=CARTESIAN_POINT('Ctrl Pts',(26.9690976283147,-34.7208516760814,0.));
#20841=CARTESIAN_POINT('Ctrl Pts',(26.9738038986838,-34.7622482477091,0.));
#20842=CARTESIAN_POINT('',(26.9738038986839,-34.762248247709,15.));
#20843=CARTESIAN_POINT('Ctrl Pts',(26.9738038986838,-34.7622482477091,15.));
#20844=CARTESIAN_POINT('Ctrl Pts',(26.9714507634922,-34.7415499619104,15.));
#20845=CARTESIAN_POINT('Ctrl Pts',(26.9666985267608,-34.700172380686,15.));
#20846=CARTESIAN_POINT('Ctrl Pts',(26.9594322726214,-34.6381629799782,15.));
#20847=CARTESIAN_POINT('Ctrl Pts',(26.9494680440307,-34.5555977590573,15.));
#20848=CARTESIAN_POINT('Ctrl Pts',(26.936552305458,-34.4525815829097,15.));
#20849=CARTESIAN_POINT('Ctrl Pts',(26.9231751225177,-34.3497565255724,15.));
#20850=CARTESIAN_POINT('Ctrl Pts',(26.9093352037262,-34.2471238425419,15.));
#20851=CARTESIAN_POINT('Ctrl Pts',(26.8950310138939,-34.1446853651051,15.));
#20852=CARTESIAN_POINT('Ctrl Pts',(26.880260834701,-34.0424436187397,15.));
#20853=CARTESIAN_POINT('Ctrl Pts',(26.8650228056313,-33.9404016650487,15.));
#20854=CARTESIAN_POINT('Ctrl Pts',(26.8493149627661,-33.838562905895,15.));
#20855=CARTESIAN_POINT('Ctrl Pts',(26.8331352836666,-33.7369308933173,15.));
#20856=CARTESIAN_POINT('Ctrl Pts',(26.8164817280846,-33.6355091508895,15.));
#20857=CARTESIAN_POINT('Ctrl Pts',(26.7993522966985,-33.5343009499673,15.));
#20858=CARTESIAN_POINT('Ctrl Pts',(26.7817450041181,-33.4333093513694,15.));
#20859=CARTESIAN_POINT('Ctrl Pts',(26.7636578270526,-33.3325373307046,15.));
#20860=CARTESIAN_POINT('Ctrl Pts',(26.7450886617884,-33.231987878652,15.));
#20861=CARTESIAN_POINT('Ctrl Pts',(26.7260352861618,-33.131664100194,15.));
#20862=CARTESIAN_POINT('Ctrl Pts',(26.7064953106254,-33.03156933761,15.));
#20863=CARTESIAN_POINT('Ctrl Pts',(26.6864661988934,-32.9317071576181,15.));
#20864=CARTESIAN_POINT('Ctrl Pts',(26.6659453236976,-32.8320812678271,15.));
#20865=CARTESIAN_POINT('Ctrl Pts',(26.6449300199763,-32.7326954489334,15.));
#20866=CARTESIAN_POINT('Ctrl Pts',(26.6234176311244,-32.6335534898936,15.));
#20867=CARTESIAN_POINT('Ctrl Pts',(26.6014055904817,-32.5346590925498,15.));
#20868=CARTESIAN_POINT('Ctrl Pts',(26.5788913672813,-32.4360159072985,15.));
#20869=CARTESIAN_POINT('Ctrl Pts',(26.555872320036,-32.3376276606981,15.));
#20870=CARTESIAN_POINT('Ctrl Pts',(26.5323455701117,-32.2394982626669,15.));
#20871=CARTESIAN_POINT('Ctrl Pts',(26.5083078928862,-32.1416319023705,15.));
#20872=CARTESIAN_POINT('Ctrl Pts',(26.4837555495616,-32.0440331917233,15.));
#20873=CARTESIAN_POINT('Ctrl Pts',(26.4586843683627,-31.9467071093816,15.));
#20874=CARTESIAN_POINT('Ctrl Pts',(26.433090040836,-31.849658771403,15.));
#20875=CARTESIAN_POINT('Ctrl Pts',(26.4069683862784,-31.7528932299312,15.));
#20876=CARTESIAN_POINT('Ctrl Pts',(26.3803155790949,-31.6564152990236,15.));
#20877=CARTESIAN_POINT('Ctrl Pts',(26.353128528169,-31.5602292672984,15.));
#20878=CARTESIAN_POINT('Ctrl Pts',(26.3254046890485,-31.4643390378084,15.));
#20879=CARTESIAN_POINT('Ctrl Pts',(26.2971413115295,-31.3687486937246,15.));
#20880=CARTESIAN_POINT('Ctrl Pts',(26.2683347859175,-31.2734629900041,15.));
#20881=CARTESIAN_POINT('Ctrl Pts',(26.2389800738214,-31.1784877826858,15.));
#20882=CARTESIAN_POINT('Ctrl Pts',(26.2090698085494,-31.0838307058369,15.));
#20883=CARTESIAN_POINT('Ctrl Pts',(26.1785946616165,-30.9895009017073,15.));
#20884=CARTESIAN_POINT('Ctrl Pts',(26.1475450294082,-30.8955077633644,15.));
#20885=CARTESIAN_POINT('Ctrl Pts',(26.1159125093178,-30.8018598357461,15.));
#20886=CARTESIAN_POINT('Ctrl Pts',(26.0836911730968,-30.7085638682391,15.));
#20887=CARTESIAN_POINT('Ctrl Pts',(26.0508796503166,-30.6156232634061,15.));
#20888=CARTESIAN_POINT('Ctrl Pts',(26.0174801292225,-30.5230388264271,15.));
#20889=CARTESIAN_POINT('Ctrl Pts',(25.9834942765902,-30.4308118142473,15.));
#20890=CARTESIAN_POINT('Ctrl Pts',(25.9489196635424,-30.3389466074503,15.));
#20891=CARTESIAN_POINT('Ctrl Pts',(25.9137466853317,-30.2474530144827,15.));
#20892=CARTESIAN_POINT('Ctrl Pts',(25.8779535511027,-30.1563500154165,15.));
#20893=CARTESIAN_POINT('Ctrl Pts',(25.8415089241134,-30.0656638016321,15.));
#20894=CARTESIAN_POINT('Ctrl Pts',(25.8043812318214,-29.9754208429384,15.));
#20895=CARTESIAN_POINT('Ctrl Pts',(25.7665469042913,-29.8856417535786,15.));
#20896=CARTESIAN_POINT('Ctrl Pts',(25.7279973711305,-29.7963360859334,15.));
#20897=CARTESIAN_POINT('Ctrl Pts',(25.6887507922748,-29.7074935910931,15.));
#20898=CARTESIAN_POINT('Ctrl Pts',(25.6488438125835,-29.6190903904157,15.));
#20899=CARTESIAN_POINT('Ctrl Pts',(25.6083094352667,-29.5311055094509,15.));
#20900=CARTESIAN_POINT('Ctrl Pts',(25.5671572096726,-29.443535683207,15.));
#20901=CARTESIAN_POINT('Ctrl Pts',(25.5253562922582,-29.356408021119,15.));
#20902=CARTESIAN_POINT('Ctrl Pts',(25.4828076101654,-29.2698007967907,15.));
#20903=CARTESIAN_POINT('Ctrl Pts',(25.4393679214513,-29.183825549991,15.));
#20904=CARTESIAN_POINT('Ctrl Pts',(25.3948997321278,-29.098589927237,15.));
#20905=CARTESIAN_POINT('Ctrl Pts',(25.3493168206005,-29.0141637699076,15.));
#20906=CARTESIAN_POINT('Ctrl Pts',(25.3026235249214,-28.9305499160476,15.));
#20907=CARTESIAN_POINT('Ctrl Pts',(25.2549775629725,-28.8476372998748,15.));
#20908=CARTESIAN_POINT('Ctrl Pts',(25.2066127148845,-28.7652594076549,15.));
#20909=CARTESIAN_POINT('Ctrl Pts',(25.1577170374459,-28.6832861366762,15.));
#20910=CARTESIAN_POINT('Ctrl Pts',(25.1083211582389,-28.6017081342376,15.));
#20911=CARTESIAN_POINT('Ctrl Pts',(25.0581926620043,-28.5207164321473,15.));
#20912=CARTESIAN_POINT('Ctrl Pts',(25.0066999111736,-28.4408053900206,15.));
#20913=CARTESIAN_POINT('Ctrl Pts',(24.9529811166897,-28.3626431274892,15.));
#20914=CARTESIAN_POINT('Ctrl Pts',(24.9075246543798,-28.3020534756061,15.));
#20915=CARTESIAN_POINT('Ctrl Pts',(24.8717258526943,-28.2579420132101,15.));
#20916=CARTESIAN_POINT('Ctrl Pts',(24.8470618363541,-28.2291563988796,15.));
#20917=CARTESIAN_POINT('Ctrl Pts',(24.8345302882955,-28.2149191006269,15.));
#20918=CARTESIAN_POINT('',(26.9738038986839,-34.762248247709,0.));
#20919=CARTESIAN_POINT('Origin',(6.66146233219318E-12,-9.16871631793044E-12,
0.));
#20920=CARTESIAN_POINT('',(24.725498909423,-36.3957374383337,0.));
#20921=CARTESIAN_POINT('Origin',(6.66146233219318E-12,-9.16871631793044E-12,
0.));
#20922=CARTESIAN_POINT('',(24.725498909423,-36.3957374383337,15.));
#20923=CARTESIAN_POINT('Origin',(6.66146233219318E-12,-9.16871631793044E-12,
15.));
#20924=CARTESIAN_POINT('',(24.725498909423,-36.3957374383337,0.));
#20925=CARTESIAN_POINT('Ctrl Pts',(19.1596907609891,-32.3379313568208,0.));
#20926=CARTESIAN_POINT('Ctrl Pts',(19.1596907609891,-32.3379313568208,18.));
#20927=CARTESIAN_POINT('Ctrl Pts',(19.1693587749508,-32.3542491343753,0.));
#20928=CARTESIAN_POINT('Ctrl Pts',(19.1693587749508,-32.3542491343753,18.));
#20929=CARTESIAN_POINT('Ctrl Pts',(19.1891139208368,-32.3866012518553,0.));
#20930=CARTESIAN_POINT('Ctrl Pts',(19.1891139208368,-32.3866012518553,18.));
#20931=CARTESIAN_POINT('Ctrl Pts',(19.2200039764927,-32.4342791270009,0.));
#20932=CARTESIAN_POINT('Ctrl Pts',(19.2200039764927,-32.4342791270009,18.));
#20933=CARTESIAN_POINT('Ctrl Pts',(19.2635813403783,-32.4962340238036,0.));
#20934=CARTESIAN_POINT('Ctrl Pts',(19.2635813403783,-32.4962340238036,18.));
#20935=CARTESIAN_POINT('Ctrl Pts',(19.3213180490743,-32.5714771007861,0.));
#20936=CARTESIAN_POINT('Ctrl Pts',(19.3213180490743,-32.5714771007861,18.));
#20937=CARTESIAN_POINT('Ctrl Pts',(19.381405831319,-32.6451434870609,0.));
#20938=CARTESIAN_POINT('Ctrl Pts',(19.381405831319,-32.6451434870609,18.));
#20939=CARTESIAN_POINT('Ctrl Pts',(19.4429429601189,-32.7178463324062,0.));
#20940=CARTESIAN_POINT('Ctrl Pts',(19.4429429601189,-32.7178463324062,18.));
#20941=CARTESIAN_POINT('Ctrl Pts',(19.5052640847974,-32.7900335943248,0.));
#20942=CARTESIAN_POINT('Ctrl Pts',(19.5052640847974,-32.7900335943248,18.));
#20943=CARTESIAN_POINT('Ctrl Pts',(19.5681157030437,-32.8618672807884,0.));
#20944=CARTESIAN_POINT('Ctrl Pts',(19.5681157030437,-32.8618672807884,18.));
#20945=CARTESIAN_POINT('Ctrl Pts',(19.6315161742485,-32.9333211533788,0.));
#20946=CARTESIAN_POINT('Ctrl Pts',(19.6315161742485,-32.9333211533788,18.));
#20947=CARTESIAN_POINT('Ctrl Pts',(19.6956473461873,-33.004256563411,0.));
#20948=CARTESIAN_POINT('Ctrl Pts',(19.6956473461873,-33.004256563411,18.));
#20949=CARTESIAN_POINT('Ctrl Pts',(19.7607398248651,-33.0745026283418,0.));
#20950=CARTESIAN_POINT('Ctrl Pts',(19.7607398248651,-33.0745026283418,18.));
#20951=CARTESIAN_POINT('Ctrl Pts',(19.8269479776239,-33.1439436707661,0.));
#20952=CARTESIAN_POINT('Ctrl Pts',(19.8269479776239,-33.1439436707661,18.));
#20953=CARTESIAN_POINT('Ctrl Pts',(19.8942704458546,-33.2125746879471,0.));
#20954=CARTESIAN_POINT('Ctrl Pts',(19.8942704458546,-33.2125746879471,18.));
#20955=CARTESIAN_POINT('Ctrl Pts',(19.9626141625205,-33.2804560993213,0.));
#20956=CARTESIAN_POINT('Ctrl Pts',(19.9626141625205,-33.2804560993213,18.));
#20957=CARTESIAN_POINT('Ctrl Pts',(20.0318342617212,-33.3476854048385,0.));
#20958=CARTESIAN_POINT('Ctrl Pts',(20.0318342617212,-33.3476854048385,18.));
#20959=CARTESIAN_POINT('Ctrl Pts',(20.1017803986381,-33.4143643679979,0.));
#20960=CARTESIAN_POINT('Ctrl Pts',(20.1017803986381,-33.4143643679979,18.));
#20961=CARTESIAN_POINT('Ctrl Pts',(20.1723475154533,-33.480563024813,0.));
#20962=CARTESIAN_POINT('Ctrl Pts',(20.1723475154533,-33.480563024813,18.));
#20963=CARTESIAN_POINT('Ctrl Pts',(20.243500298383,-33.5463023319603,0.));
#20964=CARTESIAN_POINT('Ctrl Pts',(20.243500298383,-33.5463023319603,18.));
#20965=CARTESIAN_POINT('Ctrl Pts',(20.3152448035297,-33.6115742164079,0.));
#20966=CARTESIAN_POINT('Ctrl Pts',(20.3152448035297,-33.6115742164079,18.));
#20967=CARTESIAN_POINT('Ctrl Pts',(20.3876111773341,-33.6763537716992,0.));
#20968=CARTESIAN_POINT('Ctrl Pts',(20.3876111773341,-33.6763537716992,18.));
#20969=CARTESIAN_POINT('Ctrl Pts',(20.4606334536183,-33.7406135254082,0.));
#20970=CARTESIAN_POINT('Ctrl Pts',(20.4606334536183,-33.7406135254082,18.));
#20971=CARTESIAN_POINT('Ctrl Pts',(20.5343269914034,-33.8043393734971,0.));
#20972=CARTESIAN_POINT('Ctrl Pts',(20.5343269914034,-33.8043393734971,18.));
#20973=CARTESIAN_POINT('Ctrl Pts',(20.6086800574386,-33.8675365150454,0.));
#20974=CARTESIAN_POINT('Ctrl Pts',(20.6086800574386,-33.8675365150454,18.));
#20975=CARTESIAN_POINT('Ctrl Pts',(20.683665762903,-33.9302209962425,0.));
#20976=CARTESIAN_POINT('Ctrl Pts',(20.683665762903,-33.9302209962425,18.));
#20977=CARTESIAN_POINT('Ctrl Pts',(20.7592491770603,-33.9924146647395,0.));
#20978=CARTESIAN_POINT('Ctrl Pts',(20.7592491770603,-33.9924146647395,18.));
#20979=CARTESIAN_POINT('Ctrl Pts',(20.8353957068415,-34.0541392299678,0.));
#20980=CARTESIAN_POINT('Ctrl Pts',(20.8353957068415,-34.0541392299678,18.));
#20981=CARTESIAN_POINT('Ctrl Pts',(20.9120805673809,-34.1154095510973,0.));
#20982=CARTESIAN_POINT('Ctrl Pts',(20.9120805673809,-34.1154095510973,18.));
#20983=CARTESIAN_POINT('Ctrl Pts',(20.9892914622612,-34.176231731809,0.));
#20984=CARTESIAN_POINT('Ctrl Pts',(20.9892914622612,-34.176231731809,18.));
#20985=CARTESIAN_POINT('Ctrl Pts',(21.0670234747355,-34.2366067284279,0.));
#20986=CARTESIAN_POINT('Ctrl Pts',(21.0670234747355,-34.2366067284279,18.));
#20987=CARTESIAN_POINT('Ctrl Pts',(21.1452759244399,-34.2965325673384,0.));
#20988=CARTESIAN_POINT('Ctrl Pts',(21.1452759244399,-34.2965325673384,18.));
#20989=CARTESIAN_POINT('Ctrl Pts',(21.2240487218078,-34.3560069185815,0.));
#20990=CARTESIAN_POINT('Ctrl Pts',(21.2240487218078,-34.3560069185815,18.));
#20991=CARTESIAN_POINT('Ctrl Pts',(21.3033382073239,-34.4150300340623,0.));
#20992=CARTESIAN_POINT('Ctrl Pts',(21.3033382073239,-34.4150300340623,18.));
#20993=CARTESIAN_POINT('Ctrl Pts',(21.3831361300104,-34.4736054662052,0.));
#20994=CARTESIAN_POINT('Ctrl Pts',(21.3831361300104,-34.4736054662052,18.));
#20995=CARTESIAN_POINT('Ctrl Pts',(21.4634317666004,-34.5317385658329,0.));
#20996=CARTESIAN_POINT('Ctrl Pts',(21.4634317666004,-34.5317385658329,18.));
#20997=CARTESIAN_POINT('Ctrl Pts',(21.5442132160757,-34.5894355639082,0.));
#20998=CARTESIAN_POINT('Ctrl Pts',(21.5442132160757,-34.5894355639082,18.));
#20999=CARTESIAN_POINT('Ctrl Pts',(21.6254689009796,-34.6467025072367,0.));
#21000=CARTESIAN_POINT('Ctrl Pts',(21.6254689009796,-34.6467025072367,18.));
#21001=CARTESIAN_POINT('Ctrl Pts',(21.7071892844497,-34.7035440429025,0.));
#21002=CARTESIAN_POINT('Ctrl Pts',(21.7071892844497,-34.7035440429025,18.));
#21003=CARTESIAN_POINT('Ctrl Pts',(21.7893672401137,-34.7599631530844,0.));
#21004=CARTESIAN_POINT('Ctrl Pts',(21.7893672401137,-34.7599631530844,18.));
#21005=CARTESIAN_POINT('Ctrl Pts',(21.8719971302817,-34.8159618014436,0.));
#21006=CARTESIAN_POINT('Ctrl Pts',(21.8719971302817,-34.8159618014436,18.));
#21007=CARTESIAN_POINT('Ctrl Pts',(21.9550742217675,-34.8715413418101,0.));
#21008=CARTESIAN_POINT('Ctrl Pts',(21.9550742217675,-34.8715413418101,18.));
#21009=CARTESIAN_POINT('Ctrl Pts',(22.0385940162683,-34.9267029879922,0.));
#21010=CARTESIAN_POINT('Ctrl Pts',(22.0385940162683,-34.9267029879922,18.));
#21011=CARTESIAN_POINT('Ctrl Pts',(22.1225514798584,-34.9814483545602,0.));
#21012=CARTESIAN_POINT('Ctrl Pts',(22.1225514798584,-34.9814483545602,18.));
#21013=CARTESIAN_POINT('Ctrl Pts',(22.2069408519232,-35.0357795922459,0.));
#21014=CARTESIAN_POINT('Ctrl Pts',(22.2069408519232,-35.0357795922459,18.));
#21015=CARTESIAN_POINT('Ctrl Pts',(22.2917560356802,-35.0896991159359,0.));
#21016=CARTESIAN_POINT('Ctrl Pts',(22.2917560356802,-35.0896991159359,18.));
#21017=CARTESIAN_POINT('Ctrl Pts',(22.3769908340843,-35.1432094422642,0.));
#21018=CARTESIAN_POINT('Ctrl Pts',(22.3769908340843,-35.1432094422642,18.));
#21019=CARTESIAN_POINT('Ctrl Pts',(22.4626392230023,-35.1963130003353,0.));
#21020=CARTESIAN_POINT('Ctrl Pts',(22.4626392230023,-35.1963130003353,18.));
#21021=CARTESIAN_POINT('Ctrl Pts',(22.5486956608909,-35.2490119207975,0.));
#21022=CARTESIAN_POINT('Ctrl Pts',(22.5486956608909,-35.2490119207975,18.));
#21023=CARTESIAN_POINT('Ctrl Pts',(22.635155167154,-35.3013079759253,0.));
#21024=CARTESIAN_POINT('Ctrl Pts',(22.635155167154,-35.3013079759253,18.));
#21025=CARTESIAN_POINT('Ctrl Pts',(22.7220131336912,-35.3532026952313,0.));
#21026=CARTESIAN_POINT('Ctrl Pts',(22.7220131336912,-35.3532026952313,18.));
#21027=CARTESIAN_POINT('Ctrl Pts',(22.8092652000706,-35.4046974393492,0.));
#21028=CARTESIAN_POINT('Ctrl Pts',(22.8092652000706,-35.4046974393492,18.));
#21029=CARTESIAN_POINT('Ctrl Pts',(22.8969071125089,-35.4557934871468,0.));
#21030=CARTESIAN_POINT('Ctrl Pts',(22.8969071125089,-35.4557934871468,18.));
#21031=CARTESIAN_POINT('Ctrl Pts',(22.9849345572033,-35.5064921357308,0.));
#21032=CARTESIAN_POINT('Ctrl Pts',(22.9849345572033,-35.5064921357308,18.));
#21033=CARTESIAN_POINT('Ctrl Pts',(23.0733431097058,-35.5567947408311,0.));
#21034=CARTESIAN_POINT('Ctrl Pts',(23.0733431097058,-35.5567947408311,18.));
#21035=CARTESIAN_POINT('Ctrl Pts',(23.1621283508111,-35.6067026687722,0.));
#21036=CARTESIAN_POINT('Ctrl Pts',(23.1621283508111,-35.6067026687722,18.));
#21037=CARTESIAN_POINT('Ctrl Pts',(23.2512859425032,-35.6562172725207,0.));
#21038=CARTESIAN_POINT('Ctrl Pts',(23.2512859425032,-35.6562172725207,18.));
#21039=CARTESIAN_POINT('Ctrl Pts',(23.3408117088761,-35.7053398620512,0.));
#21040=CARTESIAN_POINT('Ctrl Pts',(23.3408117088761,-35.7053398620512,18.));
#21041=CARTESIAN_POINT('Ctrl Pts',(23.4307017328227,-35.7540716771372,0.));
#21042=CARTESIAN_POINT('Ctrl Pts',(23.4307017328227,-35.7540716771372,18.));
#21043=CARTESIAN_POINT('Ctrl Pts',(23.5209523746427,-35.8024138716897,0.));
#21044=CARTESIAN_POINT('Ctrl Pts',(23.5209523746427,-35.8024138716897,18.));
#21045=CARTESIAN_POINT('Ctrl Pts',(23.611560139948,-35.8503675222884,0.));
#21046=CARTESIAN_POINT('Ctrl Pts',(23.611560139948,-35.8503675222884,18.));
#21047=CARTESIAN_POINT('Ctrl Pts',(23.7025215735353,-35.8979336336837,0.));
#21048=CARTESIAN_POINT('Ctrl Pts',(23.7025215735353,-35.8979336336837,18.));
#21049=CARTESIAN_POINT('Ctrl Pts',(23.7938331508737,-35.9451131482488,0.));
#21050=CARTESIAN_POINT('Ctrl Pts',(23.7938331508737,-35.9451131482488,18.));
#21051=CARTESIAN_POINT('Ctrl Pts',(23.8854911428946,-35.991906956547,0.));
#21052=CARTESIAN_POINT('Ctrl Pts',(23.8854911428946,-35.991906956547,18.));
#21053=CARTESIAN_POINT('Ctrl Pts',(23.9774915680089,-36.0383159101253,0.));
#21054=CARTESIAN_POINT('Ctrl Pts',(23.9774915680089,-36.0383159101253,18.));
#21055=CARTESIAN_POINT('Ctrl Pts',(24.0698304230588,-36.0843408347974,0.));
#21056=CARTESIAN_POINT('Ctrl Pts',(24.0698304230588,-36.0843408347974,18.));
#21057=CARTESIAN_POINT('Ctrl Pts',(24.1625038657964,-36.1299825471271,0.));
#21058=CARTESIAN_POINT('Ctrl Pts',(24.1625038657964,-36.1299825471271,18.));
#21059=CARTESIAN_POINT('Ctrl Pts',(24.2555084095331,-36.1752418704833,0.));
#21060=CARTESIAN_POINT('Ctrl Pts',(24.2555084095331,-36.1752418704833,18.));
#21061=CARTESIAN_POINT('Ctrl Pts',(24.3488411214068,-36.2201196586696,0.));
#21062=CARTESIAN_POINT('Ctrl Pts',(24.3488411214068,-36.2201196586696,18.));
#21063=CARTESIAN_POINT('Ctrl Pts',(24.4424997853604,-36.2646168058395,0.));
#21064=CARTESIAN_POINT('Ctrl Pts',(24.4424997853604,-36.2646168058395,18.));
#21065=CARTESIAN_POINT('Ctrl Pts',(24.5364828082556,-36.308734152297,0.));
#21066=CARTESIAN_POINT('Ctrl Pts',(24.5364828082556,-36.308734152297,18.));
#21067=CARTESIAN_POINT('Ctrl Pts',(24.6119278836614,-36.3437247532369,0.));
#21068=CARTESIAN_POINT('Ctrl Pts',(24.6119278836614,-36.3437247532369,18.));
#21069=CARTESIAN_POINT('Ctrl Pts',(24.6686569322615,-36.369797330215,0.));
#21070=CARTESIAN_POINT('Ctrl Pts',(24.6686569322615,-36.369797330215,18.));
#21071=CARTESIAN_POINT('Ctrl Pts',(24.7065408286023,-36.3871033517098,0.));
#21072=CARTESIAN_POINT('Ctrl Pts',(24.7065408286023,-36.3871033517098,18.));
#21073=CARTESIAN_POINT('Ctrl Pts',(24.725498909423,-36.3957374383337,0.));
#21074=CARTESIAN_POINT('Ctrl Pts',(24.725498909423,-36.3957374383337,18.));
#21075=CARTESIAN_POINT('Ctrl Pts',(19.1596907609891,-32.3379313568208,0.));
#21076=CARTESIAN_POINT('Ctrl Pts',(19.1693587749508,-32.3542491343753,0.));
#21077=CARTESIAN_POINT('Ctrl Pts',(19.1891139208368,-32.3866012518553,0.));
#21078=CARTESIAN_POINT('Ctrl Pts',(19.2200039764927,-32.4342791270009,0.));
#21079=CARTESIAN_POINT('Ctrl Pts',(19.2635813403783,-32.4962340238036,0.));
#21080=CARTESIAN_POINT('Ctrl Pts',(19.3213180490743,-32.5714771007861,0.));
#21081=CARTESIAN_POINT('Ctrl Pts',(19.381405831319,-32.6451434870609,0.));
#21082=CARTESIAN_POINT('Ctrl Pts',(19.4429429601189,-32.7178463324062,0.));
#21083=CARTESIAN_POINT('Ctrl Pts',(19.5052640847974,-32.7900335943248,0.));
#21084=CARTESIAN_POINT('Ctrl Pts',(19.5681157030437,-32.8618672807884,0.));
#21085=CARTESIAN_POINT('Ctrl Pts',(19.6315161742485,-32.9333211533788,0.));
#21086=CARTESIAN_POINT('Ctrl Pts',(19.6956473461873,-33.004256563411,0.));
#21087=CARTESIAN_POINT('Ctrl Pts',(19.7607398248651,-33.0745026283418,0.));
#21088=CARTESIAN_POINT('Ctrl Pts',(19.8269479776239,-33.1439436707661,0.));
#21089=CARTESIAN_POINT('Ctrl Pts',(19.8942704458546,-33.2125746879471,0.));
#21090=CARTESIAN_POINT('Ctrl Pts',(19.9626141625205,-33.2804560993213,0.));
#21091=CARTESIAN_POINT('Ctrl Pts',(20.0318342617212,-33.3476854048385,0.));
#21092=CARTESIAN_POINT('Ctrl Pts',(20.1017803986381,-33.4143643679979,0.));
#21093=CARTESIAN_POINT('Ctrl Pts',(20.1723475154533,-33.480563024813,0.));
#21094=CARTESIAN_POINT('Ctrl Pts',(20.243500298383,-33.5463023319603,0.));
#21095=CARTESIAN_POINT('Ctrl Pts',(20.3152448035297,-33.6115742164079,0.));
#21096=CARTESIAN_POINT('Ctrl Pts',(20.3876111773341,-33.6763537716992,0.));
#21097=CARTESIAN_POINT('Ctrl Pts',(20.4606334536183,-33.7406135254082,0.));
#21098=CARTESIAN_POINT('Ctrl Pts',(20.5343269914034,-33.8043393734971,0.));
#21099=CARTESIAN_POINT('Ctrl Pts',(20.6086800574386,-33.8675365150454,0.));
#21100=CARTESIAN_POINT('Ctrl Pts',(20.683665762903,-33.9302209962425,0.));
#21101=CARTESIAN_POINT('Ctrl Pts',(20.7592491770603,-33.9924146647395,0.));
#21102=CARTESIAN_POINT('Ctrl Pts',(20.8353957068415,-34.0541392299678,0.));
#21103=CARTESIAN_POINT('Ctrl Pts',(20.9120805673809,-34.1154095510973,0.));
#21104=CARTESIAN_POINT('Ctrl Pts',(20.9892914622612,-34.176231731809,0.));
#21105=CARTESIAN_POINT('Ctrl Pts',(21.0670234747355,-34.2366067284279,0.));
#21106=CARTESIAN_POINT('Ctrl Pts',(21.1452759244399,-34.2965325673384,0.));
#21107=CARTESIAN_POINT('Ctrl Pts',(21.2240487218078,-34.3560069185815,0.));
#21108=CARTESIAN_POINT('Ctrl Pts',(21.3033382073239,-34.4150300340623,0.));
#21109=CARTESIAN_POINT('Ctrl Pts',(21.3831361300104,-34.4736054662052,0.));
#21110=CARTESIAN_POINT('Ctrl Pts',(21.4634317666004,-34.5317385658329,0.));
#21111=CARTESIAN_POINT('Ctrl Pts',(21.5442132160757,-34.5894355639082,0.));
#21112=CARTESIAN_POINT('Ctrl Pts',(21.6254689009796,-34.6467025072367,0.));
#21113=CARTESIAN_POINT('Ctrl Pts',(21.7071892844497,-34.7035440429025,0.));
#21114=CARTESIAN_POINT('Ctrl Pts',(21.7893672401137,-34.7599631530844,0.));
#21115=CARTESIAN_POINT('Ctrl Pts',(21.8719971302817,-34.8159618014436,0.));
#21116=CARTESIAN_POINT('Ctrl Pts',(21.9550742217675,-34.8715413418101,0.));
#21117=CARTESIAN_POINT('Ctrl Pts',(22.0385940162683,-34.9267029879922,0.));
#21118=CARTESIAN_POINT('Ctrl Pts',(22.1225514798584,-34.9814483545602,0.));
#21119=CARTESIAN_POINT('Ctrl Pts',(22.2069408519232,-35.0357795922459,0.));
#21120=CARTESIAN_POINT('Ctrl Pts',(22.2917560356802,-35.0896991159359,0.));
#21121=CARTESIAN_POINT('Ctrl Pts',(22.3769908340843,-35.1432094422642,0.));
#21122=CARTESIAN_POINT('Ctrl Pts',(22.4626392230023,-35.1963130003353,0.));
#21123=CARTESIAN_POINT('Ctrl Pts',(22.5486956608909,-35.2490119207975,0.));
#21124=CARTESIAN_POINT('Ctrl Pts',(22.635155167154,-35.3013079759253,0.));
#21125=CARTESIAN_POINT('Ctrl Pts',(22.7220131336912,-35.3532026952313,0.));
#21126=CARTESIAN_POINT('Ctrl Pts',(22.8092652000706,-35.4046974393492,0.));
#21127=CARTESIAN_POINT('Ctrl Pts',(22.8969071125089,-35.4557934871468,0.));
#21128=CARTESIAN_POINT('Ctrl Pts',(22.9849345572033,-35.5064921357308,0.));
#21129=CARTESIAN_POINT('Ctrl Pts',(23.0733431097058,-35.5567947408311,0.));
#21130=CARTESIAN_POINT('Ctrl Pts',(23.1621283508111,-35.6067026687722,0.));
#21131=CARTESIAN_POINT('Ctrl Pts',(23.2512859425032,-35.6562172725207,0.));
#21132=CARTESIAN_POINT('Ctrl Pts',(23.3408117088761,-35.7053398620512,0.));
#21133=CARTESIAN_POINT('Ctrl Pts',(23.4307017328227,-35.7540716771372,0.));
#21134=CARTESIAN_POINT('Ctrl Pts',(23.5209523746427,-35.8024138716897,0.));
#21135=CARTESIAN_POINT('Ctrl Pts',(23.611560139948,-35.8503675222884,0.));
#21136=CARTESIAN_POINT('Ctrl Pts',(23.7025215735353,-35.8979336336837,0.));
#21137=CARTESIAN_POINT('Ctrl Pts',(23.7938331508737,-35.9451131482488,0.));
#21138=CARTESIAN_POINT('Ctrl Pts',(23.8854911428946,-35.991906956547,0.));
#21139=CARTESIAN_POINT('Ctrl Pts',(23.9774915680089,-36.0383159101253,0.));
#21140=CARTESIAN_POINT('Ctrl Pts',(24.0698304230588,-36.0843408347974,0.));
#21141=CARTESIAN_POINT('Ctrl Pts',(24.1625038657964,-36.1299825471271,0.));
#21142=CARTESIAN_POINT('Ctrl Pts',(24.2555084095331,-36.1752418704833,0.));
#21143=CARTESIAN_POINT('Ctrl Pts',(24.3488411214068,-36.2201196586696,0.));
#21144=CARTESIAN_POINT('Ctrl Pts',(24.4612315181511,-36.2735162352735,0.));
#21145=CARTESIAN_POINT('Ctrl Pts',(24.5552956307817,-36.3175386315529,0.));
#21146=CARTESIAN_POINT('Ctrl Pts',(24.630805301288,-36.3524534604649,0.));
#21147=CARTESIAN_POINT('Ctrl Pts',(24.6875827477483,-36.37846926509,0.));
#21148=CARTESIAN_POINT('Ctrl Pts',(24.725498909423,-36.3957374383337,0.));
#21149=CARTESIAN_POINT('Ctrl Pts',(19.1596907609891,-32.3379313568208,15.));
#21150=CARTESIAN_POINT('Ctrl Pts',(19.1693587749508,-32.3542491343753,15.));
#21151=CARTESIAN_POINT('Ctrl Pts',(19.1891139208368,-32.3866012518553,15.));
#21152=CARTESIAN_POINT('Ctrl Pts',(19.2200039764927,-32.4342791270009,15.));
#21153=CARTESIAN_POINT('Ctrl Pts',(19.2635813403783,-32.4962340238036,15.));
#21154=CARTESIAN_POINT('Ctrl Pts',(19.3213180490743,-32.5714771007861,15.));
#21155=CARTESIAN_POINT('Ctrl Pts',(19.381405831319,-32.6451434870609,15.));
#21156=CARTESIAN_POINT('Ctrl Pts',(19.4429429601189,-32.7178463324062,15.));
#21157=CARTESIAN_POINT('Ctrl Pts',(19.5052640847974,-32.7900335943248,15.));
#21158=CARTESIAN_POINT('Ctrl Pts',(19.5681157030437,-32.8618672807884,15.));
#21159=CARTESIAN_POINT('Ctrl Pts',(19.6315161742485,-32.9333211533788,15.));
#21160=CARTESIAN_POINT('Ctrl Pts',(19.6956473461873,-33.004256563411,15.));
#21161=CARTESIAN_POINT('Ctrl Pts',(19.7607398248651,-33.0745026283418,15.));
#21162=CARTESIAN_POINT('Ctrl Pts',(19.8269479776239,-33.1439436707661,15.));
#21163=CARTESIAN_POINT('Ctrl Pts',(19.8942704458546,-33.2125746879471,15.));
#21164=CARTESIAN_POINT('Ctrl Pts',(19.9626141625205,-33.2804560993213,15.));
#21165=CARTESIAN_POINT('Ctrl Pts',(20.0318342617212,-33.3476854048385,15.));
#21166=CARTESIAN_POINT('Ctrl Pts',(20.1017803986381,-33.4143643679979,15.));
#21167=CARTESIAN_POINT('Ctrl Pts',(20.1723475154533,-33.480563024813,15.));
#21168=CARTESIAN_POINT('Ctrl Pts',(20.243500298383,-33.5463023319603,15.));
#21169=CARTESIAN_POINT('Ctrl Pts',(20.3152448035297,-33.6115742164079,15.));
#21170=CARTESIAN_POINT('Ctrl Pts',(20.3876111773341,-33.6763537716992,15.));
#21171=CARTESIAN_POINT('Ctrl Pts',(20.4606334536183,-33.7406135254082,15.));
#21172=CARTESIAN_POINT('Ctrl Pts',(20.5343269914034,-33.8043393734971,15.));
#21173=CARTESIAN_POINT('Ctrl Pts',(20.6086800574386,-33.8675365150454,15.));
#21174=CARTESIAN_POINT('Ctrl Pts',(20.683665762903,-33.9302209962425,15.));
#21175=CARTESIAN_POINT('Ctrl Pts',(20.7592491770603,-33.9924146647395,15.));
#21176=CARTESIAN_POINT('Ctrl Pts',(20.8353957068415,-34.0541392299678,15.));
#21177=CARTESIAN_POINT('Ctrl Pts',(20.9120805673809,-34.1154095510973,15.));
#21178=CARTESIAN_POINT('Ctrl Pts',(20.9892914622612,-34.176231731809,15.));
#21179=CARTESIAN_POINT('Ctrl Pts',(21.0670234747355,-34.2366067284279,15.));
#21180=CARTESIAN_POINT('Ctrl Pts',(21.1452759244399,-34.2965325673384,15.));
#21181=CARTESIAN_POINT('Ctrl Pts',(21.2240487218078,-34.3560069185815,15.));
#21182=CARTESIAN_POINT('Ctrl Pts',(21.3033382073239,-34.4150300340623,15.));
#21183=CARTESIAN_POINT('Ctrl Pts',(21.3831361300104,-34.4736054662052,15.));
#21184=CARTESIAN_POINT('Ctrl Pts',(21.4634317666004,-34.5317385658329,15.));
#21185=CARTESIAN_POINT('Ctrl Pts',(21.5442132160757,-34.5894355639082,15.));
#21186=CARTESIAN_POINT('Ctrl Pts',(21.6254689009796,-34.6467025072367,15.));
#21187=CARTESIAN_POINT('Ctrl Pts',(21.7071892844497,-34.7035440429025,15.));
#21188=CARTESIAN_POINT('Ctrl Pts',(21.7893672401137,-34.7599631530844,15.));
#21189=CARTESIAN_POINT('Ctrl Pts',(21.8719971302817,-34.8159618014436,15.));
#21190=CARTESIAN_POINT('Ctrl Pts',(21.9550742217675,-34.8715413418101,15.));
#21191=CARTESIAN_POINT('Ctrl Pts',(22.0385940162683,-34.9267029879922,15.));
#21192=CARTESIAN_POINT('Ctrl Pts',(22.1225514798584,-34.9814483545602,15.));
#21193=CARTESIAN_POINT('Ctrl Pts',(22.2069408519232,-35.0357795922459,15.));
#21194=CARTESIAN_POINT('Ctrl Pts',(22.2917560356802,-35.0896991159359,15.));
#21195=CARTESIAN_POINT('Ctrl Pts',(22.3769908340843,-35.1432094422642,15.));
#21196=CARTESIAN_POINT('Ctrl Pts',(22.4626392230023,-35.1963130003353,15.));
#21197=CARTESIAN_POINT('Ctrl Pts',(22.5486956608909,-35.2490119207975,15.));
#21198=CARTESIAN_POINT('Ctrl Pts',(22.635155167154,-35.3013079759253,15.));
#21199=CARTESIAN_POINT('Ctrl Pts',(22.7220131336912,-35.3532026952313,15.));
#21200=CARTESIAN_POINT('Ctrl Pts',(22.8092652000706,-35.4046974393492,15.));
#21201=CARTESIAN_POINT('Ctrl Pts',(22.8969071125089,-35.4557934871468,15.));
#21202=CARTESIAN_POINT('Ctrl Pts',(22.9849345572033,-35.5064921357308,15.));
#21203=CARTESIAN_POINT('Ctrl Pts',(23.0733431097058,-35.5567947408311,15.));
#21204=CARTESIAN_POINT('Ctrl Pts',(23.1621283508111,-35.6067026687722,15.));
#21205=CARTESIAN_POINT('Ctrl Pts',(23.2512859425032,-35.6562172725207,15.));
#21206=CARTESIAN_POINT('Ctrl Pts',(23.3408117088761,-35.7053398620512,15.));
#21207=CARTESIAN_POINT('Ctrl Pts',(23.4307017328227,-35.7540716771372,15.));
#21208=CARTESIAN_POINT('Ctrl Pts',(23.5209523746427,-35.8024138716897,15.));
#21209=CARTESIAN_POINT('Ctrl Pts',(23.611560139948,-35.8503675222884,15.));
#21210=CARTESIAN_POINT('Ctrl Pts',(23.7025215735353,-35.8979336336837,15.));
#21211=CARTESIAN_POINT('Ctrl Pts',(23.7938331508737,-35.9451131482488,15.));
#21212=CARTESIAN_POINT('Ctrl Pts',(23.8854911428946,-35.991906956547,15.));
#21213=CARTESIAN_POINT('Ctrl Pts',(23.9774915680089,-36.0383159101253,15.));
#21214=CARTESIAN_POINT('Ctrl Pts',(24.0698304230588,-36.0843408347974,15.));
#21215=CARTESIAN_POINT('Ctrl Pts',(24.1625038657964,-36.1299825471271,15.));
#21216=CARTESIAN_POINT('Ctrl Pts',(24.2555084095331,-36.1752418704833,15.));
#21217=CARTESIAN_POINT('Ctrl Pts',(24.3488411214068,-36.2201196586696,15.));
#21218=CARTESIAN_POINT('Ctrl Pts',(24.4612315181511,-36.2735162352735,15.));
#21219=CARTESIAN_POINT('Ctrl Pts',(24.5552956307817,-36.3175386315529,15.));
#21220=CARTESIAN_POINT('Ctrl Pts',(24.630805301288,-36.3524534604649,15.));
#21221=CARTESIAN_POINT('Ctrl Pts',(24.6875827477483,-36.37846926509,15.));
#21222=CARTESIAN_POINT('Ctrl Pts',(24.725498909423,-36.3957374383337,15.));
#21223=CARTESIAN_POINT('Ctrl Pts',(14.911486495888,-41.396226524684,0.));
#21224=CARTESIAN_POINT('Ctrl Pts',(14.911486495888,-41.396226524684,18.));
#21225=CARTESIAN_POINT('Ctrl Pts',(14.9156446533966,-41.3758141263348,0.));
#21226=CARTESIAN_POINT('Ctrl Pts',(14.9156446533966,-41.3758141263348,18.));
#21227=CARTESIAN_POINT('Ctrl Pts',(14.9239113834707,-41.3349931861715,0.));
#21228=CARTESIAN_POINT('Ctrl Pts',(14.9239113834707,-41.3349931861715,18.));
#21229=CARTESIAN_POINT('Ctrl Pts',(14.936162723752,-41.2737733455422,0.));
#21230=CARTESIAN_POINT('Ctrl Pts',(14.936162723752,-41.2737733455422,18.));
#21231=CARTESIAN_POINT('Ctrl Pts',(14.9522002356298,-41.1921700381957,0.));
#21232=CARTESIAN_POINT('Ctrl Pts',(14.9522002356298,-41.1921700381957,18.));
#21233=CARTESIAN_POINT('Ctrl Pts',(14.9717503874227,-41.0902046498729,0.));
#21234=CARTESIAN_POINT('Ctrl Pts',(14.9717503874227,-41.0902046498729,18.));
#21235=CARTESIAN_POINT('Ctrl Pts',(14.9908026205824,-40.9882784321884,0.));
#21236=CARTESIAN_POINT('Ctrl Pts',(14.9908026205824,-40.9882784321884,18.));
#21237=CARTESIAN_POINT('Ctrl Pts',(15.0093553188655,-40.8863921801,0.));
#21238=CARTESIAN_POINT('Ctrl Pts',(15.0093553188655,-40.8863921801,18.));
#21239=CARTESIAN_POINT('Ctrl Pts',(15.0274064563211,-40.7845471608654,0.));
#21240=CARTESIAN_POINT('Ctrl Pts',(15.0274064563211,-40.7845471608654,18.));
#21241=CARTESIAN_POINT('Ctrl Pts',(15.0449536183143,-40.6827452453667,0.));
#21242=CARTESIAN_POINT('Ctrl Pts',(15.0449536183143,-40.6827452453667,18.));
#21243=CARTESIAN_POINT('Ctrl Pts',(15.0619940893017,-40.58098877043,0.));
#21244=CARTESIAN_POINT('Ctrl Pts',(15.0619940893017,-40.58098877043,18.));
#21245=CARTESIAN_POINT('Ctrl Pts',(15.0785249502524,-40.4792803645352,0.));
#21246=CARTESIAN_POINT('Ctrl Pts',(15.0785249502524,-40.4792803645352,18.));
#21247=CARTESIAN_POINT('Ctrl Pts',(15.0945431800723,-40.3776227809037,0.));
#21248=CARTESIAN_POINT('Ctrl Pts',(15.0945431800723,-40.3776227809037,18.));
#21249=CARTESIAN_POINT('Ctrl Pts',(15.1100457495259,-40.2760187401822,0.));
#21250=CARTESIAN_POINT('Ctrl Pts',(15.1100457495259,-40.2760187401822,18.));
#21251=CARTESIAN_POINT('Ctrl Pts',(15.1250297462408,-40.1744707357902,0.));
#21252=CARTESIAN_POINT('Ctrl Pts',(15.1250297462408,-40.1744707357902,18.));
#21253=CARTESIAN_POINT('Ctrl Pts',(15.1394923361537,-40.0729810652204,0.));
#21254=CARTESIAN_POINT('Ctrl Pts',(15.1394923361537,-40.0729810652204,18.));
#21255=CARTESIAN_POINT('Ctrl Pts',(15.1534306754871,-39.9715519332134,0.));
#21256=CARTESIAN_POINT('Ctrl Pts',(15.1534306754871,-39.9715519332134,18.));
#21257=CARTESIAN_POINT('Ctrl Pts',(15.1668418393198,-39.8701855339908,0.));
#21258=CARTESIAN_POINT('Ctrl Pts',(15.1668418393198,-39.8701855339908,18.));
#21259=CARTESIAN_POINT('Ctrl Pts',(15.1797227547561,-39.7688841338802,0.));
#21260=CARTESIAN_POINT('Ctrl Pts',(15.1797227547561,-39.7688841338802,18.));
#21261=CARTESIAN_POINT('Ctrl Pts',(15.1920701163803,-39.6676501731673,0.));
#21262=CARTESIAN_POINT('Ctrl Pts',(15.1920701163803,-39.6676501731673,18.));
#21263=CARTESIAN_POINT('Ctrl Pts',(15.2038804098649,-39.5664862602472,0.));
#21264=CARTESIAN_POINT('Ctrl Pts',(15.2038804098649,-39.5664862602472,18.));
#21265=CARTESIAN_POINT('Ctrl Pts',(15.2151499908149,-39.4653951093947,0.));
#21266=CARTESIAN_POINT('Ctrl Pts',(15.2151499908149,-39.4653951093947,18.));
#21267=CARTESIAN_POINT('Ctrl Pts',(15.2258751563069,-39.3643794927167,0.));
#21268=CARTESIAN_POINT('Ctrl Pts',(15.2258751563069,-39.3643794927167,18.));
#21269=CARTESIAN_POINT('Ctrl Pts',(15.2360522089072,-39.2634421927888,0.));
#21270=CARTESIAN_POINT('Ctrl Pts',(15.2360522089072,-39.2634421927888,18.));
#21271=CARTESIAN_POINT('Ctrl Pts',(15.2456775636447,-39.1625859371304,0.));
#21272=CARTESIAN_POINT('Ctrl Pts',(15.2456775636447,-39.1625859371304,18.));
#21273=CARTESIAN_POINT('Ctrl Pts',(15.2547476855825,-39.061813415425,0.));
#21274=CARTESIAN_POINT('Ctrl Pts',(15.2547476855825,-39.061813415425,18.));
#21275=CARTESIAN_POINT('Ctrl Pts',(15.2632589109473,-38.9611273555758,0.));
#21276=CARTESIAN_POINT('Ctrl Pts',(15.2632589109473,-38.9611273555758,18.));
#21277=CARTESIAN_POINT('Ctrl Pts',(15.2712072937639,-38.860530586589,0.));
#21278=CARTESIAN_POINT('Ctrl Pts',(15.2712072937639,-38.860530586589,18.));
#21279=CARTESIAN_POINT('Ctrl Pts',(15.2785884727112,-38.7600260961351,0.));
#21280=CARTESIAN_POINT('Ctrl Pts',(15.2785884727112,-38.7600260961351,18.));
#21281=CARTESIAN_POINT('Ctrl Pts',(15.2853974668211,-38.659617115053,0.));
#21282=CARTESIAN_POINT('Ctrl Pts',(15.2853974668211,-38.659617115053,18.));
#21283=CARTESIAN_POINT('Ctrl Pts',(15.2916287700102,-38.5593070891769,0.));
#21284=CARTESIAN_POINT('Ctrl Pts',(15.2916287700102,-38.5593070891769,18.));
#21285=CARTESIAN_POINT('Ctrl Pts',(15.2972767037469,-38.4590995527814,0.));
#21286=CARTESIAN_POINT('Ctrl Pts',(15.2972767037469,-38.4590995527814,18.));
#21287=CARTESIAN_POINT('Ctrl Pts',(15.3023357307483,-38.3589980188324,0.));
#21288=CARTESIAN_POINT('Ctrl Pts',(15.3023357307483,-38.3589980188324,18.));
#21289=CARTESIAN_POINT('Ctrl Pts',(15.3068007250314,-38.2590058835965,0.));
#21290=CARTESIAN_POINT('Ctrl Pts',(15.3068007250314,-38.2590058835965,18.));
#21291=CARTESIAN_POINT('Ctrl Pts',(15.310667421514,-38.1591262705847,0.));
#21292=CARTESIAN_POINT('Ctrl Pts',(15.310667421514,-38.1591262705847,18.));
#21293=CARTESIAN_POINT('Ctrl Pts',(15.3139321941687,-38.0593621055415,0.));
#21294=CARTESIAN_POINT('Ctrl Pts',(15.3139321941687,-38.0593621055415,18.));
#21295=CARTESIAN_POINT('Ctrl Pts',(15.3165911656268,-37.959716421934,0.));
#21296=CARTESIAN_POINT('Ctrl Pts',(15.3165911656268,-37.959716421934,18.));
#21297=CARTESIAN_POINT('Ctrl Pts',(15.3186394335023,-37.8601926265378,0.));
#21298=CARTESIAN_POINT('Ctrl Pts',(15.3186394335023,-37.8601926265378,18.));
#21299=CARTESIAN_POINT('Ctrl Pts',(15.320070396385,-37.7607947318286,0.));
#21300=CARTESIAN_POINT('Ctrl Pts',(15.320070396385,-37.7607947318286,18.));
#21301=CARTESIAN_POINT('Ctrl Pts',(15.320874689078,-37.6615277218027,0.));
#21302=CARTESIAN_POINT('Ctrl Pts',(15.320874689078,-37.6615277218027,18.));
#21303=CARTESIAN_POINT('Ctrl Pts',(15.3210406145546,-37.562397408596,0.));
#21304=CARTESIAN_POINT('Ctrl Pts',(15.3210406145546,-37.562397408596,18.));
#21305=CARTESIAN_POINT('Ctrl Pts',(15.3205561366169,-37.4634097578665,0.));
#21306=CARTESIAN_POINT('Ctrl Pts',(15.3205561366169,-37.4634097578665,18.));
#21307=CARTESIAN_POINT('Ctrl Pts',(15.3194106233801,-37.3645702997848,0.));
#21308=CARTESIAN_POINT('Ctrl Pts',(15.3194106233801,-37.3645702997848,18.));
#21309=CARTESIAN_POINT('Ctrl Pts',(15.3175963510697,-37.2658836214694,0.));
#21310=CARTESIAN_POINT('Ctrl Pts',(15.3175963510697,-37.2658836214694,18.));
#21311=CARTESIAN_POINT('Ctrl Pts',(15.3151109648809,-37.1673525354642,0.));
#21312=CARTESIAN_POINT('Ctrl Pts',(15.3151109648809,-37.1673525354642,18.));
#21313=CARTESIAN_POINT('Ctrl Pts',(15.3119562971444,-37.0689784837457,0.));
#21314=CARTESIAN_POINT('Ctrl Pts',(15.3119562971444,-37.0689784837457,18.));
#21315=CARTESIAN_POINT('Ctrl Pts',(15.3081335446406,-36.970763176802,0.));
#21316=CARTESIAN_POINT('Ctrl Pts',(15.3081335446406,-36.970763176802,18.));
#21317=CARTESIAN_POINT('Ctrl Pts',(15.3036390436952,-36.8727100302512,0.));
#21318=CARTESIAN_POINT('Ctrl Pts',(15.3036390436952,-36.8727100302512,18.));
#21319=CARTESIAN_POINT('Ctrl Pts',(15.2984606286737,-36.7748254044502,0.));
#21320=CARTESIAN_POINT('Ctrl Pts',(15.2984606286737,-36.7748254044502,18.));
#21321=CARTESIAN_POINT('Ctrl Pts',(15.2925717100767,-36.6771206167756,0.));
#21322=CARTESIAN_POINT('Ctrl Pts',(15.2925717100767,-36.6771206167756,18.));
#21323=CARTESIAN_POINT('Ctrl Pts',(15.2859343913094,-36.5796108931244,0.));
#21324=CARTESIAN_POINT('Ctrl Pts',(15.2859343913094,-36.5796108931244,18.));
#21325=CARTESIAN_POINT('Ctrl Pts',(15.2785104654792,-36.4823116513289,0.));
#21326=CARTESIAN_POINT('Ctrl Pts',(15.2785104654792,-36.4823116513289,18.));
#21327=CARTESIAN_POINT('Ctrl Pts',(15.2702711460936,-36.3852352131887,0.));
#21328=CARTESIAN_POINT('Ctrl Pts',(15.2702711460936,-36.3852352131887,18.));
#21329=CARTESIAN_POINT('Ctrl Pts',(15.2612053303773,-36.2883880151607,0.));
#21330=CARTESIAN_POINT('Ctrl Pts',(15.2612053303773,-36.2883880151607,18.));
#21331=CARTESIAN_POINT('Ctrl Pts',(15.2513334565427,-36.1917659216814,0.));
#21332=CARTESIAN_POINT('Ctrl Pts',(15.2513334565427,-36.1917659216814,18.));
#21333=CARTESIAN_POINT('Ctrl Pts',(15.240697754828,-36.095357546697,0.));
#21334=CARTESIAN_POINT('Ctrl Pts',(15.240697754828,-36.095357546697,18.));
#21335=CARTESIAN_POINT('Ctrl Pts',(15.2293360946131,-35.9991531408727,0.));
#21336=CARTESIAN_POINT('Ctrl Pts',(15.2293360946131,-35.9991531408727,18.));
#21337=CARTESIAN_POINT('Ctrl Pts',(15.2172585668056,-35.9031525499277,0.));
#21338=CARTESIAN_POINT('Ctrl Pts',(15.2172585668056,-35.9031525499277,18.));
#21339=CARTESIAN_POINT('Ctrl Pts',(15.2044274601769,-35.8073720252878,0.));
#21340=CARTESIAN_POINT('Ctrl Pts',(15.2044274601769,-35.8073720252878,18.));
#21341=CARTESIAN_POINT('Ctrl Pts',(15.1907243629658,-35.7118553943773,0.));
#21342=CARTESIAN_POINT('Ctrl Pts',(15.1907243629658,-35.7118553943773,18.));
#21343=CARTESIAN_POINT('Ctrl Pts',(15.1759785763051,-35.6166644736253,0.));
#21344=CARTESIAN_POINT('Ctrl Pts',(15.1759785763051,-35.6166644736253,18.));
#21345=CARTESIAN_POINT('Ctrl Pts',(15.1600260710383,-35.5218591529746,0.));
#21346=CARTESIAN_POINT('Ctrl Pts',(15.1600260710383,-35.5218591529746,18.));
#21347=CARTESIAN_POINT('Ctrl Pts',(15.1427632633831,-35.4274792115856,0.));
#21348=CARTESIAN_POINT('Ctrl Pts',(15.1427632633831,-35.4274792115856,18.));
#21349=CARTESIAN_POINT('Ctrl Pts',(15.1241934020681,-35.3335286891314,0.));
#21350=CARTESIAN_POINT('Ctrl Pts',(15.1241934020681,-35.3335286891314,18.));
#21351=CARTESIAN_POINT('Ctrl Pts',(15.104500806927,-35.2399506932815,0.));
#21352=CARTESIAN_POINT('Ctrl Pts',(15.104500806927,-35.2399506932815,18.));
#21353=CARTESIAN_POINT('Ctrl Pts',(15.08395927165,-35.1466591020976,0.));
#21354=CARTESIAN_POINT('Ctrl Pts',(15.08395927165,-35.1466591020976,18.));
#21355=CARTESIAN_POINT('Ctrl Pts',(15.0627878528202,-35.0535882932913,0.));
#21356=CARTESIAN_POINT('Ctrl Pts',(15.0627878528202,-35.0535882932913,18.));
#21357=CARTESIAN_POINT('Ctrl Pts',(15.041018569143,-34.9607388363587,0.));
#21358=CARTESIAN_POINT('Ctrl Pts',(15.041018569143,-34.9607388363587,18.));
#21359=CARTESIAN_POINT('Ctrl Pts',(15.0183713484962,-34.8682205930809,0.));
#21360=CARTESIAN_POINT('Ctrl Pts',(15.0183713484962,-34.8682205930809,18.));
#21361=CARTESIAN_POINT('Ctrl Pts',(14.9940927023321,-34.7763085406486,0.));
#21362=CARTESIAN_POINT('Ctrl Pts',(14.9940927023321,-34.7763085406486,18.));
#21363=CARTESIAN_POINT('Ctrl Pts',(14.9671565602316,-34.6853717911268,0.));
#21364=CARTESIAN_POINT('Ctrl Pts',(14.9671565602316,-34.6853717911268,18.));
#21365=CARTESIAN_POINT('Ctrl Pts',(14.9426481276593,-34.6137007885254,0.));
#21366=CARTESIAN_POINT('Ctrl Pts',(14.9426481276593,-34.6137007885254,18.));
#21367=CARTESIAN_POINT('Ctrl Pts',(14.9222326355678,-34.5606858566713,0.));
#21368=CARTESIAN_POINT('Ctrl Pts',(14.9222326355678,-34.5606858566713,18.));
#21369=CARTESIAN_POINT('Ctrl Pts',(14.9076710061311,-34.525687510388,0.));
#21370=CARTESIAN_POINT('Ctrl Pts',(14.9076710061311,-34.525687510388,18.));
#21371=CARTESIAN_POINT('Ctrl Pts',(14.9001523628048,-34.5082745737944,0.));
#21372=CARTESIAN_POINT('Ctrl Pts',(14.9001523628048,-34.5082745737944,18.));
#21373=CARTESIAN_POINT('',(14.9114864958881,-41.3962265246839,0.));
#21374=CARTESIAN_POINT('Ctrl Pts',(14.9001523628048,-34.5082745737944,0.));
#21375=CARTESIAN_POINT('Ctrl Pts',(14.9076710061311,-34.525687510388,0.));
#21376=CARTESIAN_POINT('Ctrl Pts',(14.9222326355678,-34.5606858566713,0.));
#21377=CARTESIAN_POINT('Ctrl Pts',(14.9426481276593,-34.6137007885254,0.));
#21378=CARTESIAN_POINT('Ctrl Pts',(14.9671565602316,-34.6853717911268,0.));
#21379=CARTESIAN_POINT('Ctrl Pts',(14.9940927023321,-34.7763085406486,0.));
#21380=CARTESIAN_POINT('Ctrl Pts',(15.0183713484962,-34.8682205930809,0.));
#21381=CARTESIAN_POINT('Ctrl Pts',(15.041018569143,-34.9607388363587,0.));
#21382=CARTESIAN_POINT('Ctrl Pts',(15.0627878528202,-35.0535882932913,0.));
#21383=CARTESIAN_POINT('Ctrl Pts',(15.08395927165,-35.1466591020976,0.));
#21384=CARTESIAN_POINT('Ctrl Pts',(15.104500806927,-35.2399506932815,0.));
#21385=CARTESIAN_POINT('Ctrl Pts',(15.1241934020681,-35.3335286891314,0.));
#21386=CARTESIAN_POINT('Ctrl Pts',(15.1427632633831,-35.4274792115856,0.));
#21387=CARTESIAN_POINT('Ctrl Pts',(15.1600260710383,-35.5218591529746,0.));
#21388=CARTESIAN_POINT('Ctrl Pts',(15.1759785763051,-35.6166644736253,0.));
#21389=CARTESIAN_POINT('Ctrl Pts',(15.1907243629658,-35.7118553943773,0.));
#21390=CARTESIAN_POINT('Ctrl Pts',(15.2044274601769,-35.8073720252878,0.));
#21391=CARTESIAN_POINT('Ctrl Pts',(15.2172585668056,-35.9031525499277,0.));
#21392=CARTESIAN_POINT('Ctrl Pts',(15.2293360946131,-35.9991531408727,0.));
#21393=CARTESIAN_POINT('Ctrl Pts',(15.240697754828,-36.095357546697,0.));
#21394=CARTESIAN_POINT('Ctrl Pts',(15.2513334565427,-36.1917659216814,0.));
#21395=CARTESIAN_POINT('Ctrl Pts',(15.2612053303773,-36.2883880151607,0.));
#21396=CARTESIAN_POINT('Ctrl Pts',(15.2702711460936,-36.3852352131887,0.));
#21397=CARTESIAN_POINT('Ctrl Pts',(15.2785104654792,-36.4823116513289,0.));
#21398=CARTESIAN_POINT('Ctrl Pts',(15.2859343913094,-36.5796108931244,0.));
#21399=CARTESIAN_POINT('Ctrl Pts',(15.2925717100767,-36.6771206167756,0.));
#21400=CARTESIAN_POINT('Ctrl Pts',(15.2984606286737,-36.7748254044502,0.));
#21401=CARTESIAN_POINT('Ctrl Pts',(15.3036390436952,-36.8727100302512,0.));
#21402=CARTESIAN_POINT('Ctrl Pts',(15.3081335446406,-36.970763176802,0.));
#21403=CARTESIAN_POINT('Ctrl Pts',(15.3119562971444,-37.0689784837457,0.));
#21404=CARTESIAN_POINT('Ctrl Pts',(15.3151109648809,-37.1673525354642,0.));
#21405=CARTESIAN_POINT('Ctrl Pts',(15.3175963510697,-37.2658836214694,0.));
#21406=CARTESIAN_POINT('Ctrl Pts',(15.3194106233801,-37.3645702997848,0.));
#21407=CARTESIAN_POINT('Ctrl Pts',(15.3205561366169,-37.4634097578665,0.));
#21408=CARTESIAN_POINT('Ctrl Pts',(15.3210406145546,-37.562397408596,0.));
#21409=CARTESIAN_POINT('Ctrl Pts',(15.320874689078,-37.6615277218027,0.));
#21410=CARTESIAN_POINT('Ctrl Pts',(15.320070396385,-37.7607947318286,0.));
#21411=CARTESIAN_POINT('Ctrl Pts',(15.3186394335023,-37.8601926265378,0.));
#21412=CARTESIAN_POINT('Ctrl Pts',(15.3165911656268,-37.959716421934,0.));
#21413=CARTESIAN_POINT('Ctrl Pts',(15.3139321941687,-38.0593621055415,0.));
#21414=CARTESIAN_POINT('Ctrl Pts',(15.310667421514,-38.1591262705847,0.));
#21415=CARTESIAN_POINT('Ctrl Pts',(15.3068007250314,-38.2590058835965,0.));
#21416=CARTESIAN_POINT('Ctrl Pts',(15.3023357307483,-38.3589980188324,0.));
#21417=CARTESIAN_POINT('Ctrl Pts',(15.2972767037469,-38.4590995527814,0.));
#21418=CARTESIAN_POINT('Ctrl Pts',(15.2916287700102,-38.5593070891769,0.));
#21419=CARTESIAN_POINT('Ctrl Pts',(15.2853974668211,-38.659617115053,0.));
#21420=CARTESIAN_POINT('Ctrl Pts',(15.2785884727112,-38.7600260961351,0.));
#21421=CARTESIAN_POINT('Ctrl Pts',(15.2712072937639,-38.860530586589,0.));
#21422=CARTESIAN_POINT('Ctrl Pts',(15.2632589109473,-38.9611273555758,0.));
#21423=CARTESIAN_POINT('Ctrl Pts',(15.2547476855825,-39.061813415425,0.));
#21424=CARTESIAN_POINT('Ctrl Pts',(15.2456775636447,-39.1625859371304,0.));
#21425=CARTESIAN_POINT('Ctrl Pts',(15.2360522089072,-39.2634421927888,0.));
#21426=CARTESIAN_POINT('Ctrl Pts',(15.2258751563069,-39.3643794927167,0.));
#21427=CARTESIAN_POINT('Ctrl Pts',(15.2151499908149,-39.4653951093947,0.));
#21428=CARTESIAN_POINT('Ctrl Pts',(15.2038804098649,-39.5664862602472,0.));
#21429=CARTESIAN_POINT('Ctrl Pts',(15.1920701163803,-39.6676501731673,0.));
#21430=CARTESIAN_POINT('Ctrl Pts',(15.1797227547561,-39.7688841338802,0.));
#21431=CARTESIAN_POINT('Ctrl Pts',(15.1668418393198,-39.8701855339908,0.));
#21432=CARTESIAN_POINT('Ctrl Pts',(15.1534306754871,-39.9715519332134,0.));
#21433=CARTESIAN_POINT('Ctrl Pts',(15.1394923361537,-40.0729810652204,0.));
#21434=CARTESIAN_POINT('Ctrl Pts',(15.1250297462408,-40.1744707357902,0.));
#21435=CARTESIAN_POINT('Ctrl Pts',(15.1100457495259,-40.2760187401822,0.));
#21436=CARTESIAN_POINT('Ctrl Pts',(15.0945431800723,-40.3776227809037,0.));
#21437=CARTESIAN_POINT('Ctrl Pts',(15.0785249502524,-40.4792803645352,0.));
#21438=CARTESIAN_POINT('Ctrl Pts',(15.0619940893017,-40.58098877043,0.));
#21439=CARTESIAN_POINT('Ctrl Pts',(15.0449536183143,-40.6827452453667,0.));
#21440=CARTESIAN_POINT('Ctrl Pts',(15.0274064563211,-40.7845471608654,0.));
#21441=CARTESIAN_POINT('Ctrl Pts',(15.0093553188655,-40.8863921801,0.));
#21442=CARTESIAN_POINT('Ctrl Pts',(14.9908026205824,-40.9882784321884,0.));
#21443=CARTESIAN_POINT('Ctrl Pts',(14.9679399407908,-41.1105898934098,0.));
#21444=CARTESIAN_POINT('Ctrl Pts',(14.9482653093396,-41.2125650743922,0.));
#21445=CARTESIAN_POINT('Ctrl Pts',(14.9321285285561,-41.2941761025922,0.));
#21446=CARTESIAN_POINT('Ctrl Pts',(14.919802810928,-41.3554017279611,0.));
#21447=CARTESIAN_POINT('Ctrl Pts',(14.911486495888,-41.396226524684,0.));
#21448=CARTESIAN_POINT('',(14.9114864958881,-41.3962265246839,15.));
#21449=CARTESIAN_POINT('Ctrl Pts',(14.911486495888,-41.396226524684,15.));
#21450=CARTESIAN_POINT('Ctrl Pts',(14.9156446533966,-41.3758141263348,15.));
#21451=CARTESIAN_POINT('Ctrl Pts',(14.9239113834707,-41.3349931861715,15.));
#21452=CARTESIAN_POINT('Ctrl Pts',(14.936162723752,-41.2737733455422,15.));
#21453=CARTESIAN_POINT('Ctrl Pts',(14.9522002356298,-41.1921700381957,15.));
#21454=CARTESIAN_POINT('Ctrl Pts',(14.9717503874227,-41.0902046498729,15.));
#21455=CARTESIAN_POINT('Ctrl Pts',(14.9908026205824,-40.9882784321884,15.));
#21456=CARTESIAN_POINT('Ctrl Pts',(15.0093553188655,-40.8863921801,15.));
#21457=CARTESIAN_POINT('Ctrl Pts',(15.0274064563211,-40.7845471608654,15.));
#21458=CARTESIAN_POINT('Ctrl Pts',(15.0449536183143,-40.6827452453667,15.));
#21459=CARTESIAN_POINT('Ctrl Pts',(15.0619940893017,-40.58098877043,15.));
#21460=CARTESIAN_POINT('Ctrl Pts',(15.0785249502524,-40.4792803645352,15.));
#21461=CARTESIAN_POINT('Ctrl Pts',(15.0945431800723,-40.3776227809037,15.));
#21462=CARTESIAN_POINT('Ctrl Pts',(15.1100457495259,-40.2760187401822,15.));
#21463=CARTESIAN_POINT('Ctrl Pts',(15.1250297462408,-40.1744707357902,15.));
#21464=CARTESIAN_POINT('Ctrl Pts',(15.1394923361537,-40.0729810652204,15.));
#21465=CARTESIAN_POINT('Ctrl Pts',(15.1534306754871,-39.9715519332134,15.));
#21466=CARTESIAN_POINT('Ctrl Pts',(15.1668418393198,-39.8701855339908,15.));
#21467=CARTESIAN_POINT('Ctrl Pts',(15.1797227547561,-39.7688841338802,15.));
#21468=CARTESIAN_POINT('Ctrl Pts',(15.1920701163803,-39.6676501731673,15.));
#21469=CARTESIAN_POINT('Ctrl Pts',(15.2038804098649,-39.5664862602472,15.));
#21470=CARTESIAN_POINT('Ctrl Pts',(15.2151499908149,-39.4653951093947,15.));
#21471=CARTESIAN_POINT('Ctrl Pts',(15.2258751563069,-39.3643794927167,15.));
#21472=CARTESIAN_POINT('Ctrl Pts',(15.2360522089072,-39.2634421927888,15.));
#21473=CARTESIAN_POINT('Ctrl Pts',(15.2456775636447,-39.1625859371304,15.));
#21474=CARTESIAN_POINT('Ctrl Pts',(15.2547476855825,-39.061813415425,15.));
#21475=CARTESIAN_POINT('Ctrl Pts',(15.2632589109473,-38.9611273555758,15.));
#21476=CARTESIAN_POINT('Ctrl Pts',(15.2712072937639,-38.860530586589,15.));
#21477=CARTESIAN_POINT('Ctrl Pts',(15.2785884727112,-38.7600260961351,15.));
#21478=CARTESIAN_POINT('Ctrl Pts',(15.2853974668211,-38.659617115053,15.));
#21479=CARTESIAN_POINT('Ctrl Pts',(15.2916287700102,-38.5593070891769,15.));
#21480=CARTESIAN_POINT('Ctrl Pts',(15.2972767037469,-38.4590995527814,15.));
#21481=CARTESIAN_POINT('Ctrl Pts',(15.3023357307483,-38.3589980188324,15.));
#21482=CARTESIAN_POINT('Ctrl Pts',(15.3068007250314,-38.2590058835965,15.));
#21483=CARTESIAN_POINT('Ctrl Pts',(15.310667421514,-38.1591262705847,15.));
#21484=CARTESIAN_POINT('Ctrl Pts',(15.3139321941687,-38.0593621055415,15.));
#21485=CARTESIAN_POINT('Ctrl Pts',(15.3165911656268,-37.959716421934,15.));
#21486=CARTESIAN_POINT('Ctrl Pts',(15.3186394335023,-37.8601926265378,15.));
#21487=CARTESIAN_POINT('Ctrl Pts',(15.320070396385,-37.7607947318286,15.));
#21488=CARTESIAN_POINT('Ctrl Pts',(15.320874689078,-37.6615277218027,15.));
#21489=CARTESIAN_POINT('Ctrl Pts',(15.3210406145546,-37.562397408596,15.));
#21490=CARTESIAN_POINT('Ctrl Pts',(15.3205561366169,-37.4634097578665,15.));
#21491=CARTESIAN_POINT('Ctrl Pts',(15.3194106233801,-37.3645702997848,15.));
#21492=CARTESIAN_POINT('Ctrl Pts',(15.3175963510697,-37.2658836214694,15.));
#21493=CARTESIAN_POINT('Ctrl Pts',(15.3151109648809,-37.1673525354642,15.));
#21494=CARTESIAN_POINT('Ctrl Pts',(15.3119562971444,-37.0689784837457,15.));
#21495=CARTESIAN_POINT('Ctrl Pts',(15.3081335446406,-36.970763176802,15.));
#21496=CARTESIAN_POINT('Ctrl Pts',(15.3036390436952,-36.8727100302512,15.));
#21497=CARTESIAN_POINT('Ctrl Pts',(15.2984606286737,-36.7748254044502,15.));
#21498=CARTESIAN_POINT('Ctrl Pts',(15.2925717100767,-36.6771206167756,15.));
#21499=CARTESIAN_POINT('Ctrl Pts',(15.2859343913094,-36.5796108931244,15.));
#21500=CARTESIAN_POINT('Ctrl Pts',(15.2785104654792,-36.4823116513289,15.));
#21501=CARTESIAN_POINT('Ctrl Pts',(15.2702711460936,-36.3852352131887,15.));
#21502=CARTESIAN_POINT('Ctrl Pts',(15.2612053303773,-36.2883880151607,15.));
#21503=CARTESIAN_POINT('Ctrl Pts',(15.2513334565427,-36.1917659216814,15.));
#21504=CARTESIAN_POINT('Ctrl Pts',(15.240697754828,-36.095357546697,15.));
#21505=CARTESIAN_POINT('Ctrl Pts',(15.2293360946131,-35.9991531408727,15.));
#21506=CARTESIAN_POINT('Ctrl Pts',(15.2172585668056,-35.9031525499277,15.));
#21507=CARTESIAN_POINT('Ctrl Pts',(15.2044274601769,-35.8073720252878,15.));
#21508=CARTESIAN_POINT('Ctrl Pts',(15.1907243629658,-35.7118553943773,15.));
#21509=CARTESIAN_POINT('Ctrl Pts',(15.1759785763051,-35.6166644736253,15.));
#21510=CARTESIAN_POINT('Ctrl Pts',(15.1600260710383,-35.5218591529746,15.));
#21511=CARTESIAN_POINT('Ctrl Pts',(15.1427632633831,-35.4274792115856,15.));
#21512=CARTESIAN_POINT('Ctrl Pts',(15.1241934020681,-35.3335286891314,15.));
#21513=CARTESIAN_POINT('Ctrl Pts',(15.104500806927,-35.2399506932815,15.));
#21514=CARTESIAN_POINT('Ctrl Pts',(15.08395927165,-35.1466591020976,15.));
#21515=CARTESIAN_POINT('Ctrl Pts',(15.0627878528202,-35.0535882932913,15.));
#21516=CARTESIAN_POINT('Ctrl Pts',(15.041018569143,-34.9607388363587,15.));
#21517=CARTESIAN_POINT('Ctrl Pts',(15.0183713484962,-34.8682205930809,15.));
#21518=CARTESIAN_POINT('Ctrl Pts',(14.9940927023321,-34.7763085406486,15.));
#21519=CARTESIAN_POINT('Ctrl Pts',(14.9671565602316,-34.6853717911268,15.));
#21520=CARTESIAN_POINT('Ctrl Pts',(14.9426481276593,-34.6137007885254,15.));
#21521=CARTESIAN_POINT('Ctrl Pts',(14.9222326355678,-34.5606858566713,15.));
#21522=CARTESIAN_POINT('Ctrl Pts',(14.9076710061311,-34.525687510388,15.));
#21523=CARTESIAN_POINT('Ctrl Pts',(14.9001523628048,-34.5082745737944,15.));
#21524=CARTESIAN_POINT('',(14.9114864958881,-41.3962265246839,0.));
#21525=CARTESIAN_POINT('Origin',(3.50213800024364E-12,-1.07784724682657E-11,
0.));
#21526=CARTESIAN_POINT('',(12.2684454652018,-42.2550026135057,0.));
#21527=CARTESIAN_POINT('Origin',(3.50213800024364E-12,-1.07784724682657E-11,
0.));
#21528=CARTESIAN_POINT('',(12.2684454652018,-42.2550026135057,15.));
#21529=CARTESIAN_POINT('Origin',(3.50213800024364E-12,-1.07784724682657E-11,
15.));
#21530=CARTESIAN_POINT('',(12.2684454652018,-42.2550026135057,0.));
#21531=CARTESIAN_POINT('Ctrl Pts',(8.2289783962506,-36.6758703925241,0.));
#21532=CARTESIAN_POINT('Ctrl Pts',(8.2289783962506,-36.6758703925241,18.));
#21533=CARTESIAN_POINT('Ctrl Pts',(8.23313075335376,-36.6943771018148,0.));
#21534=CARTESIAN_POINT('Ctrl Pts',(8.23313075335376,-36.6943771018148,18.));
#21535=CARTESIAN_POINT('Ctrl Pts',(8.24192165947366,-36.7312504697652,0.));
#21536=CARTESIAN_POINT('Ctrl Pts',(8.24192165947366,-36.7312504697652,18.));
#21537=CARTESIAN_POINT('Ctrl Pts',(8.2565665745182,-36.7861403757604,0.));
#21538=CARTESIAN_POINT('Ctrl Pts',(8.2565665745182,-36.7861403757604,18.));
#21539=CARTESIAN_POINT('Ctrl Pts',(8.27886599440784,-36.8585291300917,0.));
#21540=CARTESIAN_POINT('Ctrl Pts',(8.27886599440784,-36.8585291300917,18.));
#21541=CARTESIAN_POINT('Ctrl Pts',(8.3105254779459,-36.9479311729484,0.));
#21542=CARTESIAN_POINT('Ctrl Pts',(8.3105254779459,-36.9479311729484,18.));
#21543=CARTESIAN_POINT('Ctrl Pts',(8.34490818952639,-37.0365602155148,0.));
#21544=CARTESIAN_POINT('Ctrl Pts',(8.34490818952639,-37.0365602155148,18.));
#21545=CARTESIAN_POINT('Ctrl Pts',(8.38096706211447,-37.1247207489179,0.));
#21546=CARTESIAN_POINT('Ctrl Pts',(8.38096706211447,-37.1247207489179,18.));
#21547=CARTESIAN_POINT('Ctrl Pts',(8.41793088313259,-37.2126332013933,0.));
#21548=CARTESIAN_POINT('Ctrl Pts',(8.41793088313259,-37.2126332013933,18.));
#21549=CARTESIAN_POINT('Ctrl Pts',(8.45550849433959,-37.3003733151561,0.));
#21550=CARTESIAN_POINT('Ctrl Pts',(8.45550849433959,-37.3003733151561,18.));
#21551=CARTESIAN_POINT('Ctrl Pts',(8.49372546467075,-37.3879218093514,0.));
#21552=CARTESIAN_POINT('Ctrl Pts',(8.49372546467075,-37.3879218093514,18.));
#21553=CARTESIAN_POINT('Ctrl Pts',(8.53279758643783,-37.4752030152968,0.));
#21554=CARTESIAN_POINT('Ctrl Pts',(8.53279758643783,-37.4752030152968,18.));
#21555=CARTESIAN_POINT('Ctrl Pts',(8.57299698459465,-37.5621256752108,0.));
#21556=CARTESIAN_POINT('Ctrl Pts',(8.57299698459465,-37.5621256752108,18.));
#21557=CARTESIAN_POINT('Ctrl Pts',(8.61450621749154,-37.6486274754754,0.));
#21558=CARTESIAN_POINT('Ctrl Pts',(8.61450621749154,-37.6486274754754,18.));
#21559=CARTESIAN_POINT('Ctrl Pts',(8.65732553894524,-37.7347032383719,0.));
#21560=CARTESIAN_POINT('Ctrl Pts',(8.65732553894524,-37.7347032383719,18.));
#21561=CARTESIAN_POINT('Ctrl Pts',(8.70134776631143,-37.8203816669031,0.));
#21562=CARTESIAN_POINT('Ctrl Pts',(8.70134776631143,-37.8203816669031,18.));
#21563=CARTESIAN_POINT('Ctrl Pts',(8.74640499479001,-37.9057107230066,0.));
#21564=CARTESIAN_POINT('Ctrl Pts',(8.74640499479001,-37.9057107230066,18.));
#21565=CARTESIAN_POINT('Ctrl Pts',(8.79232279131091,-37.9907407304174,0.));
#21566=CARTESIAN_POINT('Ctrl Pts',(8.79232279131091,-37.9907407304174,18.));
#21567=CARTESIAN_POINT('Ctrl Pts',(8.83897959763348,-38.0755058326913,0.));
#21568=CARTESIAN_POINT('Ctrl Pts',(8.83897959763348,-38.0755058326913,18.));
#21569=CARTESIAN_POINT('Ctrl Pts',(8.88633535238434,-38.1600150482528,0.));
#21570=CARTESIAN_POINT('Ctrl Pts',(8.88633535238434,-38.1600150482528,18.));
#21571=CARTESIAN_POINT('Ctrl Pts',(8.93439830996338,-38.2442625706309,0.));
#21572=CARTESIAN_POINT('Ctrl Pts',(8.93439830996338,-38.2442625706309,18.));
#21573=CARTESIAN_POINT('Ctrl Pts',(8.98320483785759,-38.3282340281403,0.));
#21574=CARTESIAN_POINT('Ctrl Pts',(8.98320483785759,-38.3282340281403,18.));
#21575=CARTESIAN_POINT('Ctrl Pts',(9.0327957936019,-38.4119138099805,0.));
#21576=CARTESIAN_POINT('Ctrl Pts',(9.0327957936019,-38.4119138099805,18.));
#21577=CARTESIAN_POINT('Ctrl Pts',(9.08319014288085,-38.4952932486131,0.));
#21578=CARTESIAN_POINT('Ctrl Pts',(9.08319014288085,-38.4952932486131,18.));
#21579=CARTESIAN_POINT('Ctrl Pts',(9.13437512010585,-38.5783736628826,0.));
#21580=CARTESIAN_POINT('Ctrl Pts',(9.13437512010585,-38.5783736628826,18.));
#21581=CARTESIAN_POINT('Ctrl Pts',(9.18632019394329,-38.6611620045193,0.));
#21582=CARTESIAN_POINT('Ctrl Pts',(9.18632019394329,-38.6611620045193,18.));
#21583=CARTESIAN_POINT('Ctrl Pts',(9.2389853919933,-38.7436682576832,0.));
#21584=CARTESIAN_POINT('Ctrl Pts',(9.2389853919933,-38.7436682576832,18.));
#21585=CARTESIAN_POINT('Ctrl Pts',(9.29233110570902,-38.8259023794241,0.));
#21586=CARTESIAN_POINT('Ctrl Pts',(9.29233110570902,-38.8259023794241,18.));
#21587=CARTESIAN_POINT('Ctrl Pts',(9.34632917154636,-38.9078708427078,0.));
#21588=CARTESIAN_POINT('Ctrl Pts',(9.34632917154636,-38.9078708427078,18.));
#21589=CARTESIAN_POINT('Ctrl Pts',(9.40096600877643,-38.9895756526779,0.));
#21590=CARTESIAN_POINT('Ctrl Pts',(9.40096600877643,-38.9895756526779,18.));
#21591=CARTESIAN_POINT('Ctrl Pts',(9.45623664577431,-39.0710161994951,0.));
#21592=CARTESIAN_POINT('Ctrl Pts',(9.45623664577431,-39.0710161994951,18.));
#21593=CARTESIAN_POINT('Ctrl Pts',(9.5121410453562,-39.1521903958955,0.));
#21594=CARTESIAN_POINT('Ctrl Pts',(9.5121410453562,-39.1521903958955,18.));
#21595=CARTESIAN_POINT('Ctrl Pts',(9.56867984233622,-39.2330959982788,0.));
#21596=CARTESIAN_POINT('Ctrl Pts',(9.56867984233622,-39.2330959982788,18.));
#21597=CARTESIAN_POINT('Ctrl Pts',(9.62584947846542,-39.3137321153686,0.));
#21598=CARTESIAN_POINT('Ctrl Pts',(9.62584947846542,-39.3137321153686,18.));
#21599=CARTESIAN_POINT('Ctrl Pts',(9.68364100883825,-39.3940995760289,0.));
#21600=CARTESIAN_POINT('Ctrl Pts',(9.68364100883825,-39.3940995760289,18.));
#21601=CARTESIAN_POINT('Ctrl Pts',(9.74204258152662,-39.4742001555227,0.));
#21602=CARTESIAN_POINT('Ctrl Pts',(9.74204258152662,-39.4742001555227,18.));
#21603=CARTESIAN_POINT('Ctrl Pts',(9.80104095251613,-39.5540361022309,0.));
#21604=CARTESIAN_POINT('Ctrl Pts',(9.80104095251613,-39.5540361022309,18.));
#21605=CARTESIAN_POINT('Ctrl Pts',(9.86062324242559,-39.6336095893767,0.));
#21606=CARTESIAN_POINT('Ctrl Pts',(9.86062324242559,-39.6336095893767,18.));
#21607=CARTESIAN_POINT('Ctrl Pts',(9.92077894513191,-39.712922089547,0.));
#21608=CARTESIAN_POINT('Ctrl Pts',(9.92077894513191,-39.712922089547,18.));
#21609=CARTESIAN_POINT('Ctrl Pts',(9.98150036150822,-39.7919742367922,0.));
#21610=CARTESIAN_POINT('Ctrl Pts',(9.98150036150822,-39.7919742367922,18.));
#21611=CARTESIAN_POINT('Ctrl Pts',(10.0427815229883,-39.8707661565233,0.));
#21612=CARTESIAN_POINT('Ctrl Pts',(10.0427815229883,-39.8707661565233,18.));
#21613=CARTESIAN_POINT('Ctrl Pts',(10.1046175096878,-39.9492976736738,0.));
#21614=CARTESIAN_POINT('Ctrl Pts',(10.1046175096878,-39.9492976736738,18.));
#21615=CARTESIAN_POINT('Ctrl Pts',(10.1670036683795,-40.0275685525923,0.));
#21616=CARTESIAN_POINT('Ctrl Pts',(10.1670036683795,-40.0275685525923,18.));
#21617=CARTESIAN_POINT('Ctrl Pts',(10.2299347125857,-40.1055787732578,0.));
#21618=CARTESIAN_POINT('Ctrl Pts',(10.2299347125857,-40.1055787732578,18.));
#21619=CARTESIAN_POINT('Ctrl Pts',(10.2934044990237,-40.1833286010098,0.));
#21620=CARTESIAN_POINT('Ctrl Pts',(10.2934044990237,-40.1833286010098,18.));
#21621=CARTESIAN_POINT('Ctrl Pts',(10.3574064830678,-40.2608184485326,0.));
#21622=CARTESIAN_POINT('Ctrl Pts',(10.3574064830678,-40.2608184485326,18.));
#21623=CARTESIAN_POINT('Ctrl Pts',(10.421933993295,-40.3380487942952,0.));
#21624=CARTESIAN_POINT('Ctrl Pts',(10.421933993295,-40.3380487942952,18.));
#21625=CARTESIAN_POINT('Ctrl Pts',(10.48698054978,-40.4150200869536,0.));
#21626=CARTESIAN_POINT('Ctrl Pts',(10.48698054978,-40.4150200869536,18.));
#21627=CARTESIAN_POINT('Ctrl Pts',(10.552540223795,-40.4917326404439,0.));
#21628=CARTESIAN_POINT('Ctrl Pts',(10.552540223795,-40.4917326404439,18.));
#21629=CARTESIAN_POINT('Ctrl Pts',(10.618607730849,-40.5681866012103,0.));
#21630=CARTESIAN_POINT('Ctrl Pts',(10.618607730849,-40.5681866012103,18.));
#21631=CARTESIAN_POINT('Ctrl Pts',(10.6851782157325,-40.6443819999244,0.));
#21632=CARTESIAN_POINT('Ctrl Pts',(10.6851782157325,-40.6443819999244,18.));
#21633=CARTESIAN_POINT('Ctrl Pts',(10.7522471109694,-40.7203187831783,0.));
#21634=CARTESIAN_POINT('Ctrl Pts',(10.7522471109694,-40.7203187831783,18.));
#21635=CARTESIAN_POINT('Ctrl Pts',(10.8198099757795,-40.7959968527561,0.));
#21636=CARTESIAN_POINT('Ctrl Pts',(10.8198099757795,-40.7959968527561,18.));
#21637=CARTESIAN_POINT('Ctrl Pts',(10.8878623066646,-40.8714161092412,0.));
#21638=CARTESIAN_POINT('Ctrl Pts',(10.8878623066646,-40.8714161092412,18.));
#21639=CARTESIAN_POINT('Ctrl Pts',(10.956399476781,-40.9465764747798,0.));
#21640=CARTESIAN_POINT('Ctrl Pts',(10.956399476781,-40.9465764747798,18.));
#21641=CARTESIAN_POINT('Ctrl Pts',(11.0254168609972,-41.0214778832142,0.));
#21642=CARTESIAN_POINT('Ctrl Pts',(11.0254168609972,-41.0214778832142,18.));
#21643=CARTESIAN_POINT('Ctrl Pts',(11.0949099155251,-41.0961202807715,0.));
#21644=CARTESIAN_POINT('Ctrl Pts',(11.0949099155251,-41.0961202807715,18.));
#21645=CARTESIAN_POINT('Ctrl Pts',(11.1648742640378,-41.1705036228854,0.));
#21646=CARTESIAN_POINT('Ctrl Pts',(11.1648742640378,-41.1705036228854,18.));
#21647=CARTESIAN_POINT('Ctrl Pts',(11.2353057980338,-41.2446278781981,0.));
#21648=CARTESIAN_POINT('Ctrl Pts',(11.2353057980338,-41.2446278781981,18.));
#21649=CARTESIAN_POINT('Ctrl Pts',(11.3062006993745,-41.3184930194148,0.));
#21650=CARTESIAN_POINT('Ctrl Pts',(11.3062006993745,-41.3184930194148,18.));
#21651=CARTESIAN_POINT('Ctrl Pts',(11.3775553120176,-41.3920989905986,0.));
#21652=CARTESIAN_POINT('Ctrl Pts',(11.3775553120176,-41.3920989905986,18.));
#21653=CARTESIAN_POINT('Ctrl Pts',(11.4493660393849,-41.4654456796071,0.));
#21654=CARTESIAN_POINT('Ctrl Pts',(11.4493660393849,-41.4654456796071,18.));
#21655=CARTESIAN_POINT('Ctrl Pts',(11.5216292382388,-41.5385328935506,0.));
#21656=CARTESIAN_POINT('Ctrl Pts',(11.5216292382388,-41.5385328935506,18.));
#21657=CARTESIAN_POINT('Ctrl Pts',(11.5943410868252,-41.6113603270596,0.));
#21658=CARTESIAN_POINT('Ctrl Pts',(11.5943410868252,-41.6113603270596,18.));
#21659=CARTESIAN_POINT('Ctrl Pts',(11.6674975352851,-41.6839275596248,0.));
#21660=CARTESIAN_POINT('Ctrl Pts',(11.6674975352851,-41.6839275596248,18.));
#21661=CARTESIAN_POINT('Ctrl Pts',(11.7410945211992,-41.7562341395977,0.));
#21662=CARTESIAN_POINT('Ctrl Pts',(11.7410945211992,-41.7562341395977,18.));
#21663=CARTESIAN_POINT('Ctrl Pts',(11.81512813804,-41.8282796562569,0.));
#21664=CARTESIAN_POINT('Ctrl Pts',(11.81512813804,-41.8282796562569,18.));
#21665=CARTESIAN_POINT('Ctrl Pts',(11.8895948153349,-41.9000638152266,0.));
#21666=CARTESIAN_POINT('Ctrl Pts',(11.8895948153349,-41.9000638152266,18.));
#21667=CARTESIAN_POINT('Ctrl Pts',(11.9644914999263,-41.9715865222182,0.));
#21668=CARTESIAN_POINT('Ctrl Pts',(11.9644914999263,-41.9715865222182,18.));
#21669=CARTESIAN_POINT('Ctrl Pts',(12.0398158079102,-42.0428479428228,0.));
#21670=CARTESIAN_POINT('Ctrl Pts',(12.0398158079102,-42.0428479428228,18.));
#21671=CARTESIAN_POINT('Ctrl Pts',(12.1155659644537,-42.1138483839101,0.));
#21672=CARTESIAN_POINT('Ctrl Pts',(12.1155659644537,-42.1138483839101,18.));
#21673=CARTESIAN_POINT('Ctrl Pts',(12.1765058047069,-42.1704402333854,0.));
#21674=CARTESIAN_POINT('Ctrl Pts',(12.1765058047069,-42.1704402333854,18.));
#21675=CARTESIAN_POINT('Ctrl Pts',(12.2224014666679,-42.2127669677092,0.));
#21676=CARTESIAN_POINT('Ctrl Pts',(12.2224014666679,-42.2127669677092,18.));
#21677=CARTESIAN_POINT('Ctrl Pts',(12.2530833383985,-42.2409327400055,0.));
#21678=CARTESIAN_POINT('Ctrl Pts',(12.2530833383985,-42.2409327400055,18.));
#21679=CARTESIAN_POINT('Ctrl Pts',(12.2684454652018,-42.2550026135057,0.));
#21680=CARTESIAN_POINT('Ctrl Pts',(12.2684454652018,-42.2550026135057,18.));
#21681=CARTESIAN_POINT('Ctrl Pts',(8.2289783962506,-36.6758703925241,0.));
#21682=CARTESIAN_POINT('Ctrl Pts',(8.23313075335376,-36.6943771018148,0.));
#21683=CARTESIAN_POINT('Ctrl Pts',(8.24192165947366,-36.7312504697652,0.));
#21684=CARTESIAN_POINT('Ctrl Pts',(8.2565665745182,-36.7861403757604,0.));
#21685=CARTESIAN_POINT('Ctrl Pts',(8.27886599440784,-36.8585291300917,0.));
#21686=CARTESIAN_POINT('Ctrl Pts',(8.3105254779459,-36.9479311729484,0.));
#21687=CARTESIAN_POINT('Ctrl Pts',(8.34490818952639,-37.0365602155148,0.));
#21688=CARTESIAN_POINT('Ctrl Pts',(8.38096706211447,-37.1247207489179,0.));
#21689=CARTESIAN_POINT('Ctrl Pts',(8.41793088313259,-37.2126332013933,0.));
#21690=CARTESIAN_POINT('Ctrl Pts',(8.45550849433959,-37.3003733151561,0.));
#21691=CARTESIAN_POINT('Ctrl Pts',(8.49372546467075,-37.3879218093514,0.));
#21692=CARTESIAN_POINT('Ctrl Pts',(8.53279758643783,-37.4752030152968,0.));
#21693=CARTESIAN_POINT('Ctrl Pts',(8.57299698459465,-37.5621256752108,0.));
#21694=CARTESIAN_POINT('Ctrl Pts',(8.61450621749154,-37.6486274754754,0.));
#21695=CARTESIAN_POINT('Ctrl Pts',(8.65732553894524,-37.7347032383719,0.));
#21696=CARTESIAN_POINT('Ctrl Pts',(8.70134776631143,-37.8203816669031,0.));
#21697=CARTESIAN_POINT('Ctrl Pts',(8.74640499479001,-37.9057107230066,0.));
#21698=CARTESIAN_POINT('Ctrl Pts',(8.79232279131091,-37.9907407304174,0.));
#21699=CARTESIAN_POINT('Ctrl Pts',(8.83897959763348,-38.0755058326913,0.));
#21700=CARTESIAN_POINT('Ctrl Pts',(8.88633535238434,-38.1600150482528,0.));
#21701=CARTESIAN_POINT('Ctrl Pts',(8.93439830996338,-38.2442625706309,0.));
#21702=CARTESIAN_POINT('Ctrl Pts',(8.98320483785759,-38.3282340281403,0.));
#21703=CARTESIAN_POINT('Ctrl Pts',(9.0327957936019,-38.4119138099805,0.));
#21704=CARTESIAN_POINT('Ctrl Pts',(9.08319014288085,-38.4952932486131,0.));
#21705=CARTESIAN_POINT('Ctrl Pts',(9.13437512010585,-38.5783736628826,0.));
#21706=CARTESIAN_POINT('Ctrl Pts',(9.18632019394329,-38.6611620045193,0.));
#21707=CARTESIAN_POINT('Ctrl Pts',(9.2389853919933,-38.7436682576832,0.));
#21708=CARTESIAN_POINT('Ctrl Pts',(9.29233110570902,-38.8259023794241,0.));
#21709=CARTESIAN_POINT('Ctrl Pts',(9.34632917154636,-38.9078708427078,0.));
#21710=CARTESIAN_POINT('Ctrl Pts',(9.40096600877643,-38.9895756526779,0.));
#21711=CARTESIAN_POINT('Ctrl Pts',(9.45623664577431,-39.0710161994951,0.));
#21712=CARTESIAN_POINT('Ctrl Pts',(9.5121410453562,-39.1521903958955,0.));
#21713=CARTESIAN_POINT('Ctrl Pts',(9.56867984233622,-39.2330959982788,0.));
#21714=CARTESIAN_POINT('Ctrl Pts',(9.62584947846542,-39.3137321153686,0.));
#21715=CARTESIAN_POINT('Ctrl Pts',(9.68364100883825,-39.3940995760289,0.));
#21716=CARTESIAN_POINT('Ctrl Pts',(9.74204258152662,-39.4742001555227,0.));
#21717=CARTESIAN_POINT('Ctrl Pts',(9.80104095251613,-39.5540361022309,0.));
#21718=CARTESIAN_POINT('Ctrl Pts',(9.86062324242559,-39.6336095893767,0.));
#21719=CARTESIAN_POINT('Ctrl Pts',(9.92077894513191,-39.712922089547,0.));
#21720=CARTESIAN_POINT('Ctrl Pts',(9.98150036150822,-39.7919742367922,0.));
#21721=CARTESIAN_POINT('Ctrl Pts',(10.0427815229883,-39.8707661565233,0.));
#21722=CARTESIAN_POINT('Ctrl Pts',(10.1046175096878,-39.9492976736738,0.));
#21723=CARTESIAN_POINT('Ctrl Pts',(10.1670036683795,-40.0275685525923,0.));
#21724=CARTESIAN_POINT('Ctrl Pts',(10.2299347125857,-40.1055787732578,0.));
#21725=CARTESIAN_POINT('Ctrl Pts',(10.2934044990237,-40.1833286010098,0.));
#21726=CARTESIAN_POINT('Ctrl Pts',(10.3574064830678,-40.2608184485326,0.));
#21727=CARTESIAN_POINT('Ctrl Pts',(10.421933993295,-40.3380487942952,0.));
#21728=CARTESIAN_POINT('Ctrl Pts',(10.48698054978,-40.4150200869536,0.));
#21729=CARTESIAN_POINT('Ctrl Pts',(10.552540223795,-40.4917326404439,0.));
#21730=CARTESIAN_POINT('Ctrl Pts',(10.618607730849,-40.5681866012103,0.));
#21731=CARTESIAN_POINT('Ctrl Pts',(10.6851782157325,-40.6443819999244,0.));
#21732=CARTESIAN_POINT('Ctrl Pts',(10.7522471109694,-40.7203187831783,0.));
#21733=CARTESIAN_POINT('Ctrl Pts',(10.8198099757795,-40.7959968527561,0.));
#21734=CARTESIAN_POINT('Ctrl Pts',(10.8878623066646,-40.8714161092412,0.));
#21735=CARTESIAN_POINT('Ctrl Pts',(10.956399476781,-40.9465764747798,0.));
#21736=CARTESIAN_POINT('Ctrl Pts',(11.0254168609972,-41.0214778832142,0.));
#21737=CARTESIAN_POINT('Ctrl Pts',(11.0949099155251,-41.0961202807715,0.));
#21738=CARTESIAN_POINT('Ctrl Pts',(11.1648742640378,-41.1705036228854,0.));
#21739=CARTESIAN_POINT('Ctrl Pts',(11.2353057980338,-41.2446278781981,0.));
#21740=CARTESIAN_POINT('Ctrl Pts',(11.3062006993745,-41.3184930194148,0.));
#21741=CARTESIAN_POINT('Ctrl Pts',(11.3775553120176,-41.3920989905986,0.));
#21742=CARTESIAN_POINT('Ctrl Pts',(11.4493660393849,-41.4654456796071,0.));
#21743=CARTESIAN_POINT('Ctrl Pts',(11.5216292382388,-41.5385328935506,0.));
#21744=CARTESIAN_POINT('Ctrl Pts',(11.5943410868252,-41.6113603270596,0.));
#21745=CARTESIAN_POINT('Ctrl Pts',(11.6674975352851,-41.6839275596248,0.));
#21746=CARTESIAN_POINT('Ctrl Pts',(11.7410945211992,-41.7562341395977,0.));
#21747=CARTESIAN_POINT('Ctrl Pts',(11.81512813804,-41.8282796562569,0.));
#21748=CARTESIAN_POINT('Ctrl Pts',(11.8895948153349,-41.9000638152266,0.));
#21749=CARTESIAN_POINT('Ctrl Pts',(11.9644914999263,-41.9715865222182,0.));
#21750=CARTESIAN_POINT('Ctrl Pts',(12.054880669507,-42.0571002269437,0.));
#21751=CARTESIAN_POINT('Ctrl Pts',(12.1307372881904,-42.1280354231517,0.));
#21752=CARTESIAN_POINT('Ctrl Pts',(12.1917619768791,-42.18457517013,0.));
#21753=CARTESIAN_POINT('Ctrl Pts',(12.2377212115623,-42.2268628664988,0.));
#21754=CARTESIAN_POINT('Ctrl Pts',(12.2684454652018,-42.2550026135057,0.));
#21755=CARTESIAN_POINT('Ctrl Pts',(8.2289783962506,-36.6758703925241,15.));
#21756=CARTESIAN_POINT('Ctrl Pts',(8.23313075335376,-36.6943771018148,15.));
#21757=CARTESIAN_POINT('Ctrl Pts',(8.24192165947366,-36.7312504697652,15.));
#21758=CARTESIAN_POINT('Ctrl Pts',(8.2565665745182,-36.7861403757604,15.));
#21759=CARTESIAN_POINT('Ctrl Pts',(8.27886599440784,-36.8585291300917,15.));
#21760=CARTESIAN_POINT('Ctrl Pts',(8.3105254779459,-36.9479311729484,15.));
#21761=CARTESIAN_POINT('Ctrl Pts',(8.34490818952639,-37.0365602155148,15.));
#21762=CARTESIAN_POINT('Ctrl Pts',(8.38096706211447,-37.1247207489179,15.));
#21763=CARTESIAN_POINT('Ctrl Pts',(8.41793088313259,-37.2126332013933,15.));
#21764=CARTESIAN_POINT('Ctrl Pts',(8.45550849433959,-37.3003733151561,15.));
#21765=CARTESIAN_POINT('Ctrl Pts',(8.49372546467075,-37.3879218093514,15.));
#21766=CARTESIAN_POINT('Ctrl Pts',(8.53279758643783,-37.4752030152968,15.));
#21767=CARTESIAN_POINT('Ctrl Pts',(8.57299698459465,-37.5621256752108,15.));
#21768=CARTESIAN_POINT('Ctrl Pts',(8.61450621749154,-37.6486274754754,15.));
#21769=CARTESIAN_POINT('Ctrl Pts',(8.65732553894524,-37.7347032383719,15.));
#21770=CARTESIAN_POINT('Ctrl Pts',(8.70134776631143,-37.8203816669031,15.));
#21771=CARTESIAN_POINT('Ctrl Pts',(8.74640499479001,-37.9057107230066,15.));
#21772=CARTESIAN_POINT('Ctrl Pts',(8.79232279131091,-37.9907407304174,15.));
#21773=CARTESIAN_POINT('Ctrl Pts',(8.83897959763348,-38.0755058326913,15.));
#21774=CARTESIAN_POINT('Ctrl Pts',(8.88633535238434,-38.1600150482528,15.));
#21775=CARTESIAN_POINT('Ctrl Pts',(8.93439830996338,-38.2442625706309,15.));
#21776=CARTESIAN_POINT('Ctrl Pts',(8.98320483785759,-38.3282340281403,15.));
#21777=CARTESIAN_POINT('Ctrl Pts',(9.0327957936019,-38.4119138099805,15.));
#21778=CARTESIAN_POINT('Ctrl Pts',(9.08319014288085,-38.4952932486131,15.));
#21779=CARTESIAN_POINT('Ctrl Pts',(9.13437512010585,-38.5783736628826,15.));
#21780=CARTESIAN_POINT('Ctrl Pts',(9.18632019394329,-38.6611620045193,15.));
#21781=CARTESIAN_POINT('Ctrl Pts',(9.2389853919933,-38.7436682576832,15.));
#21782=CARTESIAN_POINT('Ctrl Pts',(9.29233110570902,-38.8259023794241,15.));
#21783=CARTESIAN_POINT('Ctrl Pts',(9.34632917154636,-38.9078708427078,15.));
#21784=CARTESIAN_POINT('Ctrl Pts',(9.40096600877643,-38.9895756526779,15.));
#21785=CARTESIAN_POINT('Ctrl Pts',(9.45623664577431,-39.0710161994951,15.));
#21786=CARTESIAN_POINT('Ctrl Pts',(9.5121410453562,-39.1521903958955,15.));
#21787=CARTESIAN_POINT('Ctrl Pts',(9.56867984233622,-39.2330959982788,15.));
#21788=CARTESIAN_POINT('Ctrl Pts',(9.62584947846542,-39.3137321153686,15.));
#21789=CARTESIAN_POINT('Ctrl Pts',(9.68364100883825,-39.3940995760289,15.));
#21790=CARTESIAN_POINT('Ctrl Pts',(9.74204258152662,-39.4742001555227,15.));
#21791=CARTESIAN_POINT('Ctrl Pts',(9.80104095251613,-39.5540361022309,15.));
#21792=CARTESIAN_POINT('Ctrl Pts',(9.86062324242559,-39.6336095893767,15.));
#21793=CARTESIAN_POINT('Ctrl Pts',(9.92077894513191,-39.712922089547,15.));
#21794=CARTESIAN_POINT('Ctrl Pts',(9.98150036150822,-39.7919742367922,15.));
#21795=CARTESIAN_POINT('Ctrl Pts',(10.0427815229883,-39.8707661565233,15.));
#21796=CARTESIAN_POINT('Ctrl Pts',(10.1046175096878,-39.9492976736738,15.));
#21797=CARTESIAN_POINT('Ctrl Pts',(10.1670036683795,-40.0275685525923,15.));
#21798=CARTESIAN_POINT('Ctrl Pts',(10.2299347125857,-40.1055787732578,15.));
#21799=CARTESIAN_POINT('Ctrl Pts',(10.2934044990237,-40.1833286010098,15.));
#21800=CARTESIAN_POINT('Ctrl Pts',(10.3574064830678,-40.2608184485326,15.));
#21801=CARTESIAN_POINT('Ctrl Pts',(10.421933993295,-40.3380487942952,15.));
#21802=CARTESIAN_POINT('Ctrl Pts',(10.48698054978,-40.4150200869536,15.));
#21803=CARTESIAN_POINT('Ctrl Pts',(10.552540223795,-40.4917326404439,15.));
#21804=CARTESIAN_POINT('Ctrl Pts',(10.618607730849,-40.5681866012103,15.));
#21805=CARTESIAN_POINT('Ctrl Pts',(10.6851782157325,-40.6443819999244,15.));
#21806=CARTESIAN_POINT('Ctrl Pts',(10.7522471109694,-40.7203187831783,15.));
#21807=CARTESIAN_POINT('Ctrl Pts',(10.8198099757795,-40.7959968527561,15.));
#21808=CARTESIAN_POINT('Ctrl Pts',(10.8878623066646,-40.8714161092412,15.));
#21809=CARTESIAN_POINT('Ctrl Pts',(10.956399476781,-40.9465764747798,15.));
#21810=CARTESIAN_POINT('Ctrl Pts',(11.0254168609972,-41.0214778832142,15.));
#21811=CARTESIAN_POINT('Ctrl Pts',(11.0949099155251,-41.0961202807715,15.));
#21812=CARTESIAN_POINT('Ctrl Pts',(11.1648742640378,-41.1705036228854,15.));
#21813=CARTESIAN_POINT('Ctrl Pts',(11.2353057980338,-41.2446278781981,15.));
#21814=CARTESIAN_POINT('Ctrl Pts',(11.3062006993745,-41.3184930194148,15.));
#21815=CARTESIAN_POINT('Ctrl Pts',(11.3775553120176,-41.3920989905986,15.));
#21816=CARTESIAN_POINT('Ctrl Pts',(11.4493660393849,-41.4654456796071,15.));
#21817=CARTESIAN_POINT('Ctrl Pts',(11.5216292382388,-41.5385328935506,15.));
#21818=CARTESIAN_POINT('Ctrl Pts',(11.5943410868252,-41.6113603270596,15.));
#21819=CARTESIAN_POINT('Ctrl Pts',(11.6674975352851,-41.6839275596248,15.));
#21820=CARTESIAN_POINT('Ctrl Pts',(11.7410945211992,-41.7562341395977,15.));
#21821=CARTESIAN_POINT('Ctrl Pts',(11.81512813804,-41.8282796562569,15.));
#21822=CARTESIAN_POINT('Ctrl Pts',(11.8895948153349,-41.9000638152266,15.));
#21823=CARTESIAN_POINT('Ctrl Pts',(11.9644914999263,-41.9715865222182,15.));
#21824=CARTESIAN_POINT('Ctrl Pts',(12.054880669507,-42.0571002269437,15.));
#21825=CARTESIAN_POINT('Ctrl Pts',(12.1307372881904,-42.1280354231517,15.));
#21826=CARTESIAN_POINT('Ctrl Pts',(12.1917619768791,-42.18457517013,15.));
#21827=CARTESIAN_POINT('Ctrl Pts',(12.2377212115623,-42.2268628664988,15.));
#21828=CARTESIAN_POINT('Ctrl Pts',(12.2684454652018,-42.2550026135057,15.));
#21829=CARTESIAN_POINT('Ctrl Pts',(1.38952890043915,-43.9780537249529,0.));
#21830=CARTESIAN_POINT('Ctrl Pts',(1.38952890043915,-43.9780537249529,18.));
#21831=CARTESIAN_POINT('Ctrl Pts',(1.3997913212193,-43.9599253218252,0.));
#21832=CARTESIAN_POINT('Ctrl Pts',(1.3997913212193,-43.9599253218252,18.));
#21833=CARTESIAN_POINT('Ctrl Pts',(1.42026781296156,-43.9236568607623,0.));
#21834=CARTESIAN_POINT('Ctrl Pts',(1.42026781296156,-43.9236568607623,18.));
#21835=CARTESIAN_POINT('Ctrl Pts',(1.45083750111681,-43.8692192047561,0.));
#21836=CARTESIAN_POINT('Ctrl Pts',(1.45083750111681,-43.8692192047561,18.));
#21837=CARTESIAN_POINT('Ctrl Pts',(1.49130689006066,-43.7965657112708,0.));
#21838=CARTESIAN_POINT('Ctrl Pts',(1.49130689006066,-43.7965657112708,18.));
#21839=CARTESIAN_POINT('Ctrl Pts',(1.54140922714764,-43.7056321934163,0.));
#21840=CARTESIAN_POINT('Ctrl Pts',(1.54140922714764,-43.7056321934163,18.));
#21841=CARTESIAN_POINT('Ctrl Pts',(1.59102591108103,-43.6145820637333,0.));
#21842=CARTESIAN_POINT('Ctrl Pts',(1.59102591108103,-43.6145820637333,18.));
#21843=CARTESIAN_POINT('Ctrl Pts',(1.64015515906647,-43.5234155788248,0.));
#21844=CARTESIAN_POINT('Ctrl Pts',(1.64015515906647,-43.5234155788248,18.));
#21845=CARTESIAN_POINT('Ctrl Pts',(1.68879465270607,-43.4321333178711,0.));
#21846=CARTESIAN_POINT('Ctrl Pts',(1.68879465270607,-43.4321333178711,18.));
#21847=CARTESIAN_POINT('Ctrl Pts',(1.73694151741123,-43.3407363140236,0.));
#21848=CARTESIAN_POINT('Ctrl Pts',(1.73694151741123,-43.3407363140236,18.));
#21849=CARTESIAN_POINT('Ctrl Pts',(1.78459244842769,-43.2492259505872,0.));
#21850=CARTESIAN_POINT('Ctrl Pts',(1.78459244842769,-43.2492259505872,18.));
#21851=CARTESIAN_POINT('Ctrl Pts',(1.83174385734711,-43.1576038253643,0.));
#21852=CARTESIAN_POINT('Ctrl Pts',(1.83174385734711,-43.1576038253643,18.));
#21853=CARTESIAN_POINT('Ctrl Pts',(1.87839202014608,-43.065871623255,0.));
#21854=CARTESIAN_POINT('Ctrl Pts',(1.87839202014608,-43.065871623255,18.));
#21855=CARTESIAN_POINT('Ctrl Pts',(1.92453321512435,-42.9740309956624,0.));
#21856=CARTESIAN_POINT('Ctrl Pts',(1.92453321512435,-42.9740309956624,18.));
#21857=CARTESIAN_POINT('Ctrl Pts',(1.97016390194215,-42.8820834139973,0.));
#21858=CARTESIAN_POINT('Ctrl Pts',(1.97016390194215,-42.8820834139973,18.));
#21859=CARTESIAN_POINT('Ctrl Pts',(2.01528067528089,-42.7900301875309,0.));
#21860=CARTESIAN_POINT('Ctrl Pts',(2.01528067528089,-42.7900301875309,18.));
#21861=CARTESIAN_POINT('Ctrl Pts',(2.05988014924518,-42.6978725343209,0.));
#21862=CARTESIAN_POINT('Ctrl Pts',(2.05988014924518,-42.6978725343209,18.));
#21863=CARTESIAN_POINT('Ctrl Pts',(2.1039588640177,-42.6056116373455,0.));
#21864=CARTESIAN_POINT('Ctrl Pts',(2.1039588640177,-42.6056116373455,18.));
#21865=CARTESIAN_POINT('Ctrl Pts',(2.14751319676745,-42.5132487024335,0.));
#21866=CARTESIAN_POINT('Ctrl Pts',(2.14751319676745,-42.5132487024335,18.));
#21867=CARTESIAN_POINT('Ctrl Pts',(2.19053924976737,-42.4207850290047,0.));
#21868=CARTESIAN_POINT('Ctrl Pts',(2.19053924976737,-42.4207850290047,18.));
#21869=CARTESIAN_POINT('Ctrl Pts',(2.23303287465499,-42.3282220118033,0.));
#21870=CARTESIAN_POINT('Ctrl Pts',(2.23303287465499,-42.3282220118033,18.));
#21871=CARTESIAN_POINT('Ctrl Pts',(2.27498976664773,-42.2355611060784,0.));
#21872=CARTESIAN_POINT('Ctrl Pts',(2.27498976664773,-42.2355611060784,18.));
#21873=CARTESIAN_POINT('Ctrl Pts',(2.31640554742808,-42.1428038039937,0.));
#21874=CARTESIAN_POINT('Ctrl Pts',(2.31640554742808,-42.1428038039937,18.));
#21875=CARTESIAN_POINT('Ctrl Pts',(2.35727584066428,-42.0499516093661,0.));
#21876=CARTESIAN_POINT('Ctrl Pts',(2.35727584066428,-42.0499516093661,18.));
#21877=CARTESIAN_POINT('Ctrl Pts',(2.39759639399648,-41.9570060084039,0.));
#21878=CARTESIAN_POINT('Ctrl Pts',(2.39759639399648,-41.9570060084039,18.));
#21879=CARTESIAN_POINT('Ctrl Pts',(2.437363014342,-41.8639684667923,0.));
#21880=CARTESIAN_POINT('Ctrl Pts',(2.437363014342,-41.8639684667923,18.));
#21881=CARTESIAN_POINT('Ctrl Pts',(2.47657137427692,-41.7708404467533,0.));
#21882=CARTESIAN_POINT('Ctrl Pts',(2.47657137427692,-41.7708404467533,18.));
#21883=CARTESIAN_POINT('Ctrl Pts',(2.51521684674476,-41.6776234194583,0.));
#21884=CARTESIAN_POINT('Ctrl Pts',(2.51521684674476,-41.6776234194583,18.));
#21885=CARTESIAN_POINT('Ctrl Pts',(2.55329436064183,-41.5843188786284,0.));
#21886=CARTESIAN_POINT('Ctrl Pts',(2.55329436064183,-41.5843188786284,18.));
#21887=CARTESIAN_POINT('Ctrl Pts',(2.59079818040171,-41.4909283577703,0.));
#21888=CARTESIAN_POINT('Ctrl Pts',(2.59079818040171,-41.4909283577703,18.));
#21889=CARTESIAN_POINT('Ctrl Pts',(2.62772200460655,-41.3974534325936,0.));
#21890=CARTESIAN_POINT('Ctrl Pts',(2.62772200460655,-41.3974534325936,18.));
#21891=CARTESIAN_POINT('Ctrl Pts',(2.66405934050117,-41.3038957096306,0.));
#21892=CARTESIAN_POINT('Ctrl Pts',(2.66405934050117,-41.3038957096306,18.));
#21893=CARTESIAN_POINT('Ctrl Pts',(2.69980383625015,-41.2102568187956,0.));
#21894=CARTESIAN_POINT('Ctrl Pts',(2.69980383625015,-41.2102568187956,18.));
#21895=CARTESIAN_POINT('Ctrl Pts',(2.73494956725005,-41.1165384061145,0.));
#21896=CARTESIAN_POINT('Ctrl Pts',(2.73494956725005,-41.1165384061145,18.));
#21897=CARTESIAN_POINT('Ctrl Pts',(2.76949151194863,-41.0227421242398,0.));
#21898=CARTESIAN_POINT('Ctrl Pts',(2.76949151194863,-41.0227421242398,18.));
#21899=CARTESIAN_POINT('Ctrl Pts',(2.80342531768404,-40.9288696352159,0.));
#21900=CARTESIAN_POINT('Ctrl Pts',(2.80342531768404,-40.9288696352159,18.));
#21901=CARTESIAN_POINT('Ctrl Pts',(2.83674635946678,-40.8349226258683,0.));
#21902=CARTESIAN_POINT('Ctrl Pts',(2.83674635946678,-40.8349226258683,18.));
#21903=CARTESIAN_POINT('Ctrl Pts',(2.86944892209897,-40.7409028213129,0.));
#21904=CARTESIAN_POINT('Ctrl Pts',(2.86944892209897,-40.7409028213129,18.));
#21905=CARTESIAN_POINT('Ctrl Pts',(2.90152548734342,-40.6468119976928,0.));
#21906=CARTESIAN_POINT('Ctrl Pts',(2.90152548734342,-40.6468119976928,18.));
#21907=CARTESIAN_POINT('Ctrl Pts',(2.93296560822893,-40.5526520010651,0.));
#21908=CARTESIAN_POINT('Ctrl Pts',(2.93296560822893,-40.5526520010651,18.));
#21909=CARTESIAN_POINT('Ctrl Pts',(2.96375636417322,-40.4584247445196,0.));
#21910=CARTESIAN_POINT('Ctrl Pts',(2.96375636417322,-40.4584247445196,18.));
#21911=CARTESIAN_POINT('Ctrl Pts',(2.99388446458219,-40.3641321823444,0.));
#21912=CARTESIAN_POINT('Ctrl Pts',(2.99388446458219,-40.3641321823444,18.));
#21913=CARTESIAN_POINT('Ctrl Pts',(3.02333808901594,-40.2697762886113,0.));
#21914=CARTESIAN_POINT('Ctrl Pts',(3.02333808901594,-40.2697762886113,18.));
#21915=CARTESIAN_POINT('Ctrl Pts',(3.0521084742307,-40.1753590391515,0.));
#21916=CARTESIAN_POINT('Ctrl Pts',(3.0521084742307,-40.1753590391515,18.));
#21917=CARTESIAN_POINT('Ctrl Pts',(3.08019251155015,-40.0808823811787,0.));
#21918=CARTESIAN_POINT('Ctrl Pts',(3.08019251155015,-40.0808823811787,18.));
#21919=CARTESIAN_POINT('Ctrl Pts',(3.10759149802907,-39.9863482523153,0.));
#21920=CARTESIAN_POINT('Ctrl Pts',(3.10759149802907,-39.9863482523153,18.));
#21921=CARTESIAN_POINT('Ctrl Pts',(3.13430604330355,-39.8917586491576,0.));
#21922=CARTESIAN_POINT('Ctrl Pts',(3.13430604330355,-39.8917586491576,18.));
#21923=CARTESIAN_POINT('Ctrl Pts',(3.16033160752803,-39.7971156880138,0.));
#21924=CARTESIAN_POINT('Ctrl Pts',(3.16033160752803,-39.7971156880138,18.));
#21925=CARTESIAN_POINT('Ctrl Pts',(3.18565465503835,-39.7024216585552,0.));
#21926=CARTESIAN_POINT('Ctrl Pts',(3.18565465503835,-39.7024216585552,18.));
#21927=CARTESIAN_POINT('Ctrl Pts',(3.21024640045595,-39.607679107639,0.));
#21928=CARTESIAN_POINT('Ctrl Pts',(3.21024640045595,-39.607679107639,18.));
#21929=CARTESIAN_POINT('Ctrl Pts',(3.2340660969166,-39.5128908052622,0.));
#21930=CARTESIAN_POINT('Ctrl Pts',(3.2340660969166,-39.5128908052622,18.));
#21931=CARTESIAN_POINT('Ctrl Pts',(3.25707264313387,-39.4180596080755,0.));
#21932=CARTESIAN_POINT('Ctrl Pts',(3.25707264313387,-39.4180596080755,18.));
#21933=CARTESIAN_POINT('Ctrl Pts',(3.27923485388116,-39.3231883392913,0.));
#21934=CARTESIAN_POINT('Ctrl Pts',(3.27923485388116,-39.3231883392913,18.));
#21935=CARTESIAN_POINT('Ctrl Pts',(3.30054018081687,-39.2282796893977,0.));
#21936=CARTESIAN_POINT('Ctrl Pts',(3.30054018081687,-39.2282796893977,18.));
#21937=CARTESIAN_POINT('Ctrl Pts',(3.32100933979557,-39.1333360409949,0.));
#21938=CARTESIAN_POINT('Ctrl Pts',(3.32100933979557,-39.1333360409949,18.));
#21939=CARTESIAN_POINT('Ctrl Pts',(3.34068601264472,-39.0383596151636,0.));
#21940=CARTESIAN_POINT('Ctrl Pts',(3.34068601264472,-39.0383596151636,18.));
#21941=CARTESIAN_POINT('Ctrl Pts',(3.3596092279948,-38.9433528420174,0.));
#21942=CARTESIAN_POINT('Ctrl Pts',(3.3596092279948,-38.9433528420174,18.));
#21943=CARTESIAN_POINT('Ctrl Pts',(3.37778863054481,-38.8483186930884,0.));
#21944=CARTESIAN_POINT('Ctrl Pts',(3.37778863054481,-38.8483186930884,18.));
#21945=CARTESIAN_POINT('Ctrl Pts',(3.39518333281817,-38.7532609709905,0.));
#21946=CARTESIAN_POINT('Ctrl Pts',(3.39518333281817,-38.7532609709905,18.));
#21947=CARTESIAN_POINT('Ctrl Pts',(3.411667175119,-38.6581847668347,0.));
#21948=CARTESIAN_POINT('Ctrl Pts',(3.411667175119,-38.6581847668347,18.));
#21949=CARTESIAN_POINT('Ctrl Pts',(3.42705871084996,-38.5630961226878,0.));
#21950=CARTESIAN_POINT('Ctrl Pts',(3.42705871084996,-38.5630961226878,18.));
#21951=CARTESIAN_POINT('Ctrl Pts',(3.44118343200302,-38.4680013094732,0.));
#21952=CARTESIAN_POINT('Ctrl Pts',(3.44118343200302,-38.4680013094732,18.));
#21953=CARTESIAN_POINT('Ctrl Pts',(3.45393053211022,-38.3729061502716,0.));
#21954=CARTESIAN_POINT('Ctrl Pts',(3.45393053211022,-38.3729061502716,18.));
#21955=CARTESIAN_POINT('Ctrl Pts',(3.46530185256872,-38.2778154909527,0.));
#21956=CARTESIAN_POINT('Ctrl Pts',(3.46530185256872,-38.2778154909527,18.));
#21957=CARTESIAN_POINT('Ctrl Pts',(3.47549027265411,-38.1827321816559,0.));
#21958=CARTESIAN_POINT('Ctrl Pts',(3.47549027265411,-38.1827321816559,18.));
#21959=CARTESIAN_POINT('Ctrl Pts',(3.48478279878233,-38.0876589224537,0.));
#21960=CARTESIAN_POINT('Ctrl Pts',(3.48478279878233,-38.0876589224537,18.));
#21961=CARTESIAN_POINT('Ctrl Pts',(3.49340804454645,-37.9926009950482,0.));
#21962=CARTESIAN_POINT('Ctrl Pts',(3.49340804454645,-37.9926009950482,18.));
#21963=CARTESIAN_POINT('Ctrl Pts',(3.50139628556083,-37.8975688353863,0.));
#21964=CARTESIAN_POINT('Ctrl Pts',(3.50139628556083,-37.8975688353863,18.));
#21965=CARTESIAN_POINT('Ctrl Pts',(3.50844720825127,-37.8025803811856,0.));
#21966=CARTESIAN_POINT('Ctrl Pts',(3.50844720825127,-37.8025803811856,18.));
#21967=CARTESIAN_POINT('Ctrl Pts',(3.51375922979957,-37.7076643105286,0.));
#21968=CARTESIAN_POINT('Ctrl Pts',(3.51375922979957,-37.7076643105286,18.));
#21969=CARTESIAN_POINT('Ctrl Pts',(3.51624243734644,-37.6128545966533,0.));
#21970=CARTESIAN_POINT('Ctrl Pts',(3.51624243734644,-37.6128545966533,18.));
#21971=CARTESIAN_POINT('Ctrl Pts',(3.51508109065209,-37.5371179004295,0.));
#21972=CARTESIAN_POINT('Ctrl Pts',(3.51508109065209,-37.5371179004295,18.));
#21973=CARTESIAN_POINT('Ctrl Pts',(3.5120473187636,-37.4803889700239,0.));
#21974=CARTESIAN_POINT('Ctrl Pts',(3.5120473187636,-37.4803889700239,18.));
#21975=CARTESIAN_POINT('Ctrl Pts',(3.50901346997656,-37.4426037737699,0.));
#21976=CARTESIAN_POINT('Ctrl Pts',(3.50901346997656,-37.4426037737699,18.));
#21977=CARTESIAN_POINT('Ctrl Pts',(3.50724370857672,-37.4237196983922,0.));
#21978=CARTESIAN_POINT('Ctrl Pts',(3.50724370857672,-37.4237196983922,18.));
#21979=CARTESIAN_POINT('',(1.38952890043928,-43.9780537249529,0.));
#21980=CARTESIAN_POINT('Ctrl Pts',(3.50724370857672,-37.4237196983922,0.));
#21981=CARTESIAN_POINT('Ctrl Pts',(3.50901346997656,-37.4426037737699,0.));
#21982=CARTESIAN_POINT('Ctrl Pts',(3.5120473187636,-37.4803889700239,0.));
#21983=CARTESIAN_POINT('Ctrl Pts',(3.51508109065209,-37.5371179004295,0.));
#21984=CARTESIAN_POINT('Ctrl Pts',(3.51624243734644,-37.6128545966533,0.));
#21985=CARTESIAN_POINT('Ctrl Pts',(3.51375922979957,-37.7076643105286,0.));
#21986=CARTESIAN_POINT('Ctrl Pts',(3.50844720825127,-37.8025803811856,0.));
#21987=CARTESIAN_POINT('Ctrl Pts',(3.50139628556083,-37.8975688353863,0.));
#21988=CARTESIAN_POINT('Ctrl Pts',(3.49340804454645,-37.9926009950482,0.));
#21989=CARTESIAN_POINT('Ctrl Pts',(3.48478279878233,-38.0876589224537,0.));
#21990=CARTESIAN_POINT('Ctrl Pts',(3.47549027265411,-38.1827321816559,0.));
#21991=CARTESIAN_POINT('Ctrl Pts',(3.46530185256872,-38.2778154909527,0.));
#21992=CARTESIAN_POINT('Ctrl Pts',(3.45393053211022,-38.3729061502716,0.));
#21993=CARTESIAN_POINT('Ctrl Pts',(3.44118343200302,-38.4680013094732,0.));
#21994=CARTESIAN_POINT('Ctrl Pts',(3.42705871084996,-38.5630961226878,0.));
#21995=CARTESIAN_POINT('Ctrl Pts',(3.411667175119,-38.6581847668347,0.));
#21996=CARTESIAN_POINT('Ctrl Pts',(3.39518333281817,-38.7532609709905,0.));
#21997=CARTESIAN_POINT('Ctrl Pts',(3.37778863054481,-38.8483186930884,0.));
#21998=CARTESIAN_POINT('Ctrl Pts',(3.3596092279948,-38.9433528420174,0.));
#21999=CARTESIAN_POINT('Ctrl Pts',(3.34068601264472,-39.0383596151636,0.));
#22000=CARTESIAN_POINT('Ctrl Pts',(3.32100933979557,-39.1333360409949,0.));
#22001=CARTESIAN_POINT('Ctrl Pts',(3.30054018081687,-39.2282796893977,0.));
#22002=CARTESIAN_POINT('Ctrl Pts',(3.27923485388116,-39.3231883392913,0.));
#22003=CARTESIAN_POINT('Ctrl Pts',(3.25707264313387,-39.4180596080755,0.));
#22004=CARTESIAN_POINT('Ctrl Pts',(3.2340660969166,-39.5128908052622,0.));
#22005=CARTESIAN_POINT('Ctrl Pts',(3.21024640045595,-39.607679107639,0.));
#22006=CARTESIAN_POINT('Ctrl Pts',(3.18565465503835,-39.7024216585552,0.));
#22007=CARTESIAN_POINT('Ctrl Pts',(3.16033160752803,-39.7971156880138,0.));
#22008=CARTESIAN_POINT('Ctrl Pts',(3.13430604330355,-39.8917586491576,0.));
#22009=CARTESIAN_POINT('Ctrl Pts',(3.10759149802907,-39.9863482523153,0.));
#22010=CARTESIAN_POINT('Ctrl Pts',(3.08019251155015,-40.0808823811787,0.));
#22011=CARTESIAN_POINT('Ctrl Pts',(3.0521084742307,-40.1753590391515,0.));
#22012=CARTESIAN_POINT('Ctrl Pts',(3.02333808901594,-40.2697762886113,0.));
#22013=CARTESIAN_POINT('Ctrl Pts',(2.99388446458219,-40.3641321823444,0.));
#22014=CARTESIAN_POINT('Ctrl Pts',(2.96375636417322,-40.4584247445196,0.));
#22015=CARTESIAN_POINT('Ctrl Pts',(2.93296560822893,-40.5526520010651,0.));
#22016=CARTESIAN_POINT('Ctrl Pts',(2.90152548734342,-40.6468119976928,0.));
#22017=CARTESIAN_POINT('Ctrl Pts',(2.86944892209897,-40.7409028213129,0.));
#22018=CARTESIAN_POINT('Ctrl Pts',(2.83674635946678,-40.8349226258683,0.));
#22019=CARTESIAN_POINT('Ctrl Pts',(2.80342531768404,-40.9288696352159,0.));
#22020=CARTESIAN_POINT('Ctrl Pts',(2.76949151194863,-41.0227421242398,0.));
#22021=CARTESIAN_POINT('Ctrl Pts',(2.73494956725005,-41.1165384061145,0.));
#22022=CARTESIAN_POINT('Ctrl Pts',(2.69980383625015,-41.2102568187956,0.));
#22023=CARTESIAN_POINT('Ctrl Pts',(2.66405934050117,-41.3038957096306,0.));
#22024=CARTESIAN_POINT('Ctrl Pts',(2.62772200460655,-41.3974534325936,0.));
#22025=CARTESIAN_POINT('Ctrl Pts',(2.59079818040171,-41.4909283577703,0.));
#22026=CARTESIAN_POINT('Ctrl Pts',(2.55329436064183,-41.5843188786284,0.));
#22027=CARTESIAN_POINT('Ctrl Pts',(2.51521684674476,-41.6776234194583,0.));
#22028=CARTESIAN_POINT('Ctrl Pts',(2.47657137427692,-41.7708404467533,0.));
#22029=CARTESIAN_POINT('Ctrl Pts',(2.437363014342,-41.8639684667923,0.));
#22030=CARTESIAN_POINT('Ctrl Pts',(2.39759639399648,-41.9570060084039,0.));
#22031=CARTESIAN_POINT('Ctrl Pts',(2.35727584066428,-42.0499516093661,0.));
#22032=CARTESIAN_POINT('Ctrl Pts',(2.31640554742808,-42.1428038039937,0.));
#22033=CARTESIAN_POINT('Ctrl Pts',(2.27498976664773,-42.2355611060784,0.));
#22034=CARTESIAN_POINT('Ctrl Pts',(2.23303287465499,-42.3282220118033,0.));
#22035=CARTESIAN_POINT('Ctrl Pts',(2.19053924976737,-42.4207850290047,0.));
#22036=CARTESIAN_POINT('Ctrl Pts',(2.14751319676745,-42.5132487024335,0.));
#22037=CARTESIAN_POINT('Ctrl Pts',(2.1039588640177,-42.6056116373455,0.));
#22038=CARTESIAN_POINT('Ctrl Pts',(2.05988014924518,-42.6978725343209,0.));
#22039=CARTESIAN_POINT('Ctrl Pts',(2.01528067528089,-42.7900301875309,0.));
#22040=CARTESIAN_POINT('Ctrl Pts',(1.97016390194215,-42.8820834139973,0.));
#22041=CARTESIAN_POINT('Ctrl Pts',(1.92453321512435,-42.9740309956624,0.));
#22042=CARTESIAN_POINT('Ctrl Pts',(1.87839202014608,-43.065871623255,0.));
#22043=CARTESIAN_POINT('Ctrl Pts',(1.83174385734711,-43.1576038253643,0.));
#22044=CARTESIAN_POINT('Ctrl Pts',(1.78459244842769,-43.2492259505872,0.));
#22045=CARTESIAN_POINT('Ctrl Pts',(1.73694151741123,-43.3407363140236,0.));
#22046=CARTESIAN_POINT('Ctrl Pts',(1.68879465270607,-43.4321333178711,0.));
#22047=CARTESIAN_POINT('Ctrl Pts',(1.64015515906647,-43.5234155788248,0.));
#22048=CARTESIAN_POINT('Ctrl Pts',(1.59102591108103,-43.6145820637333,0.));
#22049=CARTESIAN_POINT('Ctrl Pts',(1.53148589036096,-43.7238422193529,0.));
#22050=CARTESIAN_POINT('Ctrl Pts',(1.48126213998558,-43.8147465842503,0.));
#22051=CARTESIAN_POINT('Ctrl Pts',(1.44069595482722,-43.8873767449247,0.));
#22052=CARTESIAN_POINT('Ctrl Pts',(1.41005374202873,-43.9417969186811,0.));
#22053=CARTESIAN_POINT('Ctrl Pts',(1.38952890043915,-43.9780537249529,0.));
#22054=CARTESIAN_POINT('',(1.38952890043928,-43.9780537249529,15.));
#22055=CARTESIAN_POINT('Ctrl Pts',(1.38952890043915,-43.9780537249529,15.));
#22056=CARTESIAN_POINT('Ctrl Pts',(1.3997913212193,-43.9599253218252,15.));
#22057=CARTESIAN_POINT('Ctrl Pts',(1.42026781296156,-43.9236568607623,15.));
#22058=CARTESIAN_POINT('Ctrl Pts',(1.45083750111681,-43.8692192047561,15.));
#22059=CARTESIAN_POINT('Ctrl Pts',(1.49130689006066,-43.7965657112708,15.));
#22060=CARTESIAN_POINT('Ctrl Pts',(1.54140922714764,-43.7056321934163,15.));
#22061=CARTESIAN_POINT('Ctrl Pts',(1.59102591108103,-43.6145820637333,15.));
#22062=CARTESIAN_POINT('Ctrl Pts',(1.64015515906647,-43.5234155788248,15.));
#22063=CARTESIAN_POINT('Ctrl Pts',(1.68879465270607,-43.4321333178711,15.));
#22064=CARTESIAN_POINT('Ctrl Pts',(1.73694151741123,-43.3407363140236,15.));
#22065=CARTESIAN_POINT('Ctrl Pts',(1.78459244842769,-43.2492259505872,15.));
#22066=CARTESIAN_POINT('Ctrl Pts',(1.83174385734711,-43.1576038253643,15.));
#22067=CARTESIAN_POINT('Ctrl Pts',(1.87839202014608,-43.065871623255,15.));
#22068=CARTESIAN_POINT('Ctrl Pts',(1.92453321512435,-42.9740309956624,15.));
#22069=CARTESIAN_POINT('Ctrl Pts',(1.97016390194215,-42.8820834139973,15.));
#22070=CARTESIAN_POINT('Ctrl Pts',(2.01528067528089,-42.7900301875309,15.));
#22071=CARTESIAN_POINT('Ctrl Pts',(2.05988014924518,-42.6978725343209,15.));
#22072=CARTESIAN_POINT('Ctrl Pts',(2.1039588640177,-42.6056116373455,15.));
#22073=CARTESIAN_POINT('Ctrl Pts',(2.14751319676745,-42.5132487024335,15.));
#22074=CARTESIAN_POINT('Ctrl Pts',(2.19053924976737,-42.4207850290047,15.));
#22075=CARTESIAN_POINT('Ctrl Pts',(2.23303287465499,-42.3282220118033,15.));
#22076=CARTESIAN_POINT('Ctrl Pts',(2.27498976664773,-42.2355611060784,15.));
#22077=CARTESIAN_POINT('Ctrl Pts',(2.31640554742808,-42.1428038039937,15.));
#22078=CARTESIAN_POINT('Ctrl Pts',(2.35727584066428,-42.0499516093661,15.));
#22079=CARTESIAN_POINT('Ctrl Pts',(2.39759639399648,-41.9570060084039,15.));
#22080=CARTESIAN_POINT('Ctrl Pts',(2.437363014342,-41.8639684667923,15.));
#22081=CARTESIAN_POINT('Ctrl Pts',(2.47657137427692,-41.7708404467533,15.));
#22082=CARTESIAN_POINT('Ctrl Pts',(2.51521684674476,-41.6776234194583,15.));
#22083=CARTESIAN_POINT('Ctrl Pts',(2.55329436064183,-41.5843188786284,15.));
#22084=CARTESIAN_POINT('Ctrl Pts',(2.59079818040171,-41.4909283577703,15.));
#22085=CARTESIAN_POINT('Ctrl Pts',(2.62772200460655,-41.3974534325936,15.));
#22086=CARTESIAN_POINT('Ctrl Pts',(2.66405934050117,-41.3038957096306,15.));
#22087=CARTESIAN_POINT('Ctrl Pts',(2.69980383625015,-41.2102568187956,15.));
#22088=CARTESIAN_POINT('Ctrl Pts',(2.73494956725005,-41.1165384061145,15.));
#22089=CARTESIAN_POINT('Ctrl Pts',(2.76949151194863,-41.0227421242398,15.));
#22090=CARTESIAN_POINT('Ctrl Pts',(2.80342531768404,-40.9288696352159,15.));
#22091=CARTESIAN_POINT('Ctrl Pts',(2.83674635946678,-40.8349226258683,15.));
#22092=CARTESIAN_POINT('Ctrl Pts',(2.86944892209897,-40.7409028213129,15.));
#22093=CARTESIAN_POINT('Ctrl Pts',(2.90152548734342,-40.6468119976928,15.));
#22094=CARTESIAN_POINT('Ctrl Pts',(2.93296560822893,-40.5526520010651,15.));
#22095=CARTESIAN_POINT('Ctrl Pts',(2.96375636417322,-40.4584247445196,15.));
#22096=CARTESIAN_POINT('Ctrl Pts',(2.99388446458219,-40.3641321823444,15.));
#22097=CARTESIAN_POINT('Ctrl Pts',(3.02333808901594,-40.2697762886113,15.));
#22098=CARTESIAN_POINT('Ctrl Pts',(3.0521084742307,-40.1753590391515,15.));
#22099=CARTESIAN_POINT('Ctrl Pts',(3.08019251155015,-40.0808823811787,15.));
#22100=CARTESIAN_POINT('Ctrl Pts',(3.10759149802907,-39.9863482523153,15.));
#22101=CARTESIAN_POINT('Ctrl Pts',(3.13430604330355,-39.8917586491576,15.));
#22102=CARTESIAN_POINT('Ctrl Pts',(3.16033160752803,-39.7971156880138,15.));
#22103=CARTESIAN_POINT('Ctrl Pts',(3.18565465503835,-39.7024216585552,15.));
#22104=CARTESIAN_POINT('Ctrl Pts',(3.21024640045595,-39.607679107639,15.));
#22105=CARTESIAN_POINT('Ctrl Pts',(3.2340660969166,-39.5128908052622,15.));
#22106=CARTESIAN_POINT('Ctrl Pts',(3.25707264313387,-39.4180596080755,15.));
#22107=CARTESIAN_POINT('Ctrl Pts',(3.27923485388116,-39.3231883392913,15.));
#22108=CARTESIAN_POINT('Ctrl Pts',(3.30054018081687,-39.2282796893977,15.));
#22109=CARTESIAN_POINT('Ctrl Pts',(3.32100933979557,-39.1333360409949,15.));
#22110=CARTESIAN_POINT('Ctrl Pts',(3.34068601264472,-39.0383596151636,15.));
#22111=CARTESIAN_POINT('Ctrl Pts',(3.3596092279948,-38.9433528420174,15.));
#22112=CARTESIAN_POINT('Ctrl Pts',(3.37778863054481,-38.8483186930884,15.));
#22113=CARTESIAN_POINT('Ctrl Pts',(3.39518333281817,-38.7532609709905,15.));
#22114=CARTESIAN_POINT('Ctrl Pts',(3.411667175119,-38.6581847668347,15.));
#22115=CARTESIAN_POINT('Ctrl Pts',(3.42705871084996,-38.5630961226878,15.));
#22116=CARTESIAN_POINT('Ctrl Pts',(3.44118343200302,-38.4680013094732,15.));
#22117=CARTESIAN_POINT('Ctrl Pts',(3.45393053211022,-38.3729061502716,15.));
#22118=CARTESIAN_POINT('Ctrl Pts',(3.46530185256872,-38.2778154909527,15.));
#22119=CARTESIAN_POINT('Ctrl Pts',(3.47549027265411,-38.1827321816559,15.));
#22120=CARTESIAN_POINT('Ctrl Pts',(3.48478279878233,-38.0876589224537,15.));
#22121=CARTESIAN_POINT('Ctrl Pts',(3.49340804454645,-37.9926009950482,15.));
#22122=CARTESIAN_POINT('Ctrl Pts',(3.50139628556083,-37.8975688353863,15.));
#22123=CARTESIAN_POINT('Ctrl Pts',(3.50844720825127,-37.8025803811856,15.));
#22124=CARTESIAN_POINT('Ctrl Pts',(3.51375922979957,-37.7076643105286,15.));
#22125=CARTESIAN_POINT('Ctrl Pts',(3.51624243734644,-37.6128545966533,15.));
#22126=CARTESIAN_POINT('Ctrl Pts',(3.51508109065209,-37.5371179004295,15.));
#22127=CARTESIAN_POINT('Ctrl Pts',(3.5120473187636,-37.4803889700239,15.));
#22128=CARTESIAN_POINT('Ctrl Pts',(3.50901346997656,-37.4426037737699,15.));
#22129=CARTESIAN_POINT('Ctrl Pts',(3.50724370857672,-37.4237196983922,15.));
#22130=CARTESIAN_POINT('',(1.38952890043928,-43.9780537249529,0.));
#22131=CARTESIAN_POINT('Origin',(-2.01948391736579E-27,-1.13331566353736E-11,
0.));
#22132=CARTESIAN_POINT('',(-1.38952890043917,-43.9780537249529,0.));
#22133=CARTESIAN_POINT('Origin',(-2.01948391736579E-27,-1.13331566353736E-11,
0.));
#22134=CARTESIAN_POINT('',(-1.38952890043917,-43.9780537249529,15.));
#22135=CARTESIAN_POINT('Origin',(-2.01948391736579E-27,-1.13331566353736E-11,
15.));
#22136=CARTESIAN_POINT('',(-1.38952890043917,-43.9780537249529,0.));
#22137=CARTESIAN_POINT('Ctrl Pts',(-3.50724370857673,-37.4237196983922,
0.));
#22138=CARTESIAN_POINT('Ctrl Pts',(-3.50724370857673,-37.4237196983922,
18.));
#22139=CARTESIAN_POINT('Ctrl Pts',(-3.50901346997657,-37.4426037737699,
0.));
#22140=CARTESIAN_POINT('Ctrl Pts',(-3.50901346997657,-37.4426037737699,
18.));
#22141=CARTESIAN_POINT('Ctrl Pts',(-3.51204731876362,-37.4803889700239,
0.));
#22142=CARTESIAN_POINT('Ctrl Pts',(-3.51204731876362,-37.4803889700239,
18.));
#22143=CARTESIAN_POINT('Ctrl Pts',(-3.51508109065211,-37.5371179004295,
0.));
#22144=CARTESIAN_POINT('Ctrl Pts',(-3.51508109065211,-37.5371179004295,
18.));
#22145=CARTESIAN_POINT('Ctrl Pts',(-3.51624243734646,-37.6128545966533,
0.));
#22146=CARTESIAN_POINT('Ctrl Pts',(-3.51624243734646,-37.6128545966533,
18.));
#22147=CARTESIAN_POINT('Ctrl Pts',(-3.51375922979958,-37.7076643105286,
0.));
#22148=CARTESIAN_POINT('Ctrl Pts',(-3.51375922979958,-37.7076643105286,
18.));
#22149=CARTESIAN_POINT('Ctrl Pts',(-3.50844720825129,-37.8025803811856,
0.));
#22150=CARTESIAN_POINT('Ctrl Pts',(-3.50844720825129,-37.8025803811856,
18.));
#22151=CARTESIAN_POINT('Ctrl Pts',(-3.50139628556084,-37.8975688353863,
0.));
#22152=CARTESIAN_POINT('Ctrl Pts',(-3.50139628556084,-37.8975688353863,
18.));
#22153=CARTESIAN_POINT('Ctrl Pts',(-3.49340804454646,-37.9926009950482,
0.));
#22154=CARTESIAN_POINT('Ctrl Pts',(-3.49340804454646,-37.9926009950482,
18.));
#22155=CARTESIAN_POINT('Ctrl Pts',(-3.48478279878234,-38.0876589224537,
0.));
#22156=CARTESIAN_POINT('Ctrl Pts',(-3.48478279878234,-38.0876589224537,
18.));
#22157=CARTESIAN_POINT('Ctrl Pts',(-3.47549027265412,-38.1827321816559,
0.));
#22158=CARTESIAN_POINT('Ctrl Pts',(-3.47549027265412,-38.1827321816559,
18.));
#22159=CARTESIAN_POINT('Ctrl Pts',(-3.46530185256873,-38.2778154909527,
0.));
#22160=CARTESIAN_POINT('Ctrl Pts',(-3.46530185256873,-38.2778154909527,
18.));
#22161=CARTESIAN_POINT('Ctrl Pts',(-3.45393053211023,-38.3729061502716,
0.));
#22162=CARTESIAN_POINT('Ctrl Pts',(-3.45393053211023,-38.3729061502716,
18.));
#22163=CARTESIAN_POINT('Ctrl Pts',(-3.44118343200304,-38.4680013094732,
0.));
#22164=CARTESIAN_POINT('Ctrl Pts',(-3.44118343200304,-38.4680013094732,
18.));
#22165=CARTESIAN_POINT('Ctrl Pts',(-3.42705871084998,-38.5630961226878,
0.));
#22166=CARTESIAN_POINT('Ctrl Pts',(-3.42705871084998,-38.5630961226878,
18.));
#22167=CARTESIAN_POINT('Ctrl Pts',(-3.41166717511902,-38.6581847668347,
0.));
#22168=CARTESIAN_POINT('Ctrl Pts',(-3.41166717511902,-38.6581847668347,
18.));
#22169=CARTESIAN_POINT('Ctrl Pts',(-3.39518333281819,-38.7532609709905,
0.));
#22170=CARTESIAN_POINT('Ctrl Pts',(-3.39518333281819,-38.7532609709905,
18.));
#22171=CARTESIAN_POINT('Ctrl Pts',(-3.37778863054483,-38.8483186930884,
0.));
#22172=CARTESIAN_POINT('Ctrl Pts',(-3.37778863054483,-38.8483186930884,
18.));
#22173=CARTESIAN_POINT('Ctrl Pts',(-3.35960922799482,-38.9433528420174,
0.));
#22174=CARTESIAN_POINT('Ctrl Pts',(-3.35960922799482,-38.9433528420174,
18.));
#22175=CARTESIAN_POINT('Ctrl Pts',(-3.34068601264473,-39.0383596151636,
0.));
#22176=CARTESIAN_POINT('Ctrl Pts',(-3.34068601264473,-39.0383596151636,
18.));
#22177=CARTESIAN_POINT('Ctrl Pts',(-3.32100933979558,-39.1333360409949,
0.));
#22178=CARTESIAN_POINT('Ctrl Pts',(-3.32100933979558,-39.1333360409949,
18.));
#22179=CARTESIAN_POINT('Ctrl Pts',(-3.30054018081688,-39.2282796893977,
0.));
#22180=CARTESIAN_POINT('Ctrl Pts',(-3.30054018081688,-39.2282796893977,
18.));
#22181=CARTESIAN_POINT('Ctrl Pts',(-3.27923485388118,-39.3231883392913,
0.));
#22182=CARTESIAN_POINT('Ctrl Pts',(-3.27923485388118,-39.3231883392913,
18.));
#22183=CARTESIAN_POINT('Ctrl Pts',(-3.25707264313389,-39.4180596080755,
0.));
#22184=CARTESIAN_POINT('Ctrl Pts',(-3.25707264313389,-39.4180596080755,
18.));
#22185=CARTESIAN_POINT('Ctrl Pts',(-3.23406609691662,-39.5128908052622,
0.));
#22186=CARTESIAN_POINT('Ctrl Pts',(-3.23406609691662,-39.5128908052622,
18.));
#22187=CARTESIAN_POINT('Ctrl Pts',(-3.21024640045596,-39.607679107639,0.));
#22188=CARTESIAN_POINT('Ctrl Pts',(-3.21024640045596,-39.607679107639,18.));
#22189=CARTESIAN_POINT('Ctrl Pts',(-3.18565465503836,-39.7024216585552,
0.));
#22190=CARTESIAN_POINT('Ctrl Pts',(-3.18565465503836,-39.7024216585552,
18.));
#22191=CARTESIAN_POINT('Ctrl Pts',(-3.16033160752805,-39.7971156880138,
0.));
#22192=CARTESIAN_POINT('Ctrl Pts',(-3.16033160752805,-39.7971156880138,
18.));
#22193=CARTESIAN_POINT('Ctrl Pts',(-3.13430604330357,-39.8917586491576,
0.));
#22194=CARTESIAN_POINT('Ctrl Pts',(-3.13430604330357,-39.8917586491576,
18.));
#22195=CARTESIAN_POINT('Ctrl Pts',(-3.10759149802909,-39.9863482523153,
0.));
#22196=CARTESIAN_POINT('Ctrl Pts',(-3.10759149802909,-39.9863482523153,
18.));
#22197=CARTESIAN_POINT('Ctrl Pts',(-3.08019251155016,-40.0808823811787,
0.));
#22198=CARTESIAN_POINT('Ctrl Pts',(-3.08019251155016,-40.0808823811787,
18.));
#22199=CARTESIAN_POINT('Ctrl Pts',(-3.05210847423072,-40.1753590391515,
0.));
#22200=CARTESIAN_POINT('Ctrl Pts',(-3.05210847423072,-40.1753590391515,
18.));
#22201=CARTESIAN_POINT('Ctrl Pts',(-3.02333808901596,-40.2697762886113,
0.));
#22202=CARTESIAN_POINT('Ctrl Pts',(-3.02333808901596,-40.2697762886113,
18.));
#22203=CARTESIAN_POINT('Ctrl Pts',(-2.9938844645822,-40.3641321823444,0.));
#22204=CARTESIAN_POINT('Ctrl Pts',(-2.9938844645822,-40.3641321823444,18.));
#22205=CARTESIAN_POINT('Ctrl Pts',(-2.96375636417323,-40.4584247445196,
0.));
#22206=CARTESIAN_POINT('Ctrl Pts',(-2.96375636417323,-40.4584247445196,
18.));
#22207=CARTESIAN_POINT('Ctrl Pts',(-2.93296560822894,-40.5526520010651,
0.));
#22208=CARTESIAN_POINT('Ctrl Pts',(-2.93296560822894,-40.5526520010651,
18.));
#22209=CARTESIAN_POINT('Ctrl Pts',(-2.90152548734344,-40.6468119976928,
0.));
#22210=CARTESIAN_POINT('Ctrl Pts',(-2.90152548734344,-40.6468119976928,
18.));
#22211=CARTESIAN_POINT('Ctrl Pts',(-2.86944892209898,-40.7409028213129,
0.));
#22212=CARTESIAN_POINT('Ctrl Pts',(-2.86944892209898,-40.7409028213129,
18.));
#22213=CARTESIAN_POINT('Ctrl Pts',(-2.8367463594668,-40.8349226258683,0.));
#22214=CARTESIAN_POINT('Ctrl Pts',(-2.8367463594668,-40.8349226258683,18.));
#22215=CARTESIAN_POINT('Ctrl Pts',(-2.80342531768406,-40.9288696352159,
0.));
#22216=CARTESIAN_POINT('Ctrl Pts',(-2.80342531768406,-40.9288696352159,
18.));
#22217=CARTESIAN_POINT('Ctrl Pts',(-2.76949151194864,-41.0227421242398,
0.));
#22218=CARTESIAN_POINT('Ctrl Pts',(-2.76949151194864,-41.0227421242398,
18.));
#22219=CARTESIAN_POINT('Ctrl Pts',(-2.73494956725006,-41.1165384061145,
0.));
#22220=CARTESIAN_POINT('Ctrl Pts',(-2.73494956725006,-41.1165384061145,
18.));
#22221=CARTESIAN_POINT('Ctrl Pts',(-2.69980383625016,-41.2102568187956,
0.));
#22222=CARTESIAN_POINT('Ctrl Pts',(-2.69980383625016,-41.2102568187956,
18.));
#22223=CARTESIAN_POINT('Ctrl Pts',(-2.66405934050119,-41.3038957096306,
0.));
#22224=CARTESIAN_POINT('Ctrl Pts',(-2.66405934050119,-41.3038957096306,
18.));
#22225=CARTESIAN_POINT('Ctrl Pts',(-2.62772200460657,-41.3974534325936,
0.));
#22226=CARTESIAN_POINT('Ctrl Pts',(-2.62772200460657,-41.3974534325936,
18.));
#22227=CARTESIAN_POINT('Ctrl Pts',(-2.59079818040173,-41.4909283577703,
0.));
#22228=CARTESIAN_POINT('Ctrl Pts',(-2.59079818040173,-41.4909283577703,
18.));
#22229=CARTESIAN_POINT('Ctrl Pts',(-2.55329436064185,-41.5843188786284,
0.));
#22230=CARTESIAN_POINT('Ctrl Pts',(-2.55329436064185,-41.5843188786284,
18.));
#22231=CARTESIAN_POINT('Ctrl Pts',(-2.51521684674478,-41.6776234194583,
0.));
#22232=CARTESIAN_POINT('Ctrl Pts',(-2.51521684674478,-41.6776234194583,
18.));
#22233=CARTESIAN_POINT('Ctrl Pts',(-2.47657137427694,-41.7708404467533,
0.));
#22234=CARTESIAN_POINT('Ctrl Pts',(-2.47657137427694,-41.7708404467533,
18.));
#22235=CARTESIAN_POINT('Ctrl Pts',(-2.43736301434201,-41.8639684667923,
0.));
#22236=CARTESIAN_POINT('Ctrl Pts',(-2.43736301434201,-41.8639684667923,
18.));
#22237=CARTESIAN_POINT('Ctrl Pts',(-2.39759639399649,-41.9570060084039,
0.));
#22238=CARTESIAN_POINT('Ctrl Pts',(-2.39759639399649,-41.9570060084039,
18.));
#22239=CARTESIAN_POINT('Ctrl Pts',(-2.3572758406643,-42.0499516093661,0.));
#22240=CARTESIAN_POINT('Ctrl Pts',(-2.3572758406643,-42.0499516093661,18.));
#22241=CARTESIAN_POINT('Ctrl Pts',(-2.3164055474281,-42.1428038039937,0.));
#22242=CARTESIAN_POINT('Ctrl Pts',(-2.3164055474281,-42.1428038039937,18.));
#22243=CARTESIAN_POINT('Ctrl Pts',(-2.27498976664775,-42.2355611060784,
0.));
#22244=CARTESIAN_POINT('Ctrl Pts',(-2.27498976664775,-42.2355611060784,
18.));
#22245=CARTESIAN_POINT('Ctrl Pts',(-2.23303287465501,-42.3282220118033,
0.));
#22246=CARTESIAN_POINT('Ctrl Pts',(-2.23303287465501,-42.3282220118033,
18.));
#22247=CARTESIAN_POINT('Ctrl Pts',(-2.19053924976738,-42.4207850290047,
0.));
#22248=CARTESIAN_POINT('Ctrl Pts',(-2.19053924976738,-42.4207850290047,
18.));
#22249=CARTESIAN_POINT('Ctrl Pts',(-2.14751319676746,-42.5132487024335,
0.));
#22250=CARTESIAN_POINT('Ctrl Pts',(-2.14751319676746,-42.5132487024335,
18.));
#22251=CARTESIAN_POINT('Ctrl Pts',(-2.10395886401772,-42.6056116373455,
0.));
#22252=CARTESIAN_POINT('Ctrl Pts',(-2.10395886401772,-42.6056116373455,
18.));
#22253=CARTESIAN_POINT('Ctrl Pts',(-2.0598801492452,-42.6978725343209,0.));
#22254=CARTESIAN_POINT('Ctrl Pts',(-2.0598801492452,-42.6978725343209,18.));
#22255=CARTESIAN_POINT('Ctrl Pts',(-2.0152806752809,-42.7900301875309,0.));
#22256=CARTESIAN_POINT('Ctrl Pts',(-2.0152806752809,-42.7900301875309,18.));
#22257=CARTESIAN_POINT('Ctrl Pts',(-1.97016390194217,-42.8820834139973,
0.));
#22258=CARTESIAN_POINT('Ctrl Pts',(-1.97016390194217,-42.8820834139973,
18.));
#22259=CARTESIAN_POINT('Ctrl Pts',(-1.92453321512437,-42.9740309956624,
0.));
#22260=CARTESIAN_POINT('Ctrl Pts',(-1.92453321512437,-42.9740309956624,
18.));
#22261=CARTESIAN_POINT('Ctrl Pts',(-1.8783920201461,-43.065871623255,0.));
#22262=CARTESIAN_POINT('Ctrl Pts',(-1.8783920201461,-43.065871623255,18.));
#22263=CARTESIAN_POINT('Ctrl Pts',(-1.83174385734712,-43.1576038253643,
0.));
#22264=CARTESIAN_POINT('Ctrl Pts',(-1.83174385734712,-43.1576038253643,
18.));
#22265=CARTESIAN_POINT('Ctrl Pts',(-1.78459244842771,-43.2492259505872,
0.));
#22266=CARTESIAN_POINT('Ctrl Pts',(-1.78459244842771,-43.2492259505872,
18.));
#22267=CARTESIAN_POINT('Ctrl Pts',(-1.73694151741125,-43.3407363140236,
0.));
#22268=CARTESIAN_POINT('Ctrl Pts',(-1.73694151741125,-43.3407363140236,
18.));
#22269=CARTESIAN_POINT('Ctrl Pts',(-1.68879465270609,-43.4321333178711,
0.));
#22270=CARTESIAN_POINT('Ctrl Pts',(-1.68879465270609,-43.4321333178711,
18.));
#22271=CARTESIAN_POINT('Ctrl Pts',(-1.64015515906649,-43.5234155788248,
0.));
#22272=CARTESIAN_POINT('Ctrl Pts',(-1.64015515906649,-43.5234155788248,
18.));
#22273=CARTESIAN_POINT('Ctrl Pts',(-1.59102591108105,-43.6145820637333,
0.));
#22274=CARTESIAN_POINT('Ctrl Pts',(-1.59102591108105,-43.6145820637333,
18.));
#22275=CARTESIAN_POINT('Ctrl Pts',(-1.54140922714765,-43.7056321934163,
0.));
#22276=CARTESIAN_POINT('Ctrl Pts',(-1.54140922714765,-43.7056321934163,
18.));
#22277=CARTESIAN_POINT('Ctrl Pts',(-1.49130689006068,-43.7965657112708,
0.));
#22278=CARTESIAN_POINT('Ctrl Pts',(-1.49130689006068,-43.7965657112708,
18.));
#22279=CARTESIAN_POINT('Ctrl Pts',(-1.45083750111683,-43.8692192047561,
0.));
#22280=CARTESIAN_POINT('Ctrl Pts',(-1.45083750111683,-43.8692192047561,
18.));
#22281=CARTESIAN_POINT('Ctrl Pts',(-1.42026781296157,-43.9236568607623,
0.));
#22282=CARTESIAN_POINT('Ctrl Pts',(-1.42026781296157,-43.9236568607623,
18.));
#22283=CARTESIAN_POINT('Ctrl Pts',(-1.39979132121932,-43.9599253218251,
0.));
#22284=CARTESIAN_POINT('Ctrl Pts',(-1.39979132121932,-43.9599253218251,
18.));
#22285=CARTESIAN_POINT('Ctrl Pts',(-1.38952890043917,-43.9780537249529,
0.));
#22286=CARTESIAN_POINT('Ctrl Pts',(-1.38952890043917,-43.9780537249529,
18.));
#22287=CARTESIAN_POINT('Ctrl Pts',(-3.50724370857673,-37.4237196983922,
0.));
#22288=CARTESIAN_POINT('Ctrl Pts',(-3.50901346997657,-37.4426037737699,
0.));
#22289=CARTESIAN_POINT('Ctrl Pts',(-3.51204731876362,-37.4803889700239,
0.));
#22290=CARTESIAN_POINT('Ctrl Pts',(-3.51508109065211,-37.5371179004295,
0.));
#22291=CARTESIAN_POINT('Ctrl Pts',(-3.51624243734646,-37.6128545966533,
0.));
#22292=CARTESIAN_POINT('Ctrl Pts',(-3.51375922979958,-37.7076643105286,
0.));
#22293=CARTESIAN_POINT('Ctrl Pts',(-3.50844720825129,-37.8025803811856,
0.));
#22294=CARTESIAN_POINT('Ctrl Pts',(-3.50139628556084,-37.8975688353863,
0.));
#22295=CARTESIAN_POINT('Ctrl Pts',(-3.49340804454646,-37.9926009950482,
0.));
#22296=CARTESIAN_POINT('Ctrl Pts',(-3.48478279878234,-38.0876589224537,
0.));
#22297=CARTESIAN_POINT('Ctrl Pts',(-3.47549027265412,-38.1827321816559,
0.));
#22298=CARTESIAN_POINT('Ctrl Pts',(-3.46530185256873,-38.2778154909527,
0.));
#22299=CARTESIAN_POINT('Ctrl Pts',(-3.45393053211023,-38.3729061502716,
0.));
#22300=CARTESIAN_POINT('Ctrl Pts',(-3.44118343200304,-38.4680013094732,
0.));
#22301=CARTESIAN_POINT('Ctrl Pts',(-3.42705871084998,-38.5630961226878,
0.));
#22302=CARTESIAN_POINT('Ctrl Pts',(-3.41166717511902,-38.6581847668347,
0.));
#22303=CARTESIAN_POINT('Ctrl Pts',(-3.39518333281819,-38.7532609709905,
0.));
#22304=CARTESIAN_POINT('Ctrl Pts',(-3.37778863054483,-38.8483186930884,
0.));
#22305=CARTESIAN_POINT('Ctrl Pts',(-3.35960922799482,-38.9433528420174,
0.));
#22306=CARTESIAN_POINT('Ctrl Pts',(-3.34068601264473,-39.0383596151636,
0.));
#22307=CARTESIAN_POINT('Ctrl Pts',(-3.32100933979558,-39.1333360409949,
0.));
#22308=CARTESIAN_POINT('Ctrl Pts',(-3.30054018081688,-39.2282796893977,
0.));
#22309=CARTESIAN_POINT('Ctrl Pts',(-3.27923485388118,-39.3231883392913,
0.));
#22310=CARTESIAN_POINT('Ctrl Pts',(-3.25707264313389,-39.4180596080755,
0.));
#22311=CARTESIAN_POINT('Ctrl Pts',(-3.23406609691662,-39.5128908052622,
0.));
#22312=CARTESIAN_POINT('Ctrl Pts',(-3.21024640045596,-39.607679107639,0.));
#22313=CARTESIAN_POINT('Ctrl Pts',(-3.18565465503836,-39.7024216585552,
0.));
#22314=CARTESIAN_POINT('Ctrl Pts',(-3.16033160752805,-39.7971156880138,
0.));
#22315=CARTESIAN_POINT('Ctrl Pts',(-3.13430604330357,-39.8917586491576,
0.));
#22316=CARTESIAN_POINT('Ctrl Pts',(-3.10759149802909,-39.9863482523153,
0.));
#22317=CARTESIAN_POINT('Ctrl Pts',(-3.08019251155016,-40.0808823811787,
0.));
#22318=CARTESIAN_POINT('Ctrl Pts',(-3.05210847423072,-40.1753590391515,
0.));
#22319=CARTESIAN_POINT('Ctrl Pts',(-3.02333808901596,-40.2697762886113,
0.));
#22320=CARTESIAN_POINT('Ctrl Pts',(-2.9938844645822,-40.3641321823444,0.));
#22321=CARTESIAN_POINT('Ctrl Pts',(-2.96375636417323,-40.4584247445196,
0.));
#22322=CARTESIAN_POINT('Ctrl Pts',(-2.93296560822894,-40.5526520010651,
0.));
#22323=CARTESIAN_POINT('Ctrl Pts',(-2.90152548734344,-40.6468119976928,
0.));
#22324=CARTESIAN_POINT('Ctrl Pts',(-2.86944892209898,-40.7409028213129,
0.));
#22325=CARTESIAN_POINT('Ctrl Pts',(-2.8367463594668,-40.8349226258683,0.));
#22326=CARTESIAN_POINT('Ctrl Pts',(-2.80342531768406,-40.9288696352159,
0.));
#22327=CARTESIAN_POINT('Ctrl Pts',(-2.76949151194864,-41.0227421242398,
0.));
#22328=CARTESIAN_POINT('Ctrl Pts',(-2.73494956725006,-41.1165384061145,
0.));
#22329=CARTESIAN_POINT('Ctrl Pts',(-2.69980383625016,-41.2102568187956,
0.));
#22330=CARTESIAN_POINT('Ctrl Pts',(-2.66405934050119,-41.3038957096306,
0.));
#22331=CARTESIAN_POINT('Ctrl Pts',(-2.62772200460657,-41.3974534325936,
0.));
#22332=CARTESIAN_POINT('Ctrl Pts',(-2.59079818040173,-41.4909283577703,
0.));
#22333=CARTESIAN_POINT('Ctrl Pts',(-2.55329436064185,-41.5843188786284,
0.));
#22334=CARTESIAN_POINT('Ctrl Pts',(-2.51521684674478,-41.6776234194583,
0.));
#22335=CARTESIAN_POINT('Ctrl Pts',(-2.47657137427694,-41.7708404467533,
0.));
#22336=CARTESIAN_POINT('Ctrl Pts',(-2.43736301434201,-41.8639684667923,
0.));
#22337=CARTESIAN_POINT('Ctrl Pts',(-2.39759639399649,-41.9570060084039,
0.));
#22338=CARTESIAN_POINT('Ctrl Pts',(-2.3572758406643,-42.0499516093661,0.));
#22339=CARTESIAN_POINT('Ctrl Pts',(-2.3164055474281,-42.1428038039937,0.));
#22340=CARTESIAN_POINT('Ctrl Pts',(-2.27498976664775,-42.2355611060784,
0.));
#22341=CARTESIAN_POINT('Ctrl Pts',(-2.23303287465501,-42.3282220118033,
0.));
#22342=CARTESIAN_POINT('Ctrl Pts',(-2.19053924976738,-42.4207850290047,
0.));
#22343=CARTESIAN_POINT('Ctrl Pts',(-2.14751319676746,-42.5132487024335,
0.));
#22344=CARTESIAN_POINT('Ctrl Pts',(-2.10395886401772,-42.6056116373455,
0.));
#22345=CARTESIAN_POINT('Ctrl Pts',(-2.0598801492452,-42.6978725343209,0.));
#22346=CARTESIAN_POINT('Ctrl Pts',(-2.0152806752809,-42.7900301875309,0.));
#22347=CARTESIAN_POINT('Ctrl Pts',(-1.97016390194217,-42.8820834139973,
0.));
#22348=CARTESIAN_POINT('Ctrl Pts',(-1.92453321512437,-42.9740309956624,
0.));
#22349=CARTESIAN_POINT('Ctrl Pts',(-1.8783920201461,-43.065871623255,0.));
#22350=CARTESIAN_POINT('Ctrl Pts',(-1.83174385734712,-43.1576038253643,
0.));
#22351=CARTESIAN_POINT('Ctrl Pts',(-1.78459244842771,-43.2492259505872,
0.));
#22352=CARTESIAN_POINT('Ctrl Pts',(-1.73694151741125,-43.3407363140236,
0.));
#22353=CARTESIAN_POINT('Ctrl Pts',(-1.68879465270609,-43.4321333178711,
0.));
#22354=CARTESIAN_POINT('Ctrl Pts',(-1.64015515906649,-43.5234155788248,
0.));
#22355=CARTESIAN_POINT('Ctrl Pts',(-1.59102591108105,-43.6145820637333,
0.));
#22356=CARTESIAN_POINT('Ctrl Pts',(-1.53148589036097,-43.7238422193529,
0.));
#22357=CARTESIAN_POINT('Ctrl Pts',(-1.48126213998561,-43.8147465842503,
0.));
#22358=CARTESIAN_POINT('Ctrl Pts',(-1.44069595482724,-43.8873767449247,
0.));
#22359=CARTESIAN_POINT('Ctrl Pts',(-1.41005374202874,-43.9417969186811,
0.));
#22360=CARTESIAN_POINT('Ctrl Pts',(-1.38952890043917,-43.9780537249529,
0.));
#22361=CARTESIAN_POINT('Ctrl Pts',(-3.50724370857673,-37.4237196983922,
15.));
#22362=CARTESIAN_POINT('Ctrl Pts',(-3.50901346997657,-37.4426037737699,
15.));
#22363=CARTESIAN_POINT('Ctrl Pts',(-3.51204731876362,-37.4803889700239,
15.));
#22364=CARTESIAN_POINT('Ctrl Pts',(-3.51508109065211,-37.5371179004295,
15.));
#22365=CARTESIAN_POINT('Ctrl Pts',(-3.51624243734646,-37.6128545966533,
15.));
#22366=CARTESIAN_POINT('Ctrl Pts',(-3.51375922979958,-37.7076643105286,
15.));
#22367=CARTESIAN_POINT('Ctrl Pts',(-3.50844720825129,-37.8025803811856,
15.));
#22368=CARTESIAN_POINT('Ctrl Pts',(-3.50139628556084,-37.8975688353863,
15.));
#22369=CARTESIAN_POINT('Ctrl Pts',(-3.49340804454646,-37.9926009950482,
15.));
#22370=CARTESIAN_POINT('Ctrl Pts',(-3.48478279878234,-38.0876589224537,
15.));
#22371=CARTESIAN_POINT('Ctrl Pts',(-3.47549027265412,-38.1827321816559,
15.));
#22372=CARTESIAN_POINT('Ctrl Pts',(-3.46530185256873,-38.2778154909527,
15.));
#22373=CARTESIAN_POINT('Ctrl Pts',(-3.45393053211023,-38.3729061502716,
15.));
#22374=CARTESIAN_POINT('Ctrl Pts',(-3.44118343200304,-38.4680013094732,
15.));
#22375=CARTESIAN_POINT('Ctrl Pts',(-3.42705871084998,-38.5630961226878,
15.));
#22376=CARTESIAN_POINT('Ctrl Pts',(-3.41166717511902,-38.6581847668347,
15.));
#22377=CARTESIAN_POINT('Ctrl Pts',(-3.39518333281819,-38.7532609709905,
15.));
#22378=CARTESIAN_POINT('Ctrl Pts',(-3.37778863054483,-38.8483186930884,
15.));
#22379=CARTESIAN_POINT('Ctrl Pts',(-3.35960922799482,-38.9433528420174,
15.));
#22380=CARTESIAN_POINT('Ctrl Pts',(-3.34068601264473,-39.0383596151636,
15.));
#22381=CARTESIAN_POINT('Ctrl Pts',(-3.32100933979558,-39.1333360409949,
15.));
#22382=CARTESIAN_POINT('Ctrl Pts',(-3.30054018081688,-39.2282796893977,
15.));
#22383=CARTESIAN_POINT('Ctrl Pts',(-3.27923485388118,-39.3231883392913,
15.));
#22384=CARTESIAN_POINT('Ctrl Pts',(-3.25707264313389,-39.4180596080755,
15.));
#22385=CARTESIAN_POINT('Ctrl Pts',(-3.23406609691662,-39.5128908052622,
15.));
#22386=CARTESIAN_POINT('Ctrl Pts',(-3.21024640045596,-39.607679107639,15.));
#22387=CARTESIAN_POINT('Ctrl Pts',(-3.18565465503836,-39.7024216585552,
15.));
#22388=CARTESIAN_POINT('Ctrl Pts',(-3.16033160752805,-39.7971156880138,
15.));
#22389=CARTESIAN_POINT('Ctrl Pts',(-3.13430604330357,-39.8917586491576,
15.));
#22390=CARTESIAN_POINT('Ctrl Pts',(-3.10759149802909,-39.9863482523153,
15.));
#22391=CARTESIAN_POINT('Ctrl Pts',(-3.08019251155016,-40.0808823811787,
15.));
#22392=CARTESIAN_POINT('Ctrl Pts',(-3.05210847423072,-40.1753590391515,
15.));
#22393=CARTESIAN_POINT('Ctrl Pts',(-3.02333808901596,-40.2697762886113,
15.));
#22394=CARTESIAN_POINT('Ctrl Pts',(-2.9938844645822,-40.3641321823444,15.));
#22395=CARTESIAN_POINT('Ctrl Pts',(-2.96375636417323,-40.4584247445196,
15.));
#22396=CARTESIAN_POINT('Ctrl Pts',(-2.93296560822894,-40.5526520010651,
15.));
#22397=CARTESIAN_POINT('Ctrl Pts',(-2.90152548734344,-40.6468119976928,
15.));
#22398=CARTESIAN_POINT('Ctrl Pts',(-2.86944892209898,-40.7409028213129,
15.));
#22399=CARTESIAN_POINT('Ctrl Pts',(-2.8367463594668,-40.8349226258683,15.));
#22400=CARTESIAN_POINT('Ctrl Pts',(-2.80342531768406,-40.9288696352159,
15.));
#22401=CARTESIAN_POINT('Ctrl Pts',(-2.76949151194864,-41.0227421242398,
15.));
#22402=CARTESIAN_POINT('Ctrl Pts',(-2.73494956725006,-41.1165384061145,
15.));
#22403=CARTESIAN_POINT('Ctrl Pts',(-2.69980383625016,-41.2102568187956,
15.));
#22404=CARTESIAN_POINT('Ctrl Pts',(-2.66405934050119,-41.3038957096306,
15.));
#22405=CARTESIAN_POINT('Ctrl Pts',(-2.62772200460657,-41.3974534325936,
15.));
#22406=CARTESIAN_POINT('Ctrl Pts',(-2.59079818040173,-41.4909283577703,
15.));
#22407=CARTESIAN_POINT('Ctrl Pts',(-2.55329436064185,-41.5843188786284,
15.));
#22408=CARTESIAN_POINT('Ctrl Pts',(-2.51521684674478,-41.6776234194583,
15.));
#22409=CARTESIAN_POINT('Ctrl Pts',(-2.47657137427694,-41.7708404467533,
15.));
#22410=CARTESIAN_POINT('Ctrl Pts',(-2.43736301434201,-41.8639684667923,
15.));
#22411=CARTESIAN_POINT('Ctrl Pts',(-2.39759639399649,-41.9570060084039,
15.));
#22412=CARTESIAN_POINT('Ctrl Pts',(-2.3572758406643,-42.0499516093661,15.));
#22413=CARTESIAN_POINT('Ctrl Pts',(-2.3164055474281,-42.1428038039937,15.));
#22414=CARTESIAN_POINT('Ctrl Pts',(-2.27498976664775,-42.2355611060784,
15.));
#22415=CARTESIAN_POINT('Ctrl Pts',(-2.23303287465501,-42.3282220118033,
15.));
#22416=CARTESIAN_POINT('Ctrl Pts',(-2.19053924976738,-42.4207850290047,
15.));
#22417=CARTESIAN_POINT('Ctrl Pts',(-2.14751319676746,-42.5132487024335,
15.));
#22418=CARTESIAN_POINT('Ctrl Pts',(-2.10395886401772,-42.6056116373455,
15.));
#22419=CARTESIAN_POINT('Ctrl Pts',(-2.0598801492452,-42.6978725343209,15.));
#22420=CARTESIAN_POINT('Ctrl Pts',(-2.0152806752809,-42.7900301875309,15.));
#22421=CARTESIAN_POINT('Ctrl Pts',(-1.97016390194217,-42.8820834139973,
15.));
#22422=CARTESIAN_POINT('Ctrl Pts',(-1.92453321512437,-42.9740309956624,
15.));
#22423=CARTESIAN_POINT('Ctrl Pts',(-1.8783920201461,-43.065871623255,15.));
#22424=CARTESIAN_POINT('Ctrl Pts',(-1.83174385734712,-43.1576038253643,
15.));
#22425=CARTESIAN_POINT('Ctrl Pts',(-1.78459244842771,-43.2492259505872,
15.));
#22426=CARTESIAN_POINT('Ctrl Pts',(-1.73694151741125,-43.3407363140236,
15.));
#22427=CARTESIAN_POINT('Ctrl Pts',(-1.68879465270609,-43.4321333178711,
15.));
#22428=CARTESIAN_POINT('Ctrl Pts',(-1.64015515906649,-43.5234155788248,
15.));
#22429=CARTESIAN_POINT('Ctrl Pts',(-1.59102591108105,-43.6145820637333,
15.));
#22430=CARTESIAN_POINT('Ctrl Pts',(-1.53148589036097,-43.7238422193529,
15.));
#22431=CARTESIAN_POINT('Ctrl Pts',(-1.48126213998561,-43.8147465842503,
15.));
#22432=CARTESIAN_POINT('Ctrl Pts',(-1.44069595482724,-43.8873767449247,
15.));
#22433=CARTESIAN_POINT('Ctrl Pts',(-1.41005374202874,-43.9417969186811,
15.));
#22434=CARTESIAN_POINT('Ctrl Pts',(-1.38952890043917,-43.9780537249529,
15.));
#22435=CARTESIAN_POINT('Ctrl Pts',(-12.2684454652018,-42.2550026135057,
0.));
#22436=CARTESIAN_POINT('Ctrl Pts',(-12.2684454652018,-42.2550026135057,
18.));
#22437=CARTESIAN_POINT('Ctrl Pts',(-12.2530833383985,-42.2409327400055,
0.));
#22438=CARTESIAN_POINT('Ctrl Pts',(-12.2530833383985,-42.2409327400055,
18.));
#22439=CARTESIAN_POINT('Ctrl Pts',(-12.222401466668,-42.2127669677092,0.));
#22440=CARTESIAN_POINT('Ctrl Pts',(-12.222401466668,-42.2127669677092,18.));
#22441=CARTESIAN_POINT('Ctrl Pts',(-12.1765058047069,-42.1704402333854,
0.));
#22442=CARTESIAN_POINT('Ctrl Pts',(-12.1765058047069,-42.1704402333854,
18.));
#22443=CARTESIAN_POINT('Ctrl Pts',(-12.1155659644537,-42.1138483839101,
0.));
#22444=CARTESIAN_POINT('Ctrl Pts',(-12.1155659644537,-42.1138483839101,
18.));
#22445=CARTESIAN_POINT('Ctrl Pts',(-12.0398158079102,-42.0428479428228,
0.));
#22446=CARTESIAN_POINT('Ctrl Pts',(-12.0398158079102,-42.0428479428228,
18.));
#22447=CARTESIAN_POINT('Ctrl Pts',(-11.9644914999263,-41.9715865222182,
0.));
#22448=CARTESIAN_POINT('Ctrl Pts',(-11.9644914999263,-41.9715865222182,
18.));
#22449=CARTESIAN_POINT('Ctrl Pts',(-11.8895948153349,-41.9000638152266,
0.));
#22450=CARTESIAN_POINT('Ctrl Pts',(-11.8895948153349,-41.9000638152266,
18.));
#22451=CARTESIAN_POINT('Ctrl Pts',(-11.81512813804,-41.8282796562569,0.));
#22452=CARTESIAN_POINT('Ctrl Pts',(-11.81512813804,-41.8282796562569,18.));
#22453=CARTESIAN_POINT('Ctrl Pts',(-11.7410945211992,-41.7562341395977,
0.));
#22454=CARTESIAN_POINT('Ctrl Pts',(-11.7410945211992,-41.7562341395977,
18.));
#22455=CARTESIAN_POINT('Ctrl Pts',(-11.6674975352852,-41.6839275596248,
0.));
#22456=CARTESIAN_POINT('Ctrl Pts',(-11.6674975352852,-41.6839275596248,
18.));
#22457=CARTESIAN_POINT('Ctrl Pts',(-11.5943410868252,-41.6113603270596,
0.));
#22458=CARTESIAN_POINT('Ctrl Pts',(-11.5943410868252,-41.6113603270596,
18.));
#22459=CARTESIAN_POINT('Ctrl Pts',(-11.5216292382388,-41.5385328935506,
0.));
#22460=CARTESIAN_POINT('Ctrl Pts',(-11.5216292382388,-41.5385328935506,
18.));
#22461=CARTESIAN_POINT('Ctrl Pts',(-11.449366039385,-41.4654456796071,0.));
#22462=CARTESIAN_POINT('Ctrl Pts',(-11.449366039385,-41.4654456796071,18.));
#22463=CARTESIAN_POINT('Ctrl Pts',(-11.3775553120177,-41.3920989905986,
0.));
#22464=CARTESIAN_POINT('Ctrl Pts',(-11.3775553120177,-41.3920989905986,
18.));
#22465=CARTESIAN_POINT('Ctrl Pts',(-11.3062006993745,-41.3184930194148,
0.));
#22466=CARTESIAN_POINT('Ctrl Pts',(-11.3062006993745,-41.3184930194148,
18.));
#22467=CARTESIAN_POINT('Ctrl Pts',(-11.2353057980338,-41.2446278781981,
0.));
#22468=CARTESIAN_POINT('Ctrl Pts',(-11.2353057980338,-41.2446278781981,
18.));
#22469=CARTESIAN_POINT('Ctrl Pts',(-11.1648742640378,-41.1705036228854,
0.));
#22470=CARTESIAN_POINT('Ctrl Pts',(-11.1648742640378,-41.1705036228854,
18.));
#22471=CARTESIAN_POINT('Ctrl Pts',(-11.0949099155251,-41.0961202807715,
0.));
#22472=CARTESIAN_POINT('Ctrl Pts',(-11.0949099155251,-41.0961202807715,
18.));
#22473=CARTESIAN_POINT('Ctrl Pts',(-11.0254168609972,-41.0214778832142,
0.));
#22474=CARTESIAN_POINT('Ctrl Pts',(-11.0254168609972,-41.0214778832142,
18.));
#22475=CARTESIAN_POINT('Ctrl Pts',(-10.956399476781,-40.9465764747798,0.));
#22476=CARTESIAN_POINT('Ctrl Pts',(-10.956399476781,-40.9465764747798,18.));
#22477=CARTESIAN_POINT('Ctrl Pts',(-10.8878623066647,-40.8714161092412,
0.));
#22478=CARTESIAN_POINT('Ctrl Pts',(-10.8878623066647,-40.8714161092412,
18.));
#22479=CARTESIAN_POINT('Ctrl Pts',(-10.8198099757795,-40.7959968527561,
0.));
#22480=CARTESIAN_POINT('Ctrl Pts',(-10.8198099757795,-40.7959968527561,
18.));
#22481=CARTESIAN_POINT('Ctrl Pts',(-10.7522471109694,-40.7203187831783,
0.));
#22482=CARTESIAN_POINT('Ctrl Pts',(-10.7522471109694,-40.7203187831783,
18.));
#22483=CARTESIAN_POINT('Ctrl Pts',(-10.6851782157325,-40.6443819999244,
0.));
#22484=CARTESIAN_POINT('Ctrl Pts',(-10.6851782157325,-40.6443819999244,
18.));
#22485=CARTESIAN_POINT('Ctrl Pts',(-10.618607730849,-40.5681866012103,0.));
#22486=CARTESIAN_POINT('Ctrl Pts',(-10.618607730849,-40.5681866012103,18.));
#22487=CARTESIAN_POINT('Ctrl Pts',(-10.5525402237951,-40.4917326404439,
0.));
#22488=CARTESIAN_POINT('Ctrl Pts',(-10.5525402237951,-40.4917326404439,
18.));
#22489=CARTESIAN_POINT('Ctrl Pts',(-10.48698054978,-40.4150200869536,0.));
#22490=CARTESIAN_POINT('Ctrl Pts',(-10.48698054978,-40.4150200869536,18.));
#22491=CARTESIAN_POINT('Ctrl Pts',(-10.4219339932951,-40.3380487942952,
0.));
#22492=CARTESIAN_POINT('Ctrl Pts',(-10.4219339932951,-40.3380487942952,
18.));
#22493=CARTESIAN_POINT('Ctrl Pts',(-10.3574064830678,-40.2608184485326,
0.));
#22494=CARTESIAN_POINT('Ctrl Pts',(-10.3574064830678,-40.2608184485326,
18.));
#22495=CARTESIAN_POINT('Ctrl Pts',(-10.2934044990237,-40.1833286010098,
0.));
#22496=CARTESIAN_POINT('Ctrl Pts',(-10.2934044990237,-40.1833286010098,
18.));
#22497=CARTESIAN_POINT('Ctrl Pts',(-10.2299347125857,-40.1055787732578,
0.));
#22498=CARTESIAN_POINT('Ctrl Pts',(-10.2299347125857,-40.1055787732578,
18.));
#22499=CARTESIAN_POINT('Ctrl Pts',(-10.1670036683795,-40.0275685525923,
0.));
#22500=CARTESIAN_POINT('Ctrl Pts',(-10.1670036683795,-40.0275685525923,
18.));
#22501=CARTESIAN_POINT('Ctrl Pts',(-10.1046175096878,-39.9492976736738,
0.));
#22502=CARTESIAN_POINT('Ctrl Pts',(-10.1046175096878,-39.9492976736738,
18.));
#22503=CARTESIAN_POINT('Ctrl Pts',(-10.0427815229883,-39.8707661565233,
0.));
#22504=CARTESIAN_POINT('Ctrl Pts',(-10.0427815229883,-39.8707661565233,
18.));
#22505=CARTESIAN_POINT('Ctrl Pts',(-9.98150036150824,-39.7919742367922,
0.));
#22506=CARTESIAN_POINT('Ctrl Pts',(-9.98150036150824,-39.7919742367922,
18.));
#22507=CARTESIAN_POINT('Ctrl Pts',(-9.92077894513193,-39.712922089547,0.));
#22508=CARTESIAN_POINT('Ctrl Pts',(-9.92077894513193,-39.712922089547,18.));
#22509=CARTESIAN_POINT('Ctrl Pts',(-9.86062324242561,-39.6336095893767,
0.));
#22510=CARTESIAN_POINT('Ctrl Pts',(-9.86062324242561,-39.6336095893767,
18.));
#22511=CARTESIAN_POINT('Ctrl Pts',(-9.80104095251614,-39.5540361022309,
0.));
#22512=CARTESIAN_POINT('Ctrl Pts',(-9.80104095251614,-39.5540361022309,
18.));
#22513=CARTESIAN_POINT('Ctrl Pts',(-9.74204258152664,-39.4742001555227,
0.));
#22514=CARTESIAN_POINT('Ctrl Pts',(-9.74204258152664,-39.4742001555227,
18.));
#22515=CARTESIAN_POINT('Ctrl Pts',(-9.68364100883828,-39.3940995760289,
0.));
#22516=CARTESIAN_POINT('Ctrl Pts',(-9.68364100883828,-39.3940995760289,
18.));
#22517=CARTESIAN_POINT('Ctrl Pts',(-9.62584947846544,-39.3137321153686,
0.));
#22518=CARTESIAN_POINT('Ctrl Pts',(-9.62584947846544,-39.3137321153686,
18.));
#22519=CARTESIAN_POINT('Ctrl Pts',(-9.56867984233624,-39.2330959982788,
0.));
#22520=CARTESIAN_POINT('Ctrl Pts',(-9.56867984233624,-39.2330959982788,
18.));
#22521=CARTESIAN_POINT('Ctrl Pts',(-9.51214104535621,-39.1521903958955,
0.));
#22522=CARTESIAN_POINT('Ctrl Pts',(-9.51214104535621,-39.1521903958955,
18.));
#22523=CARTESIAN_POINT('Ctrl Pts',(-9.45623664577432,-39.0710161994951,
0.));
#22524=CARTESIAN_POINT('Ctrl Pts',(-9.45623664577432,-39.0710161994951,
18.));
#22525=CARTESIAN_POINT('Ctrl Pts',(-9.40096600877644,-38.9895756526779,
0.));
#22526=CARTESIAN_POINT('Ctrl Pts',(-9.40096600877644,-38.9895756526779,
18.));
#22527=CARTESIAN_POINT('Ctrl Pts',(-9.34632917154637,-38.9078708427078,
0.));
#22528=CARTESIAN_POINT('Ctrl Pts',(-9.34632917154637,-38.9078708427078,
18.));
#22529=CARTESIAN_POINT('Ctrl Pts',(-9.29233110570904,-38.8259023794241,
0.));
#22530=CARTESIAN_POINT('Ctrl Pts',(-9.29233110570904,-38.8259023794241,
18.));
#22531=CARTESIAN_POINT('Ctrl Pts',(-9.23898539199332,-38.7436682576832,
0.));
#22532=CARTESIAN_POINT('Ctrl Pts',(-9.23898539199332,-38.7436682576832,
18.));
#22533=CARTESIAN_POINT('Ctrl Pts',(-9.1863201939433,-38.6611620045193,0.));
#22534=CARTESIAN_POINT('Ctrl Pts',(-9.1863201939433,-38.6611620045193,18.));
#22535=CARTESIAN_POINT('Ctrl Pts',(-9.13437512010587,-38.5783736628826,
0.));
#22536=CARTESIAN_POINT('Ctrl Pts',(-9.13437512010587,-38.5783736628826,
18.));
#22537=CARTESIAN_POINT('Ctrl Pts',(-9.08319014288087,-38.4952932486131,
0.));
#22538=CARTESIAN_POINT('Ctrl Pts',(-9.08319014288087,-38.4952932486131,
18.));
#22539=CARTESIAN_POINT('Ctrl Pts',(-9.03279579360191,-38.4119138099805,
0.));
#22540=CARTESIAN_POINT('Ctrl Pts',(-9.03279579360191,-38.4119138099805,
18.));
#22541=CARTESIAN_POINT('Ctrl Pts',(-8.98320483785761,-38.3282340281403,
0.));
#22542=CARTESIAN_POINT('Ctrl Pts',(-8.98320483785761,-38.3282340281403,
18.));
#22543=CARTESIAN_POINT('Ctrl Pts',(-8.9343983099634,-38.2442625706309,0.));
#22544=CARTESIAN_POINT('Ctrl Pts',(-8.9343983099634,-38.2442625706309,18.));
#22545=CARTESIAN_POINT('Ctrl Pts',(-8.88633535238435,-38.1600150482528,
0.));
#22546=CARTESIAN_POINT('Ctrl Pts',(-8.88633535238435,-38.1600150482528,
18.));
#22547=CARTESIAN_POINT('Ctrl Pts',(-8.8389795976335,-38.0755058326913,0.));
#22548=CARTESIAN_POINT('Ctrl Pts',(-8.8389795976335,-38.0755058326913,18.));
#22549=CARTESIAN_POINT('Ctrl Pts',(-8.79232279131093,-37.9907407304174,
0.));
#22550=CARTESIAN_POINT('Ctrl Pts',(-8.79232279131093,-37.9907407304174,
18.));
#22551=CARTESIAN_POINT('Ctrl Pts',(-8.74640499479003,-37.9057107230066,
0.));
#22552=CARTESIAN_POINT('Ctrl Pts',(-8.74640499479003,-37.9057107230066,
18.));
#22553=CARTESIAN_POINT('Ctrl Pts',(-8.70134776631144,-37.8203816669031,
0.));
#22554=CARTESIAN_POINT('Ctrl Pts',(-8.70134776631144,-37.8203816669031,
18.));
#22555=CARTESIAN_POINT('Ctrl Pts',(-8.65732553894525,-37.7347032383719,
0.));
#22556=CARTESIAN_POINT('Ctrl Pts',(-8.65732553894525,-37.7347032383719,
18.));
#22557=CARTESIAN_POINT('Ctrl Pts',(-8.61450621749156,-37.6486274754754,
0.));
#22558=CARTESIAN_POINT('Ctrl Pts',(-8.61450621749156,-37.6486274754754,
18.));
#22559=CARTESIAN_POINT('Ctrl Pts',(-8.57299698459467,-37.5621256752108,
0.));
#22560=CARTESIAN_POINT('Ctrl Pts',(-8.57299698459467,-37.5621256752108,
18.));
#22561=CARTESIAN_POINT('Ctrl Pts',(-8.53279758643785,-37.4752030152968,
0.));
#22562=CARTESIAN_POINT('Ctrl Pts',(-8.53279758643785,-37.4752030152968,
18.));
#22563=CARTESIAN_POINT('Ctrl Pts',(-8.49372546467076,-37.3879218093514,
0.));
#22564=CARTESIAN_POINT('Ctrl Pts',(-8.49372546467076,-37.3879218093514,
18.));
#22565=CARTESIAN_POINT('Ctrl Pts',(-8.45550849433961,-37.3003733151561,
0.));
#22566=CARTESIAN_POINT('Ctrl Pts',(-8.45550849433961,-37.3003733151561,
18.));
#22567=CARTESIAN_POINT('Ctrl Pts',(-8.41793088313261,-37.2126332013933,
0.));
#22568=CARTESIAN_POINT('Ctrl Pts',(-8.41793088313261,-37.2126332013933,
18.));
#22569=CARTESIAN_POINT('Ctrl Pts',(-8.38096706211449,-37.1247207489179,
0.));
#22570=CARTESIAN_POINT('Ctrl Pts',(-8.38096706211449,-37.1247207489179,
18.));
#22571=CARTESIAN_POINT('Ctrl Pts',(-8.3449081895264,-37.0365602155148,0.));
#22572=CARTESIAN_POINT('Ctrl Pts',(-8.3449081895264,-37.0365602155148,18.));
#22573=CARTESIAN_POINT('Ctrl Pts',(-8.31052547794592,-36.9479311729484,
0.));
#22574=CARTESIAN_POINT('Ctrl Pts',(-8.31052547794592,-36.9479311729484,
18.));
#22575=CARTESIAN_POINT('Ctrl Pts',(-8.27886599440786,-36.8585291300917,
0.));
#22576=CARTESIAN_POINT('Ctrl Pts',(-8.27886599440786,-36.8585291300917,
18.));
#22577=CARTESIAN_POINT('Ctrl Pts',(-8.25656657451821,-36.7861403757604,
0.));
#22578=CARTESIAN_POINT('Ctrl Pts',(-8.25656657451821,-36.7861403757604,
18.));
#22579=CARTESIAN_POINT('Ctrl Pts',(-8.24192165947368,-36.7312504697652,
0.));
#22580=CARTESIAN_POINT('Ctrl Pts',(-8.24192165947368,-36.7312504697652,
18.));
#22581=CARTESIAN_POINT('Ctrl Pts',(-8.23313075335377,-36.6943771018148,
0.));
#22582=CARTESIAN_POINT('Ctrl Pts',(-8.23313075335377,-36.6943771018148,
18.));
#22583=CARTESIAN_POINT('Ctrl Pts',(-8.22897839625062,-36.6758703925241,
0.));
#22584=CARTESIAN_POINT('Ctrl Pts',(-8.22897839625062,-36.6758703925241,
18.));
#22585=CARTESIAN_POINT('',(-12.2684454652017,-42.2550026135057,0.));
#22586=CARTESIAN_POINT('Ctrl Pts',(-8.22897839625062,-36.6758703925241,
0.));
#22587=CARTESIAN_POINT('Ctrl Pts',(-8.23313075335377,-36.6943771018148,
0.));
#22588=CARTESIAN_POINT('Ctrl Pts',(-8.24192165947368,-36.7312504697652,
0.));
#22589=CARTESIAN_POINT('Ctrl Pts',(-8.25656657451821,-36.7861403757604,
0.));
#22590=CARTESIAN_POINT('Ctrl Pts',(-8.27886599440786,-36.8585291300917,
0.));
#22591=CARTESIAN_POINT('Ctrl Pts',(-8.31052547794592,-36.9479311729484,
0.));
#22592=CARTESIAN_POINT('Ctrl Pts',(-8.3449081895264,-37.0365602155148,0.));
#22593=CARTESIAN_POINT('Ctrl Pts',(-8.38096706211449,-37.1247207489179,
0.));
#22594=CARTESIAN_POINT('Ctrl Pts',(-8.41793088313261,-37.2126332013933,
0.));
#22595=CARTESIAN_POINT('Ctrl Pts',(-8.45550849433961,-37.3003733151561,
0.));
#22596=CARTESIAN_POINT('Ctrl Pts',(-8.49372546467076,-37.3879218093514,
0.));
#22597=CARTESIAN_POINT('Ctrl Pts',(-8.53279758643785,-37.4752030152968,
0.));
#22598=CARTESIAN_POINT('Ctrl Pts',(-8.57299698459467,-37.5621256752108,
0.));
#22599=CARTESIAN_POINT('Ctrl Pts',(-8.61450621749156,-37.6486274754754,
0.));
#22600=CARTESIAN_POINT('Ctrl Pts',(-8.65732553894525,-37.7347032383719,
0.));
#22601=CARTESIAN_POINT('Ctrl Pts',(-8.70134776631144,-37.8203816669031,
0.));
#22602=CARTESIAN_POINT('Ctrl Pts',(-8.74640499479003,-37.9057107230066,
0.));
#22603=CARTESIAN_POINT('Ctrl Pts',(-8.79232279131093,-37.9907407304174,
0.));
#22604=CARTESIAN_POINT('Ctrl Pts',(-8.8389795976335,-38.0755058326913,0.));
#22605=CARTESIAN_POINT('Ctrl Pts',(-8.88633535238435,-38.1600150482528,
0.));
#22606=CARTESIAN_POINT('Ctrl Pts',(-8.9343983099634,-38.2442625706309,0.));
#22607=CARTESIAN_POINT('Ctrl Pts',(-8.98320483785761,-38.3282340281403,
0.));
#22608=CARTESIAN_POINT('Ctrl Pts',(-9.03279579360191,-38.4119138099805,
0.));
#22609=CARTESIAN_POINT('Ctrl Pts',(-9.08319014288087,-38.4952932486131,
0.));
#22610=CARTESIAN_POINT('Ctrl Pts',(-9.13437512010587,-38.5783736628826,
0.));
#22611=CARTESIAN_POINT('Ctrl Pts',(-9.1863201939433,-38.6611620045193,0.));
#22612=CARTESIAN_POINT('Ctrl Pts',(-9.23898539199332,-38.7436682576832,
0.));
#22613=CARTESIAN_POINT('Ctrl Pts',(-9.29233110570904,-38.8259023794241,
0.));
#22614=CARTESIAN_POINT('Ctrl Pts',(-9.34632917154637,-38.9078708427078,
0.));
#22615=CARTESIAN_POINT('Ctrl Pts',(-9.40096600877644,-38.9895756526779,
0.));
#22616=CARTESIAN_POINT('Ctrl Pts',(-9.45623664577432,-39.0710161994951,
0.));
#22617=CARTESIAN_POINT('Ctrl Pts',(-9.51214104535621,-39.1521903958955,
0.));
#22618=CARTESIAN_POINT('Ctrl Pts',(-9.56867984233624,-39.2330959982788,
0.));
#22619=CARTESIAN_POINT('Ctrl Pts',(-9.62584947846544,-39.3137321153686,
0.));
#22620=CARTESIAN_POINT('Ctrl Pts',(-9.68364100883828,-39.3940995760289,
0.));
#22621=CARTESIAN_POINT('Ctrl Pts',(-9.74204258152664,-39.4742001555227,
0.));
#22622=CARTESIAN_POINT('Ctrl Pts',(-9.80104095251614,-39.5540361022309,
0.));
#22623=CARTESIAN_POINT('Ctrl Pts',(-9.86062324242561,-39.6336095893767,
0.));
#22624=CARTESIAN_POINT('Ctrl Pts',(-9.92077894513193,-39.712922089547,0.));
#22625=CARTESIAN_POINT('Ctrl Pts',(-9.98150036150824,-39.7919742367922,
0.));
#22626=CARTESIAN_POINT('Ctrl Pts',(-10.0427815229883,-39.8707661565233,
0.));
#22627=CARTESIAN_POINT('Ctrl Pts',(-10.1046175096878,-39.9492976736738,
0.));
#22628=CARTESIAN_POINT('Ctrl Pts',(-10.1670036683795,-40.0275685525923,
0.));
#22629=CARTESIAN_POINT('Ctrl Pts',(-10.2299347125857,-40.1055787732578,
0.));
#22630=CARTESIAN_POINT('Ctrl Pts',(-10.2934044990237,-40.1833286010098,
0.));
#22631=CARTESIAN_POINT('Ctrl Pts',(-10.3574064830678,-40.2608184485326,
0.));
#22632=CARTESIAN_POINT('Ctrl Pts',(-10.4219339932951,-40.3380487942952,
0.));
#22633=CARTESIAN_POINT('Ctrl Pts',(-10.48698054978,-40.4150200869536,0.));
#22634=CARTESIAN_POINT('Ctrl Pts',(-10.5525402237951,-40.4917326404439,
0.));
#22635=CARTESIAN_POINT('Ctrl Pts',(-10.618607730849,-40.5681866012103,0.));
#22636=CARTESIAN_POINT('Ctrl Pts',(-10.6851782157325,-40.6443819999244,
0.));
#22637=CARTESIAN_POINT('Ctrl Pts',(-10.7522471109694,-40.7203187831783,
0.));
#22638=CARTESIAN_POINT('Ctrl Pts',(-10.8198099757795,-40.7959968527561,
0.));
#22639=CARTESIAN_POINT('Ctrl Pts',(-10.8878623066647,-40.8714161092412,
0.));
#22640=CARTESIAN_POINT('Ctrl Pts',(-10.956399476781,-40.9465764747798,0.));
#22641=CARTESIAN_POINT('Ctrl Pts',(-11.0254168609972,-41.0214778832142,
0.));
#22642=CARTESIAN_POINT('Ctrl Pts',(-11.0949099155251,-41.0961202807715,
0.));
#22643=CARTESIAN_POINT('Ctrl Pts',(-11.1648742640378,-41.1705036228854,
0.));
#22644=CARTESIAN_POINT('Ctrl Pts',(-11.2353057980338,-41.2446278781981,
0.));
#22645=CARTESIAN_POINT('Ctrl Pts',(-11.3062006993745,-41.3184930194148,
0.));
#22646=CARTESIAN_POINT('Ctrl Pts',(-11.3775553120177,-41.3920989905986,
0.));
#22647=CARTESIAN_POINT('Ctrl Pts',(-11.449366039385,-41.4654456796071,0.));
#22648=CARTESIAN_POINT('Ctrl Pts',(-11.5216292382388,-41.5385328935506,
0.));
#22649=CARTESIAN_POINT('Ctrl Pts',(-11.5943410868252,-41.6113603270596,
0.));
#22650=CARTESIAN_POINT('Ctrl Pts',(-11.6674975352852,-41.6839275596248,
0.));
#22651=CARTESIAN_POINT('Ctrl Pts',(-11.7410945211992,-41.7562341395977,
0.));
#22652=CARTESIAN_POINT('Ctrl Pts',(-11.81512813804,-41.8282796562569,0.));
#22653=CARTESIAN_POINT('Ctrl Pts',(-11.8895948153349,-41.9000638152266,
0.));
#22654=CARTESIAN_POINT('Ctrl Pts',(-11.9644914999263,-41.9715865222182,
0.));
#22655=CARTESIAN_POINT('Ctrl Pts',(-12.054880669507,-42.0571002269437,0.));
#22656=CARTESIAN_POINT('Ctrl Pts',(-12.1307372881904,-42.1280354231517,
0.));
#22657=CARTESIAN_POINT('Ctrl Pts',(-12.1917619768791,-42.18457517013,0.));
#22658=CARTESIAN_POINT('Ctrl Pts',(-12.2377212115625,-42.2268628664988,
0.));
#22659=CARTESIAN_POINT('Ctrl Pts',(-12.2684454652018,-42.2550026135057,
0.));
#22660=CARTESIAN_POINT('',(-12.2684454652017,-42.2550026135057,15.));
#22661=CARTESIAN_POINT('Ctrl Pts',(-12.2684454652018,-42.2550026135057,
15.));
#22662=CARTESIAN_POINT('Ctrl Pts',(-12.2530833383985,-42.2409327400055,
15.));
#22663=CARTESIAN_POINT('Ctrl Pts',(-12.222401466668,-42.2127669677092,15.));
#22664=CARTESIAN_POINT('Ctrl Pts',(-12.1765058047069,-42.1704402333854,
15.));
#22665=CARTESIAN_POINT('Ctrl Pts',(-12.1155659644537,-42.1138483839101,
15.));
#22666=CARTESIAN_POINT('Ctrl Pts',(-12.0398158079102,-42.0428479428228,
15.));
#22667=CARTESIAN_POINT('Ctrl Pts',(-11.9644914999263,-41.9715865222182,
15.));
#22668=CARTESIAN_POINT('Ctrl Pts',(-11.8895948153349,-41.9000638152266,
15.));
#22669=CARTESIAN_POINT('Ctrl Pts',(-11.81512813804,-41.8282796562569,15.));
#22670=CARTESIAN_POINT('Ctrl Pts',(-11.7410945211992,-41.7562341395977,
15.));
#22671=CARTESIAN_POINT('Ctrl Pts',(-11.6674975352852,-41.6839275596248,
15.));
#22672=CARTESIAN_POINT('Ctrl Pts',(-11.5943410868252,-41.6113603270596,
15.));
#22673=CARTESIAN_POINT('Ctrl Pts',(-11.5216292382388,-41.5385328935506,
15.));
#22674=CARTESIAN_POINT('Ctrl Pts',(-11.449366039385,-41.4654456796071,15.));
#22675=CARTESIAN_POINT('Ctrl Pts',(-11.3775553120177,-41.3920989905986,
15.));
#22676=CARTESIAN_POINT('Ctrl Pts',(-11.3062006993745,-41.3184930194148,
15.));
#22677=CARTESIAN_POINT('Ctrl Pts',(-11.2353057980338,-41.2446278781981,
15.));
#22678=CARTESIAN_POINT('Ctrl Pts',(-11.1648742640378,-41.1705036228854,
15.));
#22679=CARTESIAN_POINT('Ctrl Pts',(-11.0949099155251,-41.0961202807715,
15.));
#22680=CARTESIAN_POINT('Ctrl Pts',(-11.0254168609972,-41.0214778832142,
15.));
#22681=CARTESIAN_POINT('Ctrl Pts',(-10.956399476781,-40.9465764747798,15.));
#22682=CARTESIAN_POINT('Ctrl Pts',(-10.8878623066647,-40.8714161092412,
15.));
#22683=CARTESIAN_POINT('Ctrl Pts',(-10.8198099757795,-40.7959968527561,
15.));
#22684=CARTESIAN_POINT('Ctrl Pts',(-10.7522471109694,-40.7203187831783,
15.));
#22685=CARTESIAN_POINT('Ctrl Pts',(-10.6851782157325,-40.6443819999244,
15.));
#22686=CARTESIAN_POINT('Ctrl Pts',(-10.618607730849,-40.5681866012103,15.));
#22687=CARTESIAN_POINT('Ctrl Pts',(-10.5525402237951,-40.4917326404439,
15.));
#22688=CARTESIAN_POINT('Ctrl Pts',(-10.48698054978,-40.4150200869536,15.));
#22689=CARTESIAN_POINT('Ctrl Pts',(-10.4219339932951,-40.3380487942952,
15.));
#22690=CARTESIAN_POINT('Ctrl Pts',(-10.3574064830678,-40.2608184485326,
15.));
#22691=CARTESIAN_POINT('Ctrl Pts',(-10.2934044990237,-40.1833286010098,
15.));
#22692=CARTESIAN_POINT('Ctrl Pts',(-10.2299347125857,-40.1055787732578,
15.));
#22693=CARTESIAN_POINT('Ctrl Pts',(-10.1670036683795,-40.0275685525923,
15.));
#22694=CARTESIAN_POINT('Ctrl Pts',(-10.1046175096878,-39.9492976736738,
15.));
#22695=CARTESIAN_POINT('Ctrl Pts',(-10.0427815229883,-39.8707661565233,
15.));
#22696=CARTESIAN_POINT('Ctrl Pts',(-9.98150036150824,-39.7919742367922,
15.));
#22697=CARTESIAN_POINT('Ctrl Pts',(-9.92077894513193,-39.712922089547,15.));
#22698=CARTESIAN_POINT('Ctrl Pts',(-9.86062324242561,-39.6336095893767,
15.));
#22699=CARTESIAN_POINT('Ctrl Pts',(-9.80104095251614,-39.5540361022309,
15.));
#22700=CARTESIAN_POINT('Ctrl Pts',(-9.74204258152664,-39.4742001555227,
15.));
#22701=CARTESIAN_POINT('Ctrl Pts',(-9.68364100883828,-39.3940995760289,
15.));
#22702=CARTESIAN_POINT('Ctrl Pts',(-9.62584947846544,-39.3137321153686,
15.));
#22703=CARTESIAN_POINT('Ctrl Pts',(-9.56867984233624,-39.2330959982788,
15.));
#22704=CARTESIAN_POINT('Ctrl Pts',(-9.51214104535621,-39.1521903958955,
15.));
#22705=CARTESIAN_POINT('Ctrl Pts',(-9.45623664577432,-39.0710161994951,
15.));
#22706=CARTESIAN_POINT('Ctrl Pts',(-9.40096600877644,-38.9895756526779,
15.));
#22707=CARTESIAN_POINT('Ctrl Pts',(-9.34632917154637,-38.9078708427078,
15.));
#22708=CARTESIAN_POINT('Ctrl Pts',(-9.29233110570904,-38.8259023794241,
15.));
#22709=CARTESIAN_POINT('Ctrl Pts',(-9.23898539199332,-38.7436682576832,
15.));
#22710=CARTESIAN_POINT('Ctrl Pts',(-9.1863201939433,-38.6611620045193,15.));
#22711=CARTESIAN_POINT('Ctrl Pts',(-9.13437512010587,-38.5783736628826,
15.));
#22712=CARTESIAN_POINT('Ctrl Pts',(-9.08319014288087,-38.4952932486131,
15.));
#22713=CARTESIAN_POINT('Ctrl Pts',(-9.03279579360191,-38.4119138099805,
15.));
#22714=CARTESIAN_POINT('Ctrl Pts',(-8.98320483785761,-38.3282340281403,
15.));
#22715=CARTESIAN_POINT('Ctrl Pts',(-8.9343983099634,-38.2442625706309,15.));
#22716=CARTESIAN_POINT('Ctrl Pts',(-8.88633535238435,-38.1600150482528,
15.));
#22717=CARTESIAN_POINT('Ctrl Pts',(-8.8389795976335,-38.0755058326913,15.));
#22718=CARTESIAN_POINT('Ctrl Pts',(-8.79232279131093,-37.9907407304174,
15.));
#22719=CARTESIAN_POINT('Ctrl Pts',(-8.74640499479003,-37.9057107230066,
15.));
#22720=CARTESIAN_POINT('Ctrl Pts',(-8.70134776631144,-37.8203816669031,
15.));
#22721=CARTESIAN_POINT('Ctrl Pts',(-8.65732553894525,-37.7347032383719,
15.));
#22722=CARTESIAN_POINT('Ctrl Pts',(-8.61450621749156,-37.6486274754754,
15.));
#22723=CARTESIAN_POINT('Ctrl Pts',(-8.57299698459467,-37.5621256752108,
15.));
#22724=CARTESIAN_POINT('Ctrl Pts',(-8.53279758643785,-37.4752030152968,
15.));
#22725=CARTESIAN_POINT('Ctrl Pts',(-8.49372546467076,-37.3879218093514,
15.));
#22726=CARTESIAN_POINT('Ctrl Pts',(-8.45550849433961,-37.3003733151561,
15.));
#22727=CARTESIAN_POINT('Ctrl Pts',(-8.41793088313261,-37.2126332013933,
15.));
#22728=CARTESIAN_POINT('Ctrl Pts',(-8.38096706211449,-37.1247207489179,
15.));
#22729=CARTESIAN_POINT('Ctrl Pts',(-8.3449081895264,-37.0365602155148,15.));
#22730=CARTESIAN_POINT('Ctrl Pts',(-8.31052547794592,-36.9479311729484,
15.));
#22731=CARTESIAN_POINT('Ctrl Pts',(-8.27886599440786,-36.8585291300917,
15.));
#22732=CARTESIAN_POINT('Ctrl Pts',(-8.25656657451821,-36.7861403757604,
15.));
#22733=CARTESIAN_POINT('Ctrl Pts',(-8.24192165947368,-36.7312504697652,
15.));
#22734=CARTESIAN_POINT('Ctrl Pts',(-8.23313075335377,-36.6943771018148,
15.));
#22735=CARTESIAN_POINT('Ctrl Pts',(-8.22897839625062,-36.6758703925241,
15.));
#22736=CARTESIAN_POINT('',(-12.2684454652017,-42.2550026135057,0.));
#22737=CARTESIAN_POINT('Origin',(-3.50213800024364E-12,-1.07784724682657E-11,
0.));
#22738=CARTESIAN_POINT('',(-14.911486495888,-41.396226524684,0.));
#22739=CARTESIAN_POINT('Origin',(-3.50213800024364E-12,-1.07784724682657E-11,
0.));
#22740=CARTESIAN_POINT('',(-14.911486495888,-41.396226524684,15.));
#22741=CARTESIAN_POINT('Origin',(-3.50213800024364E-12,-1.07784724682657E-11,
15.));
#22742=CARTESIAN_POINT('',(-14.911486495888,-41.396226524684,0.));
#22743=CARTESIAN_POINT('Ctrl Pts',(-14.9001523628048,-34.5082745737944,
0.));
#22744=CARTESIAN_POINT('Ctrl Pts',(-14.9001523628048,-34.5082745737944,
18.));
#22745=CARTESIAN_POINT('Ctrl Pts',(-14.9076710061311,-34.525687510388,0.));
#22746=CARTESIAN_POINT('Ctrl Pts',(-14.9076710061311,-34.525687510388,18.));
#22747=CARTESIAN_POINT('Ctrl Pts',(-14.9222326355678,-34.5606858566713,
0.));
#22748=CARTESIAN_POINT('Ctrl Pts',(-14.9222326355678,-34.5606858566713,
18.));
#22749=CARTESIAN_POINT('Ctrl Pts',(-14.9426481276593,-34.6137007885254,
0.));
#22750=CARTESIAN_POINT('Ctrl Pts',(-14.9426481276593,-34.6137007885254,
18.));
#22751=CARTESIAN_POINT('Ctrl Pts',(-14.9671565602316,-34.6853717911268,
0.));
#22752=CARTESIAN_POINT('Ctrl Pts',(-14.9671565602316,-34.6853717911268,
18.));
#22753=CARTESIAN_POINT('Ctrl Pts',(-14.9940927023322,-34.7763085406486,
0.));
#22754=CARTESIAN_POINT('Ctrl Pts',(-14.9940927023322,-34.7763085406486,
18.));
#22755=CARTESIAN_POINT('Ctrl Pts',(-15.0183713484962,-34.8682205930809,
0.));
#22756=CARTESIAN_POINT('Ctrl Pts',(-15.0183713484962,-34.8682205930809,
18.));
#22757=CARTESIAN_POINT('Ctrl Pts',(-15.041018569143,-34.9607388363587,0.));
#22758=CARTESIAN_POINT('Ctrl Pts',(-15.041018569143,-34.9607388363587,18.));
#22759=CARTESIAN_POINT('Ctrl Pts',(-15.0627878528202,-35.0535882932913,
0.));
#22760=CARTESIAN_POINT('Ctrl Pts',(-15.0627878528202,-35.0535882932913,
18.));
#22761=CARTESIAN_POINT('Ctrl Pts',(-15.08395927165,-35.1466591020976,0.));
#22762=CARTESIAN_POINT('Ctrl Pts',(-15.08395927165,-35.1466591020976,18.));
#22763=CARTESIAN_POINT('Ctrl Pts',(-15.104500806927,-35.2399506932815,0.));
#22764=CARTESIAN_POINT('Ctrl Pts',(-15.104500806927,-35.2399506932815,18.));
#22765=CARTESIAN_POINT('Ctrl Pts',(-15.1241934020682,-35.3335286891314,
0.));
#22766=CARTESIAN_POINT('Ctrl Pts',(-15.1241934020682,-35.3335286891314,
18.));
#22767=CARTESIAN_POINT('Ctrl Pts',(-15.1427632633831,-35.4274792115856,
0.));
#22768=CARTESIAN_POINT('Ctrl Pts',(-15.1427632633831,-35.4274792115856,
18.));
#22769=CARTESIAN_POINT('Ctrl Pts',(-15.1600260710384,-35.5218591529745,
0.));
#22770=CARTESIAN_POINT('Ctrl Pts',(-15.1600260710384,-35.5218591529745,
18.));
#22771=CARTESIAN_POINT('Ctrl Pts',(-15.1759785763051,-35.6166644736253,
0.));
#22772=CARTESIAN_POINT('Ctrl Pts',(-15.1759785763051,-35.6166644736253,
18.));
#22773=CARTESIAN_POINT('Ctrl Pts',(-15.1907243629659,-35.7118553943773,
0.));
#22774=CARTESIAN_POINT('Ctrl Pts',(-15.1907243629659,-35.7118553943773,
18.));
#22775=CARTESIAN_POINT('Ctrl Pts',(-15.2044274601769,-35.8073720252878,
0.));
#22776=CARTESIAN_POINT('Ctrl Pts',(-15.2044274601769,-35.8073720252878,
18.));
#22777=CARTESIAN_POINT('Ctrl Pts',(-15.2172585668056,-35.9031525499277,
0.));
#22778=CARTESIAN_POINT('Ctrl Pts',(-15.2172585668056,-35.9031525499277,
18.));
#22779=CARTESIAN_POINT('Ctrl Pts',(-15.2293360946131,-35.9991531408727,
0.));
#22780=CARTESIAN_POINT('Ctrl Pts',(-15.2293360946131,-35.9991531408727,
18.));
#22781=CARTESIAN_POINT('Ctrl Pts',(-15.240697754828,-36.095357546697,0.));
#22782=CARTESIAN_POINT('Ctrl Pts',(-15.240697754828,-36.095357546697,18.));
#22783=CARTESIAN_POINT('Ctrl Pts',(-15.2513334565427,-36.1917659216814,
0.));
#22784=CARTESIAN_POINT('Ctrl Pts',(-15.2513334565427,-36.1917659216814,
18.));
#22785=CARTESIAN_POINT('Ctrl Pts',(-15.2612053303774,-36.2883880151607,
0.));
#22786=CARTESIAN_POINT('Ctrl Pts',(-15.2612053303774,-36.2883880151607,
18.));
#22787=CARTESIAN_POINT('Ctrl Pts',(-15.2702711460937,-36.3852352131887,
0.));
#22788=CARTESIAN_POINT('Ctrl Pts',(-15.2702711460937,-36.3852352131887,
18.));
#22789=CARTESIAN_POINT('Ctrl Pts',(-15.2785104654792,-36.4823116513289,
0.));
#22790=CARTESIAN_POINT('Ctrl Pts',(-15.2785104654792,-36.4823116513289,
18.));
#22791=CARTESIAN_POINT('Ctrl Pts',(-15.2859343913094,-36.5796108931244,
0.));
#22792=CARTESIAN_POINT('Ctrl Pts',(-15.2859343913094,-36.5796108931244,
18.));
#22793=CARTESIAN_POINT('Ctrl Pts',(-15.2925717100767,-36.6771206167755,
0.));
#22794=CARTESIAN_POINT('Ctrl Pts',(-15.2925717100767,-36.6771206167755,
18.));
#22795=CARTESIAN_POINT('Ctrl Pts',(-15.2984606286738,-36.7748254044502,
0.));
#22796=CARTESIAN_POINT('Ctrl Pts',(-15.2984606286738,-36.7748254044502,
18.));
#22797=CARTESIAN_POINT('Ctrl Pts',(-15.3036390436952,-36.8727100302512,
0.));
#22798=CARTESIAN_POINT('Ctrl Pts',(-15.3036390436952,-36.8727100302512,
18.));
#22799=CARTESIAN_POINT('Ctrl Pts',(-15.3081335446406,-36.970763176802,0.));
#22800=CARTESIAN_POINT('Ctrl Pts',(-15.3081335446406,-36.970763176802,18.));
#22801=CARTESIAN_POINT('Ctrl Pts',(-15.3119562971444,-37.0689784837457,
0.));
#22802=CARTESIAN_POINT('Ctrl Pts',(-15.3119562971444,-37.0689784837457,
18.));
#22803=CARTESIAN_POINT('Ctrl Pts',(-15.3151109648809,-37.1673525354641,
0.));
#22804=CARTESIAN_POINT('Ctrl Pts',(-15.3151109648809,-37.1673525354641,
18.));
#22805=CARTESIAN_POINT('Ctrl Pts',(-15.3175963510698,-37.2658836214694,
0.));
#22806=CARTESIAN_POINT('Ctrl Pts',(-15.3175963510698,-37.2658836214694,
18.));
#22807=CARTESIAN_POINT('Ctrl Pts',(-15.3194106233802,-37.3645702997848,
0.));
#22808=CARTESIAN_POINT('Ctrl Pts',(-15.3194106233802,-37.3645702997848,
18.));
#22809=CARTESIAN_POINT('Ctrl Pts',(-15.3205561366169,-37.4634097578665,
0.));
#22810=CARTESIAN_POINT('Ctrl Pts',(-15.3205561366169,-37.4634097578665,
18.));
#22811=CARTESIAN_POINT('Ctrl Pts',(-15.3210406145546,-37.562397408596,0.));
#22812=CARTESIAN_POINT('Ctrl Pts',(-15.3210406145546,-37.562397408596,18.));
#22813=CARTESIAN_POINT('Ctrl Pts',(-15.3208746890781,-37.6615277218027,
0.));
#22814=CARTESIAN_POINT('Ctrl Pts',(-15.3208746890781,-37.6615277218027,
18.));
#22815=CARTESIAN_POINT('Ctrl Pts',(-15.320070396385,-37.7607947318286,0.));
#22816=CARTESIAN_POINT('Ctrl Pts',(-15.320070396385,-37.7607947318286,18.));
#22817=CARTESIAN_POINT('Ctrl Pts',(-15.3186394335023,-37.8601926265378,
0.));
#22818=CARTESIAN_POINT('Ctrl Pts',(-15.3186394335023,-37.8601926265378,
18.));
#22819=CARTESIAN_POINT('Ctrl Pts',(-15.3165911656268,-37.959716421934,0.));
#22820=CARTESIAN_POINT('Ctrl Pts',(-15.3165911656268,-37.959716421934,18.));
#22821=CARTESIAN_POINT('Ctrl Pts',(-15.3139321941687,-38.0593621055415,
0.));
#22822=CARTESIAN_POINT('Ctrl Pts',(-15.3139321941687,-38.0593621055415,
18.));
#22823=CARTESIAN_POINT('Ctrl Pts',(-15.310667421514,-38.1591262705847,0.));
#22824=CARTESIAN_POINT('Ctrl Pts',(-15.310667421514,-38.1591262705847,18.));
#22825=CARTESIAN_POINT('Ctrl Pts',(-15.3068007250314,-38.2590058835965,
0.));
#22826=CARTESIAN_POINT('Ctrl Pts',(-15.3068007250314,-38.2590058835965,
18.));
#22827=CARTESIAN_POINT('Ctrl Pts',(-15.3023357307483,-38.3589980188324,
0.));
#22828=CARTESIAN_POINT('Ctrl Pts',(-15.3023357307483,-38.3589980188324,
18.));
#22829=CARTESIAN_POINT('Ctrl Pts',(-15.297276703747,-38.4590995527814,0.));
#22830=CARTESIAN_POINT('Ctrl Pts',(-15.297276703747,-38.4590995527814,18.));
#22831=CARTESIAN_POINT('Ctrl Pts',(-15.2916287700102,-38.5593070891769,
0.));
#22832=CARTESIAN_POINT('Ctrl Pts',(-15.2916287700102,-38.5593070891769,
18.));
#22833=CARTESIAN_POINT('Ctrl Pts',(-15.2853974668211,-38.659617115053,0.));
#22834=CARTESIAN_POINT('Ctrl Pts',(-15.2853974668211,-38.659617115053,18.));
#22835=CARTESIAN_POINT('Ctrl Pts',(-15.2785884727112,-38.7600260961351,
0.));
#22836=CARTESIAN_POINT('Ctrl Pts',(-15.2785884727112,-38.7600260961351,
18.));
#22837=CARTESIAN_POINT('Ctrl Pts',(-15.2712072937639,-38.860530586589,0.));
#22838=CARTESIAN_POINT('Ctrl Pts',(-15.2712072937639,-38.860530586589,18.));
#22839=CARTESIAN_POINT('Ctrl Pts',(-15.2632589109473,-38.9611273555758,
0.));
#22840=CARTESIAN_POINT('Ctrl Pts',(-15.2632589109473,-38.9611273555758,
18.));
#22841=CARTESIAN_POINT('Ctrl Pts',(-15.2547476855825,-39.061813415425,0.));
#22842=CARTESIAN_POINT('Ctrl Pts',(-15.2547476855825,-39.061813415425,18.));
#22843=CARTESIAN_POINT('Ctrl Pts',(-15.2456775636447,-39.1625859371304,
0.));
#22844=CARTESIAN_POINT('Ctrl Pts',(-15.2456775636447,-39.1625859371304,
18.));
#22845=CARTESIAN_POINT('Ctrl Pts',(-15.2360522089072,-39.2634421927888,
0.));
#22846=CARTESIAN_POINT('Ctrl Pts',(-15.2360522089072,-39.2634421927888,
18.));
#22847=CARTESIAN_POINT('Ctrl Pts',(-15.225875156307,-39.3643794927167,0.));
#22848=CARTESIAN_POINT('Ctrl Pts',(-15.225875156307,-39.3643794927167,18.));
#22849=CARTESIAN_POINT('Ctrl Pts',(-15.2151499908149,-39.4653951093947,
0.));
#22850=CARTESIAN_POINT('Ctrl Pts',(-15.2151499908149,-39.4653951093947,
18.));
#22851=CARTESIAN_POINT('Ctrl Pts',(-15.2038804098649,-39.5664862602472,
0.));
#22852=CARTESIAN_POINT('Ctrl Pts',(-15.2038804098649,-39.5664862602472,
18.));
#22853=CARTESIAN_POINT('Ctrl Pts',(-15.1920701163804,-39.6676501731673,
0.));
#22854=CARTESIAN_POINT('Ctrl Pts',(-15.1920701163804,-39.6676501731673,
18.));
#22855=CARTESIAN_POINT('Ctrl Pts',(-15.1797227547562,-39.7688841338802,
0.));
#22856=CARTESIAN_POINT('Ctrl Pts',(-15.1797227547562,-39.7688841338802,
18.));
#22857=CARTESIAN_POINT('Ctrl Pts',(-15.1668418393198,-39.8701855339908,
0.));
#22858=CARTESIAN_POINT('Ctrl Pts',(-15.1668418393198,-39.8701855339908,
18.));
#22859=CARTESIAN_POINT('Ctrl Pts',(-15.1534306754871,-39.9715519332134,
0.));
#22860=CARTESIAN_POINT('Ctrl Pts',(-15.1534306754871,-39.9715519332134,
18.));
#22861=CARTESIAN_POINT('Ctrl Pts',(-15.1394923361537,-40.0729810652204,
0.));
#22862=CARTESIAN_POINT('Ctrl Pts',(-15.1394923361537,-40.0729810652204,
18.));
#22863=CARTESIAN_POINT('Ctrl Pts',(-15.1250297462408,-40.1744707357902,
0.));
#22864=CARTESIAN_POINT('Ctrl Pts',(-15.1250297462408,-40.1744707357902,
18.));
#22865=CARTESIAN_POINT('Ctrl Pts',(-15.1100457495259,-40.2760187401821,
0.));
#22866=CARTESIAN_POINT('Ctrl Pts',(-15.1100457495259,-40.2760187401821,
18.));
#22867=CARTESIAN_POINT('Ctrl Pts',(-15.0945431800724,-40.3776227809037,
0.));
#22868=CARTESIAN_POINT('Ctrl Pts',(-15.0945431800724,-40.3776227809037,
18.));
#22869=CARTESIAN_POINT('Ctrl Pts',(-15.0785249502524,-40.4792803645352,
0.));
#22870=CARTESIAN_POINT('Ctrl Pts',(-15.0785249502524,-40.4792803645352,
18.));
#22871=CARTESIAN_POINT('Ctrl Pts',(-15.0619940893017,-40.58098877043,0.));
#22872=CARTESIAN_POINT('Ctrl Pts',(-15.0619940893017,-40.58098877043,18.));
#22873=CARTESIAN_POINT('Ctrl Pts',(-15.0449536183143,-40.6827452453667,
0.));
#22874=CARTESIAN_POINT('Ctrl Pts',(-15.0449536183143,-40.6827452453667,
18.));
#22875=CARTESIAN_POINT('Ctrl Pts',(-15.0274064563211,-40.7845471608654,
0.));
#22876=CARTESIAN_POINT('Ctrl Pts',(-15.0274064563211,-40.7845471608654,
18.));
#22877=CARTESIAN_POINT('Ctrl Pts',(-15.0093553188655,-40.8863921801,0.));
#22878=CARTESIAN_POINT('Ctrl Pts',(-15.0093553188655,-40.8863921801,18.));
#22879=CARTESIAN_POINT('Ctrl Pts',(-14.9908026205824,-40.9882784321884,
0.));
#22880=CARTESIAN_POINT('Ctrl Pts',(-14.9908026205824,-40.9882784321884,
18.));
#22881=CARTESIAN_POINT('Ctrl Pts',(-14.9717503874227,-41.0902046498729,
0.));
#22882=CARTESIAN_POINT('Ctrl Pts',(-14.9717503874227,-41.0902046498729,
18.));
#22883=CARTESIAN_POINT('Ctrl Pts',(-14.9522002356298,-41.1921700381957,
0.));
#22884=CARTESIAN_POINT('Ctrl Pts',(-14.9522002356298,-41.1921700381957,
18.));
#22885=CARTESIAN_POINT('Ctrl Pts',(-14.936162723752,-41.2737733455422,0.));
#22886=CARTESIAN_POINT('Ctrl Pts',(-14.936162723752,-41.2737733455422,18.));
#22887=CARTESIAN_POINT('Ctrl Pts',(-14.9239113834707,-41.3349931861715,
0.));
#22888=CARTESIAN_POINT('Ctrl Pts',(-14.9239113834707,-41.3349931861715,
18.));
#22889=CARTESIAN_POINT('Ctrl Pts',(-14.9156446533966,-41.3758141263348,
0.));
#22890=CARTESIAN_POINT('Ctrl Pts',(-14.9156446533966,-41.3758141263348,
18.));
#22891=CARTESIAN_POINT('Ctrl Pts',(-14.911486495888,-41.396226524684,0.));
#22892=CARTESIAN_POINT('Ctrl Pts',(-14.911486495888,-41.396226524684,18.));
#22893=CARTESIAN_POINT('Ctrl Pts',(-14.9001523628048,-34.5082745737944,
0.));
#22894=CARTESIAN_POINT('Ctrl Pts',(-14.9076710061311,-34.525687510388,0.));
#22895=CARTESIAN_POINT('Ctrl Pts',(-14.9222326355678,-34.5606858566713,
0.));
#22896=CARTESIAN_POINT('Ctrl Pts',(-14.9426481276593,-34.6137007885254,
0.));
#22897=CARTESIAN_POINT('Ctrl Pts',(-14.9671565602316,-34.6853717911268,
0.));
#22898=CARTESIAN_POINT('Ctrl Pts',(-14.9940927023322,-34.7763085406486,
0.));
#22899=CARTESIAN_POINT('Ctrl Pts',(-15.0183713484962,-34.8682205930809,
0.));
#22900=CARTESIAN_POINT('Ctrl Pts',(-15.041018569143,-34.9607388363587,0.));
#22901=CARTESIAN_POINT('Ctrl Pts',(-15.0627878528202,-35.0535882932913,
0.));
#22902=CARTESIAN_POINT('Ctrl Pts',(-15.08395927165,-35.1466591020976,0.));
#22903=CARTESIAN_POINT('Ctrl Pts',(-15.104500806927,-35.2399506932815,0.));
#22904=CARTESIAN_POINT('Ctrl Pts',(-15.1241934020682,-35.3335286891314,
0.));
#22905=CARTESIAN_POINT('Ctrl Pts',(-15.1427632633831,-35.4274792115856,
0.));
#22906=CARTESIAN_POINT('Ctrl Pts',(-15.1600260710384,-35.5218591529745,
0.));
#22907=CARTESIAN_POINT('Ctrl Pts',(-15.1759785763051,-35.6166644736253,
0.));
#22908=CARTESIAN_POINT('Ctrl Pts',(-15.1907243629659,-35.7118553943773,
0.));
#22909=CARTESIAN_POINT('Ctrl Pts',(-15.2044274601769,-35.8073720252878,
0.));
#22910=CARTESIAN_POINT('Ctrl Pts',(-15.2172585668056,-35.9031525499277,
0.));
#22911=CARTESIAN_POINT('Ctrl Pts',(-15.2293360946131,-35.9991531408727,
0.));
#22912=CARTESIAN_POINT('Ctrl Pts',(-15.240697754828,-36.095357546697,0.));
#22913=CARTESIAN_POINT('Ctrl Pts',(-15.2513334565427,-36.1917659216814,
0.));
#22914=CARTESIAN_POINT('Ctrl Pts',(-15.2612053303774,-36.2883880151607,
0.));
#22915=CARTESIAN_POINT('Ctrl Pts',(-15.2702711460937,-36.3852352131887,
0.));
#22916=CARTESIAN_POINT('Ctrl Pts',(-15.2785104654792,-36.4823116513289,
0.));
#22917=CARTESIAN_POINT('Ctrl Pts',(-15.2859343913094,-36.5796108931244,
0.));
#22918=CARTESIAN_POINT('Ctrl Pts',(-15.2925717100767,-36.6771206167755,
0.));
#22919=CARTESIAN_POINT('Ctrl Pts',(-15.2984606286738,-36.7748254044502,
0.));
#22920=CARTESIAN_POINT('Ctrl Pts',(-15.3036390436952,-36.8727100302512,
0.));
#22921=CARTESIAN_POINT('Ctrl Pts',(-15.3081335446406,-36.970763176802,0.));
#22922=CARTESIAN_POINT('Ctrl Pts',(-15.3119562971444,-37.0689784837457,
0.));
#22923=CARTESIAN_POINT('Ctrl Pts',(-15.3151109648809,-37.1673525354641,
0.));
#22924=CARTESIAN_POINT('Ctrl Pts',(-15.3175963510698,-37.2658836214694,
0.));
#22925=CARTESIAN_POINT('Ctrl Pts',(-15.3194106233802,-37.3645702997848,
0.));
#22926=CARTESIAN_POINT('Ctrl Pts',(-15.3205561366169,-37.4634097578665,
0.));
#22927=CARTESIAN_POINT('Ctrl Pts',(-15.3210406145546,-37.562397408596,0.));
#22928=CARTESIAN_POINT('Ctrl Pts',(-15.3208746890781,-37.6615277218027,
0.));
#22929=CARTESIAN_POINT('Ctrl Pts',(-15.320070396385,-37.7607947318286,0.));
#22930=CARTESIAN_POINT('Ctrl Pts',(-15.3186394335023,-37.8601926265378,
0.));
#22931=CARTESIAN_POINT('Ctrl Pts',(-15.3165911656268,-37.959716421934,0.));
#22932=CARTESIAN_POINT('Ctrl Pts',(-15.3139321941687,-38.0593621055415,
0.));
#22933=CARTESIAN_POINT('Ctrl Pts',(-15.310667421514,-38.1591262705847,0.));
#22934=CARTESIAN_POINT('Ctrl Pts',(-15.3068007250314,-38.2590058835965,
0.));
#22935=CARTESIAN_POINT('Ctrl Pts',(-15.3023357307483,-38.3589980188324,
0.));
#22936=CARTESIAN_POINT('Ctrl Pts',(-15.297276703747,-38.4590995527814,0.));
#22937=CARTESIAN_POINT('Ctrl Pts',(-15.2916287700102,-38.5593070891769,
0.));
#22938=CARTESIAN_POINT('Ctrl Pts',(-15.2853974668211,-38.659617115053,0.));
#22939=CARTESIAN_POINT('Ctrl Pts',(-15.2785884727112,-38.7600260961351,
0.));
#22940=CARTESIAN_POINT('Ctrl Pts',(-15.2712072937639,-38.860530586589,0.));
#22941=CARTESIAN_POINT('Ctrl Pts',(-15.2632589109473,-38.9611273555758,
0.));
#22942=CARTESIAN_POINT('Ctrl Pts',(-15.2547476855825,-39.061813415425,0.));
#22943=CARTESIAN_POINT('Ctrl Pts',(-15.2456775636447,-39.1625859371304,
0.));
#22944=CARTESIAN_POINT('Ctrl Pts',(-15.2360522089072,-39.2634421927888,
0.));
#22945=CARTESIAN_POINT('Ctrl Pts',(-15.225875156307,-39.3643794927167,0.));
#22946=CARTESIAN_POINT('Ctrl Pts',(-15.2151499908149,-39.4653951093947,
0.));
#22947=CARTESIAN_POINT('Ctrl Pts',(-15.2038804098649,-39.5664862602472,
0.));
#22948=CARTESIAN_POINT('Ctrl Pts',(-15.1920701163804,-39.6676501731673,
0.));
#22949=CARTESIAN_POINT('Ctrl Pts',(-15.1797227547562,-39.7688841338802,
0.));
#22950=CARTESIAN_POINT('Ctrl Pts',(-15.1668418393198,-39.8701855339908,
0.));
#22951=CARTESIAN_POINT('Ctrl Pts',(-15.1534306754871,-39.9715519332134,
0.));
#22952=CARTESIAN_POINT('Ctrl Pts',(-15.1394923361537,-40.0729810652204,
0.));
#22953=CARTESIAN_POINT('Ctrl Pts',(-15.1250297462408,-40.1744707357902,
0.));
#22954=CARTESIAN_POINT('Ctrl Pts',(-15.1100457495259,-40.2760187401821,
0.));
#22955=CARTESIAN_POINT('Ctrl Pts',(-15.0945431800724,-40.3776227809037,
0.));
#22956=CARTESIAN_POINT('Ctrl Pts',(-15.0785249502524,-40.4792803645352,
0.));
#22957=CARTESIAN_POINT('Ctrl Pts',(-15.0619940893017,-40.58098877043,0.));
#22958=CARTESIAN_POINT('Ctrl Pts',(-15.0449536183143,-40.6827452453667,
0.));
#22959=CARTESIAN_POINT('Ctrl Pts',(-15.0274064563211,-40.7845471608654,
0.));
#22960=CARTESIAN_POINT('Ctrl Pts',(-15.0093553188655,-40.8863921801,0.));
#22961=CARTESIAN_POINT('Ctrl Pts',(-14.9908026205824,-40.9882784321884,
0.));
#22962=CARTESIAN_POINT('Ctrl Pts',(-14.9679399407908,-41.1105898934098,
0.));
#22963=CARTESIAN_POINT('Ctrl Pts',(-14.9482653093396,-41.2125650743922,
0.));
#22964=CARTESIAN_POINT('Ctrl Pts',(-14.9321285285561,-41.2941761025922,
0.));
#22965=CARTESIAN_POINT('Ctrl Pts',(-14.919802810928,-41.3554017279611,0.));
#22966=CARTESIAN_POINT('Ctrl Pts',(-14.911486495888,-41.396226524684,0.));
#22967=CARTESIAN_POINT('Ctrl Pts',(-14.9001523628048,-34.5082745737944,
15.));
#22968=CARTESIAN_POINT('Ctrl Pts',(-14.9076710061311,-34.525687510388,15.));
#22969=CARTESIAN_POINT('Ctrl Pts',(-14.9222326355678,-34.5606858566713,
15.));
#22970=CARTESIAN_POINT('Ctrl Pts',(-14.9426481276593,-34.6137007885254,
15.));
#22971=CARTESIAN_POINT('Ctrl Pts',(-14.9671565602316,-34.6853717911268,
15.));
#22972=CARTESIAN_POINT('Ctrl Pts',(-14.9940927023322,-34.7763085406486,
15.));
#22973=CARTESIAN_POINT('Ctrl Pts',(-15.0183713484962,-34.8682205930809,
15.));
#22974=CARTESIAN_POINT('Ctrl Pts',(-15.041018569143,-34.9607388363587,15.));
#22975=CARTESIAN_POINT('Ctrl Pts',(-15.0627878528202,-35.0535882932913,
15.));
#22976=CARTESIAN_POINT('Ctrl Pts',(-15.08395927165,-35.1466591020976,15.));
#22977=CARTESIAN_POINT('Ctrl Pts',(-15.104500806927,-35.2399506932815,15.));
#22978=CARTESIAN_POINT('Ctrl Pts',(-15.1241934020682,-35.3335286891314,
15.));
#22979=CARTESIAN_POINT('Ctrl Pts',(-15.1427632633831,-35.4274792115856,
15.));
#22980=CARTESIAN_POINT('Ctrl Pts',(-15.1600260710384,-35.5218591529745,
15.));
#22981=CARTESIAN_POINT('Ctrl Pts',(-15.1759785763051,-35.6166644736253,
15.));
#22982=CARTESIAN_POINT('Ctrl Pts',(-15.1907243629659,-35.7118553943773,
15.));
#22983=CARTESIAN_POINT('Ctrl Pts',(-15.2044274601769,-35.8073720252878,
15.));
#22984=CARTESIAN_POINT('Ctrl Pts',(-15.2172585668056,-35.9031525499277,
15.));
#22985=CARTESIAN_POINT('Ctrl Pts',(-15.2293360946131,-35.9991531408727,
15.));
#22986=CARTESIAN_POINT('Ctrl Pts',(-15.240697754828,-36.095357546697,15.));
#22987=CARTESIAN_POINT('Ctrl Pts',(-15.2513334565427,-36.1917659216814,
15.));
#22988=CARTESIAN_POINT('Ctrl Pts',(-15.2612053303774,-36.2883880151607,
15.));
#22989=CARTESIAN_POINT('Ctrl Pts',(-15.2702711460937,-36.3852352131887,
15.));
#22990=CARTESIAN_POINT('Ctrl Pts',(-15.2785104654792,-36.4823116513289,
15.));
#22991=CARTESIAN_POINT('Ctrl Pts',(-15.2859343913094,-36.5796108931244,
15.));
#22992=CARTESIAN_POINT('Ctrl Pts',(-15.2925717100767,-36.6771206167755,
15.));
#22993=CARTESIAN_POINT('Ctrl Pts',(-15.2984606286738,-36.7748254044502,
15.));
#22994=CARTESIAN_POINT('Ctrl Pts',(-15.3036390436952,-36.8727100302512,
15.));
#22995=CARTESIAN_POINT('Ctrl Pts',(-15.3081335446406,-36.970763176802,15.));
#22996=CARTESIAN_POINT('Ctrl Pts',(-15.3119562971444,-37.0689784837457,
15.));
#22997=CARTESIAN_POINT('Ctrl Pts',(-15.3151109648809,-37.1673525354641,
15.));
#22998=CARTESIAN_POINT('Ctrl Pts',(-15.3175963510698,-37.2658836214694,
15.));
#22999=CARTESIAN_POINT('Ctrl Pts',(-15.3194106233802,-37.3645702997848,
15.));
#23000=CARTESIAN_POINT('Ctrl Pts',(-15.3205561366169,-37.4634097578665,
15.));
#23001=CARTESIAN_POINT('Ctrl Pts',(-15.3210406145546,-37.562397408596,15.));
#23002=CARTESIAN_POINT('Ctrl Pts',(-15.3208746890781,-37.6615277218027,
15.));
#23003=CARTESIAN_POINT('Ctrl Pts',(-15.320070396385,-37.7607947318286,15.));
#23004=CARTESIAN_POINT('Ctrl Pts',(-15.3186394335023,-37.8601926265378,
15.));
#23005=CARTESIAN_POINT('Ctrl Pts',(-15.3165911656268,-37.959716421934,15.));
#23006=CARTESIAN_POINT('Ctrl Pts',(-15.3139321941687,-38.0593621055415,
15.));
#23007=CARTESIAN_POINT('Ctrl Pts',(-15.310667421514,-38.1591262705847,15.));
#23008=CARTESIAN_POINT('Ctrl Pts',(-15.3068007250314,-38.2590058835965,
15.));
#23009=CARTESIAN_POINT('Ctrl Pts',(-15.3023357307483,-38.3589980188324,
15.));
#23010=CARTESIAN_POINT('Ctrl Pts',(-15.297276703747,-38.4590995527814,15.));
#23011=CARTESIAN_POINT('Ctrl Pts',(-15.2916287700102,-38.5593070891769,
15.));
#23012=CARTESIAN_POINT('Ctrl Pts',(-15.2853974668211,-38.659617115053,15.));
#23013=CARTESIAN_POINT('Ctrl Pts',(-15.2785884727112,-38.7600260961351,
15.));
#23014=CARTESIAN_POINT('Ctrl Pts',(-15.2712072937639,-38.860530586589,15.));
#23015=CARTESIAN_POINT('Ctrl Pts',(-15.2632589109473,-38.9611273555758,
15.));
#23016=CARTESIAN_POINT('Ctrl Pts',(-15.2547476855825,-39.061813415425,15.));
#23017=CARTESIAN_POINT('Ctrl Pts',(-15.2456775636447,-39.1625859371304,
15.));
#23018=CARTESIAN_POINT('Ctrl Pts',(-15.2360522089072,-39.2634421927888,
15.));
#23019=CARTESIAN_POINT('Ctrl Pts',(-15.225875156307,-39.3643794927167,15.));
#23020=CARTESIAN_POINT('Ctrl Pts',(-15.2151499908149,-39.4653951093947,
15.));
#23021=CARTESIAN_POINT('Ctrl Pts',(-15.2038804098649,-39.5664862602472,
15.));
#23022=CARTESIAN_POINT('Ctrl Pts',(-15.1920701163804,-39.6676501731673,
15.));
#23023=CARTESIAN_POINT('Ctrl Pts',(-15.1797227547562,-39.7688841338802,
15.));
#23024=CARTESIAN_POINT('Ctrl Pts',(-15.1668418393198,-39.8701855339908,
15.));
#23025=CARTESIAN_POINT('Ctrl Pts',(-15.1534306754871,-39.9715519332134,
15.));
#23026=CARTESIAN_POINT('Ctrl Pts',(-15.1394923361537,-40.0729810652204,
15.));
#23027=CARTESIAN_POINT('Ctrl Pts',(-15.1250297462408,-40.1744707357902,
15.));
#23028=CARTESIAN_POINT('Ctrl Pts',(-15.1100457495259,-40.2760187401821,
15.));
#23029=CARTESIAN_POINT('Ctrl Pts',(-15.0945431800724,-40.3776227809037,
15.));
#23030=CARTESIAN_POINT('Ctrl Pts',(-15.0785249502524,-40.4792803645352,
15.));
#23031=CARTESIAN_POINT('Ctrl Pts',(-15.0619940893017,-40.58098877043,15.));
#23032=CARTESIAN_POINT('Ctrl Pts',(-15.0449536183143,-40.6827452453667,
15.));
#23033=CARTESIAN_POINT('Ctrl Pts',(-15.0274064563211,-40.7845471608654,
15.));
#23034=CARTESIAN_POINT('Ctrl Pts',(-15.0093553188655,-40.8863921801,15.));
#23035=CARTESIAN_POINT('Ctrl Pts',(-14.9908026205824,-40.9882784321884,
15.));
#23036=CARTESIAN_POINT('Ctrl Pts',(-14.9679399407908,-41.1105898934098,
15.));
#23037=CARTESIAN_POINT('Ctrl Pts',(-14.9482653093396,-41.2125650743922,
15.));
#23038=CARTESIAN_POINT('Ctrl Pts',(-14.9321285285561,-41.2941761025922,
15.));
#23039=CARTESIAN_POINT('Ctrl Pts',(-14.919802810928,-41.3554017279611,15.));
#23040=CARTESIAN_POINT('Ctrl Pts',(-14.911486495888,-41.396226524684,15.));
#23041=CARTESIAN_POINT('Ctrl Pts',(-24.725498909423,-36.3957374383337,0.));
#23042=CARTESIAN_POINT('Ctrl Pts',(-24.725498909423,-36.3957374383337,18.));
#23043=CARTESIAN_POINT('Ctrl Pts',(-24.7065408286023,-36.3871033517098,
0.));
#23044=CARTESIAN_POINT('Ctrl Pts',(-24.7065408286023,-36.3871033517098,
18.));
#23045=CARTESIAN_POINT('Ctrl Pts',(-24.6686569322616,-36.369797330215,0.));
#23046=CARTESIAN_POINT('Ctrl Pts',(-24.6686569322616,-36.369797330215,18.));
#23047=CARTESIAN_POINT('Ctrl Pts',(-24.6119278836614,-36.3437247532368,
0.));
#23048=CARTESIAN_POINT('Ctrl Pts',(-24.6119278836614,-36.3437247532368,
18.));
#23049=CARTESIAN_POINT('Ctrl Pts',(-24.5364828082556,-36.3087341522969,
0.));
#23050=CARTESIAN_POINT('Ctrl Pts',(-24.5364828082556,-36.3087341522969,
18.));
#23051=CARTESIAN_POINT('Ctrl Pts',(-24.4424997853605,-36.2646168058395,
0.));
#23052=CARTESIAN_POINT('Ctrl Pts',(-24.4424997853605,-36.2646168058395,
18.));
#23053=CARTESIAN_POINT('Ctrl Pts',(-24.3488411214068,-36.2201196586696,
0.));
#23054=CARTESIAN_POINT('Ctrl Pts',(-24.3488411214068,-36.2201196586696,
18.));
#23055=CARTESIAN_POINT('Ctrl Pts',(-24.2555084095332,-36.1752418704833,
0.));
#23056=CARTESIAN_POINT('Ctrl Pts',(-24.2555084095332,-36.1752418704833,
18.));
#23057=CARTESIAN_POINT('Ctrl Pts',(-24.1625038657964,-36.1299825471271,
0.));
#23058=CARTESIAN_POINT('Ctrl Pts',(-24.1625038657964,-36.1299825471271,
18.));
#23059=CARTESIAN_POINT('Ctrl Pts',(-24.0698304230588,-36.0843408347974,
0.));
#23060=CARTESIAN_POINT('Ctrl Pts',(-24.0698304230588,-36.0843408347974,
18.));
#23061=CARTESIAN_POINT('Ctrl Pts',(-23.9774915680089,-36.0383159101253,
0.));
#23062=CARTESIAN_POINT('Ctrl Pts',(-23.9774915680089,-36.0383159101253,
18.));
#23063=CARTESIAN_POINT('Ctrl Pts',(-23.8854911428946,-35.9919069565469,
0.));
#23064=CARTESIAN_POINT('Ctrl Pts',(-23.8854911428946,-35.9919069565469,
18.));
#23065=CARTESIAN_POINT('Ctrl Pts',(-23.7938331508737,-35.9451131482488,
0.));
#23066=CARTESIAN_POINT('Ctrl Pts',(-23.7938331508737,-35.9451131482488,
18.));
#23067=CARTESIAN_POINT('Ctrl Pts',(-23.7025215735353,-35.8979336336837,
0.));
#23068=CARTESIAN_POINT('Ctrl Pts',(-23.7025215735353,-35.8979336336837,
18.));
#23069=CARTESIAN_POINT('Ctrl Pts',(-23.611560139948,-35.8503675222885,0.));
#23070=CARTESIAN_POINT('Ctrl Pts',(-23.611560139948,-35.8503675222885,18.));
#23071=CARTESIAN_POINT('Ctrl Pts',(-23.5209523746427,-35.8024138716896,
0.));
#23072=CARTESIAN_POINT('Ctrl Pts',(-23.5209523746427,-35.8024138716896,
18.));
#23073=CARTESIAN_POINT('Ctrl Pts',(-23.4307017328227,-35.7540716771372,
0.));
#23074=CARTESIAN_POINT('Ctrl Pts',(-23.4307017328227,-35.7540716771372,
18.));
#23075=CARTESIAN_POINT('Ctrl Pts',(-23.3408117088762,-35.7053398620512,
0.));
#23076=CARTESIAN_POINT('Ctrl Pts',(-23.3408117088762,-35.7053398620512,
18.));
#23077=CARTESIAN_POINT('Ctrl Pts',(-23.2512859425032,-35.6562172725207,
0.));
#23078=CARTESIAN_POINT('Ctrl Pts',(-23.2512859425032,-35.6562172725207,
18.));
#23079=CARTESIAN_POINT('Ctrl Pts',(-23.1621283508111,-35.6067026687722,
0.));
#23080=CARTESIAN_POINT('Ctrl Pts',(-23.1621283508111,-35.6067026687722,
18.));
#23081=CARTESIAN_POINT('Ctrl Pts',(-23.0733431097058,-35.5567947408311,
0.));
#23082=CARTESIAN_POINT('Ctrl Pts',(-23.0733431097058,-35.5567947408311,
18.));
#23083=CARTESIAN_POINT('Ctrl Pts',(-22.9849345572033,-35.5064921357308,
0.));
#23084=CARTESIAN_POINT('Ctrl Pts',(-22.9849345572033,-35.5064921357308,
18.));
#23085=CARTESIAN_POINT('Ctrl Pts',(-22.8969071125089,-35.4557934871468,
0.));
#23086=CARTESIAN_POINT('Ctrl Pts',(-22.8969071125089,-35.4557934871468,
18.));
#23087=CARTESIAN_POINT('Ctrl Pts',(-22.8092652000706,-35.4046974393492,
0.));
#23088=CARTESIAN_POINT('Ctrl Pts',(-22.8092652000706,-35.4046974393492,
18.));
#23089=CARTESIAN_POINT('Ctrl Pts',(-22.7220131336912,-35.3532026952313,
0.));
#23090=CARTESIAN_POINT('Ctrl Pts',(-22.7220131336912,-35.3532026952313,
18.));
#23091=CARTESIAN_POINT('Ctrl Pts',(-22.635155167154,-35.3013079759252,0.));
#23092=CARTESIAN_POINT('Ctrl Pts',(-22.635155167154,-35.3013079759252,18.));
#23093=CARTESIAN_POINT('Ctrl Pts',(-22.5486956608909,-35.2490119207975,
0.));
#23094=CARTESIAN_POINT('Ctrl Pts',(-22.5486956608909,-35.2490119207975,
18.));
#23095=CARTESIAN_POINT('Ctrl Pts',(-22.4626392230023,-35.1963130003352,
0.));
#23096=CARTESIAN_POINT('Ctrl Pts',(-22.4626392230023,-35.1963130003352,
18.));
#23097=CARTESIAN_POINT('Ctrl Pts',(-22.3769908340843,-35.1432094422642,
0.));
#23098=CARTESIAN_POINT('Ctrl Pts',(-22.3769908340843,-35.1432094422642,
18.));
#23099=CARTESIAN_POINT('Ctrl Pts',(-22.2917560356803,-35.0896991159359,
0.));
#23100=CARTESIAN_POINT('Ctrl Pts',(-22.2917560356803,-35.0896991159359,
18.));
#23101=CARTESIAN_POINT('Ctrl Pts',(-22.2069408519233,-35.0357795922459,
0.));
#23102=CARTESIAN_POINT('Ctrl Pts',(-22.2069408519233,-35.0357795922459,
18.));
#23103=CARTESIAN_POINT('Ctrl Pts',(-22.1225514798584,-34.9814483545602,
0.));
#23104=CARTESIAN_POINT('Ctrl Pts',(-22.1225514798584,-34.9814483545602,
18.));
#23105=CARTESIAN_POINT('Ctrl Pts',(-22.0385940162683,-34.9267029879922,
0.));
#23106=CARTESIAN_POINT('Ctrl Pts',(-22.0385940162683,-34.9267029879922,
18.));
#23107=CARTESIAN_POINT('Ctrl Pts',(-21.9550742217675,-34.8715413418101,
0.));
#23108=CARTESIAN_POINT('Ctrl Pts',(-21.9550742217675,-34.8715413418101,
18.));
#23109=CARTESIAN_POINT('Ctrl Pts',(-21.8719971302817,-34.8159618014436,
0.));
#23110=CARTESIAN_POINT('Ctrl Pts',(-21.8719971302817,-34.8159618014436,
18.));
#23111=CARTESIAN_POINT('Ctrl Pts',(-21.7893672401137,-34.7599631530844,
0.));
#23112=CARTESIAN_POINT('Ctrl Pts',(-21.7893672401137,-34.7599631530844,
18.));
#23113=CARTESIAN_POINT('Ctrl Pts',(-21.7071892844497,-34.7035440429025,
0.));
#23114=CARTESIAN_POINT('Ctrl Pts',(-21.7071892844497,-34.7035440429025,
18.));
#23115=CARTESIAN_POINT('Ctrl Pts',(-21.6254689009796,-34.6467025072367,
0.));
#23116=CARTESIAN_POINT('Ctrl Pts',(-21.6254689009796,-34.6467025072367,
18.));
#23117=CARTESIAN_POINT('Ctrl Pts',(-21.5442132160757,-34.5894355639081,
0.));
#23118=CARTESIAN_POINT('Ctrl Pts',(-21.5442132160757,-34.5894355639081,
18.));
#23119=CARTESIAN_POINT('Ctrl Pts',(-21.4634317666005,-34.5317385658329,
0.));
#23120=CARTESIAN_POINT('Ctrl Pts',(-21.4634317666005,-34.5317385658329,
18.));
#23121=CARTESIAN_POINT('Ctrl Pts',(-21.3831361300104,-34.4736054662052,
0.));
#23122=CARTESIAN_POINT('Ctrl Pts',(-21.3831361300104,-34.4736054662052,
18.));
#23123=CARTESIAN_POINT('Ctrl Pts',(-21.3033382073239,-34.4150300340623,
0.));
#23124=CARTESIAN_POINT('Ctrl Pts',(-21.3033382073239,-34.4150300340623,
18.));
#23125=CARTESIAN_POINT('Ctrl Pts',(-21.2240487218079,-34.3560069185815,
0.));
#23126=CARTESIAN_POINT('Ctrl Pts',(-21.2240487218079,-34.3560069185815,
18.));
#23127=CARTESIAN_POINT('Ctrl Pts',(-21.1452759244399,-34.2965325673384,
0.));
#23128=CARTESIAN_POINT('Ctrl Pts',(-21.1452759244399,-34.2965325673384,
18.));
#23129=CARTESIAN_POINT('Ctrl Pts',(-21.0670234747355,-34.2366067284279,
0.));
#23130=CARTESIAN_POINT('Ctrl Pts',(-21.0670234747355,-34.2366067284279,
18.));
#23131=CARTESIAN_POINT('Ctrl Pts',(-20.9892914622612,-34.176231731809,0.));
#23132=CARTESIAN_POINT('Ctrl Pts',(-20.9892914622612,-34.176231731809,18.));
#23133=CARTESIAN_POINT('Ctrl Pts',(-20.9120805673809,-34.1154095510973,
0.));
#23134=CARTESIAN_POINT('Ctrl Pts',(-20.9120805673809,-34.1154095510973,
18.));
#23135=CARTESIAN_POINT('Ctrl Pts',(-20.8353957068415,-34.0541392299678,
0.));
#23136=CARTESIAN_POINT('Ctrl Pts',(-20.8353957068415,-34.0541392299678,
18.));
#23137=CARTESIAN_POINT('Ctrl Pts',(-20.7592491770603,-33.9924146647395,
0.));
#23138=CARTESIAN_POINT('Ctrl Pts',(-20.7592491770603,-33.9924146647395,
18.));
#23139=CARTESIAN_POINT('Ctrl Pts',(-20.683665762903,-33.9302209962425,0.));
#23140=CARTESIAN_POINT('Ctrl Pts',(-20.683665762903,-33.9302209962425,18.));
#23141=CARTESIAN_POINT('Ctrl Pts',(-20.6086800574386,-33.8675365150454,
0.));
#23142=CARTESIAN_POINT('Ctrl Pts',(-20.6086800574386,-33.8675365150454,
18.));
#23143=CARTESIAN_POINT('Ctrl Pts',(-20.5343269914034,-33.8043393734971,
0.));
#23144=CARTESIAN_POINT('Ctrl Pts',(-20.5343269914034,-33.8043393734971,
18.));
#23145=CARTESIAN_POINT('Ctrl Pts',(-20.4606334536183,-33.7406135254082,
0.));
#23146=CARTESIAN_POINT('Ctrl Pts',(-20.4606334536183,-33.7406135254082,
18.));
#23147=CARTESIAN_POINT('Ctrl Pts',(-20.3876111773341,-33.6763537716992,
0.));
#23148=CARTESIAN_POINT('Ctrl Pts',(-20.3876111773341,-33.6763537716992,
18.));
#23149=CARTESIAN_POINT('Ctrl Pts',(-20.3152448035298,-33.6115742164079,
0.));
#23150=CARTESIAN_POINT('Ctrl Pts',(-20.3152448035298,-33.6115742164079,
18.));
#23151=CARTESIAN_POINT('Ctrl Pts',(-20.243500298383,-33.5463023319603,0.));
#23152=CARTESIAN_POINT('Ctrl Pts',(-20.243500298383,-33.5463023319603,18.));
#23153=CARTESIAN_POINT('Ctrl Pts',(-20.1723475154533,-33.480563024813,0.));
#23154=CARTESIAN_POINT('Ctrl Pts',(-20.1723475154533,-33.480563024813,18.));
#23155=CARTESIAN_POINT('Ctrl Pts',(-20.1017803986381,-33.4143643679979,
0.));
#23156=CARTESIAN_POINT('Ctrl Pts',(-20.1017803986381,-33.4143643679979,
18.));
#23157=CARTESIAN_POINT('Ctrl Pts',(-20.0318342617213,-33.3476854048385,
0.));
#23158=CARTESIAN_POINT('Ctrl Pts',(-20.0318342617213,-33.3476854048385,
18.));
#23159=CARTESIAN_POINT('Ctrl Pts',(-19.9626141625205,-33.2804560993213,
0.));
#23160=CARTESIAN_POINT('Ctrl Pts',(-19.9626141625205,-33.2804560993213,
18.));
#23161=CARTESIAN_POINT('Ctrl Pts',(-19.8942704458546,-33.2125746879471,
0.));
#23162=CARTESIAN_POINT('Ctrl Pts',(-19.8942704458546,-33.2125746879471,
18.));
#23163=CARTESIAN_POINT('Ctrl Pts',(-19.8269479776239,-33.1439436707661,
0.));
#23164=CARTESIAN_POINT('Ctrl Pts',(-19.8269479776239,-33.1439436707661,
18.));
#23165=CARTESIAN_POINT('Ctrl Pts',(-19.7607398248651,-33.0745026283418,
0.));
#23166=CARTESIAN_POINT('Ctrl Pts',(-19.7607398248651,-33.0745026283418,
18.));
#23167=CARTESIAN_POINT('Ctrl Pts',(-19.6956473461873,-33.004256563411,0.));
#23168=CARTESIAN_POINT('Ctrl Pts',(-19.6956473461873,-33.004256563411,18.));
#23169=CARTESIAN_POINT('Ctrl Pts',(-19.6315161742485,-32.9333211533788,
0.));
#23170=CARTESIAN_POINT('Ctrl Pts',(-19.6315161742485,-32.9333211533788,
18.));
#23171=CARTESIAN_POINT('Ctrl Pts',(-19.5681157030437,-32.8618672807884,
0.));
#23172=CARTESIAN_POINT('Ctrl Pts',(-19.5681157030437,-32.8618672807884,
18.));
#23173=CARTESIAN_POINT('Ctrl Pts',(-19.5052640847974,-32.7900335943248,
0.));
#23174=CARTESIAN_POINT('Ctrl Pts',(-19.5052640847974,-32.7900335943248,
18.));
#23175=CARTESIAN_POINT('Ctrl Pts',(-19.4429429601189,-32.7178463324062,
0.));
#23176=CARTESIAN_POINT('Ctrl Pts',(-19.4429429601189,-32.7178463324062,
18.));
#23177=CARTESIAN_POINT('Ctrl Pts',(-19.381405831319,-32.6451434870609,0.));
#23178=CARTESIAN_POINT('Ctrl Pts',(-19.381405831319,-32.6451434870609,18.));
#23179=CARTESIAN_POINT('Ctrl Pts',(-19.3213180490743,-32.5714771007861,
0.));
#23180=CARTESIAN_POINT('Ctrl Pts',(-19.3213180490743,-32.5714771007861,
18.));
#23181=CARTESIAN_POINT('Ctrl Pts',(-19.2635813403783,-32.4962340238036,
0.));
#23182=CARTESIAN_POINT('Ctrl Pts',(-19.2635813403783,-32.4962340238036,
18.));
#23183=CARTESIAN_POINT('Ctrl Pts',(-19.2200039764927,-32.4342791270009,
0.));
#23184=CARTESIAN_POINT('Ctrl Pts',(-19.2200039764927,-32.4342791270009,
18.));
#23185=CARTESIAN_POINT('Ctrl Pts',(-19.1891139208368,-32.3866012518553,
0.));
#23186=CARTESIAN_POINT('Ctrl Pts',(-19.1891139208368,-32.3866012518553,
18.));
#23187=CARTESIAN_POINT('Ctrl Pts',(-19.1693587749508,-32.3542491343753,
0.));
#23188=CARTESIAN_POINT('Ctrl Pts',(-19.1693587749508,-32.3542491343753,
18.));
#23189=CARTESIAN_POINT('Ctrl Pts',(-19.1596907609891,-32.3379313568208,
0.));
#23190=CARTESIAN_POINT('Ctrl Pts',(-19.1596907609891,-32.3379313568208,
18.));
#23191=CARTESIAN_POINT('',(-24.7254989094229,-36.3957374383337,0.));
#23192=CARTESIAN_POINT('Ctrl Pts',(-19.1596907609891,-32.3379313568208,
0.));
#23193=CARTESIAN_POINT('Ctrl Pts',(-19.1693587749508,-32.3542491343753,
0.));
#23194=CARTESIAN_POINT('Ctrl Pts',(-19.1891139208368,-32.3866012518553,
0.));
#23195=CARTESIAN_POINT('Ctrl Pts',(-19.2200039764927,-32.4342791270009,
0.));
#23196=CARTESIAN_POINT('Ctrl Pts',(-19.2635813403783,-32.4962340238036,
0.));
#23197=CARTESIAN_POINT('Ctrl Pts',(-19.3213180490743,-32.5714771007861,
0.));
#23198=CARTESIAN_POINT('Ctrl Pts',(-19.381405831319,-32.6451434870609,0.));
#23199=CARTESIAN_POINT('Ctrl Pts',(-19.4429429601189,-32.7178463324062,
0.));
#23200=CARTESIAN_POINT('Ctrl Pts',(-19.5052640847974,-32.7900335943248,
0.));
#23201=CARTESIAN_POINT('Ctrl Pts',(-19.5681157030437,-32.8618672807884,
0.));
#23202=CARTESIAN_POINT('Ctrl Pts',(-19.6315161742485,-32.9333211533788,
0.));
#23203=CARTESIAN_POINT('Ctrl Pts',(-19.6956473461873,-33.004256563411,0.));
#23204=CARTESIAN_POINT('Ctrl Pts',(-19.7607398248651,-33.0745026283418,
0.));
#23205=CARTESIAN_POINT('Ctrl Pts',(-19.8269479776239,-33.1439436707661,
0.));
#23206=CARTESIAN_POINT('Ctrl Pts',(-19.8942704458546,-33.2125746879471,
0.));
#23207=CARTESIAN_POINT('Ctrl Pts',(-19.9626141625205,-33.2804560993213,
0.));
#23208=CARTESIAN_POINT('Ctrl Pts',(-20.0318342617213,-33.3476854048385,
0.));
#23209=CARTESIAN_POINT('Ctrl Pts',(-20.1017803986381,-33.4143643679979,
0.));
#23210=CARTESIAN_POINT('Ctrl Pts',(-20.1723475154533,-33.480563024813,0.));
#23211=CARTESIAN_POINT('Ctrl Pts',(-20.243500298383,-33.5463023319603,0.));
#23212=CARTESIAN_POINT('Ctrl Pts',(-20.3152448035298,-33.6115742164079,
0.));
#23213=CARTESIAN_POINT('Ctrl Pts',(-20.3876111773341,-33.6763537716992,
0.));
#23214=CARTESIAN_POINT('Ctrl Pts',(-20.4606334536183,-33.7406135254082,
0.));
#23215=CARTESIAN_POINT('Ctrl Pts',(-20.5343269914034,-33.8043393734971,
0.));
#23216=CARTESIAN_POINT('Ctrl Pts',(-20.6086800574386,-33.8675365150454,
0.));
#23217=CARTESIAN_POINT('Ctrl Pts',(-20.683665762903,-33.9302209962425,0.));
#23218=CARTESIAN_POINT('Ctrl Pts',(-20.7592491770603,-33.9924146647395,
0.));
#23219=CARTESIAN_POINT('Ctrl Pts',(-20.8353957068415,-34.0541392299678,
0.));
#23220=CARTESIAN_POINT('Ctrl Pts',(-20.9120805673809,-34.1154095510973,
0.));
#23221=CARTESIAN_POINT('Ctrl Pts',(-20.9892914622612,-34.176231731809,0.));
#23222=CARTESIAN_POINT('Ctrl Pts',(-21.0670234747355,-34.2366067284279,
0.));
#23223=CARTESIAN_POINT('Ctrl Pts',(-21.1452759244399,-34.2965325673384,
0.));
#23224=CARTESIAN_POINT('Ctrl Pts',(-21.2240487218079,-34.3560069185815,
0.));
#23225=CARTESIAN_POINT('Ctrl Pts',(-21.3033382073239,-34.4150300340623,
0.));
#23226=CARTESIAN_POINT('Ctrl Pts',(-21.3831361300104,-34.4736054662052,
0.));
#23227=CARTESIAN_POINT('Ctrl Pts',(-21.4634317666005,-34.5317385658329,
0.));
#23228=CARTESIAN_POINT('Ctrl Pts',(-21.5442132160757,-34.5894355639081,
0.));
#23229=CARTESIAN_POINT('Ctrl Pts',(-21.6254689009796,-34.6467025072367,
0.));
#23230=CARTESIAN_POINT('Ctrl Pts',(-21.7071892844497,-34.7035440429025,
0.));
#23231=CARTESIAN_POINT('Ctrl Pts',(-21.7893672401137,-34.7599631530844,
0.));
#23232=CARTESIAN_POINT('Ctrl Pts',(-21.8719971302817,-34.8159618014436,
0.));
#23233=CARTESIAN_POINT('Ctrl Pts',(-21.9550742217675,-34.8715413418101,
0.));
#23234=CARTESIAN_POINT('Ctrl Pts',(-22.0385940162683,-34.9267029879922,
0.));
#23235=CARTESIAN_POINT('Ctrl Pts',(-22.1225514798584,-34.9814483545602,
0.));
#23236=CARTESIAN_POINT('Ctrl Pts',(-22.2069408519233,-35.0357795922459,
0.));
#23237=CARTESIAN_POINT('Ctrl Pts',(-22.2917560356803,-35.0896991159359,
0.));
#23238=CARTESIAN_POINT('Ctrl Pts',(-22.3769908340843,-35.1432094422642,
0.));
#23239=CARTESIAN_POINT('Ctrl Pts',(-22.4626392230023,-35.1963130003352,
0.));
#23240=CARTESIAN_POINT('Ctrl Pts',(-22.5486956608909,-35.2490119207975,
0.));
#23241=CARTESIAN_POINT('Ctrl Pts',(-22.635155167154,-35.3013079759252,0.));
#23242=CARTESIAN_POINT('Ctrl Pts',(-22.7220131336912,-35.3532026952313,
0.));
#23243=CARTESIAN_POINT('Ctrl Pts',(-22.8092652000706,-35.4046974393492,
0.));
#23244=CARTESIAN_POINT('Ctrl Pts',(-22.8969071125089,-35.4557934871468,
0.));
#23245=CARTESIAN_POINT('Ctrl Pts',(-22.9849345572033,-35.5064921357308,
0.));
#23246=CARTESIAN_POINT('Ctrl Pts',(-23.0733431097058,-35.5567947408311,
0.));
#23247=CARTESIAN_POINT('Ctrl Pts',(-23.1621283508111,-35.6067026687722,
0.));
#23248=CARTESIAN_POINT('Ctrl Pts',(-23.2512859425032,-35.6562172725207,
0.));
#23249=CARTESIAN_POINT('Ctrl Pts',(-23.3408117088762,-35.7053398620512,
0.));
#23250=CARTESIAN_POINT('Ctrl Pts',(-23.4307017328227,-35.7540716771372,
0.));
#23251=CARTESIAN_POINT('Ctrl Pts',(-23.5209523746427,-35.8024138716896,
0.));
#23252=CARTESIAN_POINT('Ctrl Pts',(-23.611560139948,-35.8503675222885,0.));
#23253=CARTESIAN_POINT('Ctrl Pts',(-23.7025215735353,-35.8979336336837,
0.));
#23254=CARTESIAN_POINT('Ctrl Pts',(-23.7938331508737,-35.9451131482488,
0.));
#23255=CARTESIAN_POINT('Ctrl Pts',(-23.8854911428946,-35.9919069565469,
0.));
#23256=CARTESIAN_POINT('Ctrl Pts',(-23.9774915680089,-36.0383159101253,
0.));
#23257=CARTESIAN_POINT('Ctrl Pts',(-24.0698304230588,-36.0843408347974,
0.));
#23258=CARTESIAN_POINT('Ctrl Pts',(-24.1625038657964,-36.1299825471271,
0.));
#23259=CARTESIAN_POINT('Ctrl Pts',(-24.2555084095332,-36.1752418704833,
0.));
#23260=CARTESIAN_POINT('Ctrl Pts',(-24.3488411214068,-36.2201196586696,
0.));
#23261=CARTESIAN_POINT('Ctrl Pts',(-24.4612315181512,-36.2735162352735,
0.));
#23262=CARTESIAN_POINT('Ctrl Pts',(-24.5552956307817,-36.3175386315528,
0.));
#23263=CARTESIAN_POINT('Ctrl Pts',(-24.630805301288,-36.3524534604648,0.));
#23264=CARTESIAN_POINT('Ctrl Pts',(-24.6875827477484,-36.3784692650901,
0.));
#23265=CARTESIAN_POINT('Ctrl Pts',(-24.725498909423,-36.3957374383337,0.));
#23266=CARTESIAN_POINT('',(-24.7254989094229,-36.3957374383337,15.));
#23267=CARTESIAN_POINT('Ctrl Pts',(-24.725498909423,-36.3957374383337,15.));
#23268=CARTESIAN_POINT('Ctrl Pts',(-24.7065408286023,-36.3871033517098,
15.));
#23269=CARTESIAN_POINT('Ctrl Pts',(-24.6686569322616,-36.369797330215,15.));
#23270=CARTESIAN_POINT('Ctrl Pts',(-24.6119278836614,-36.3437247532368,
15.));
#23271=CARTESIAN_POINT('Ctrl Pts',(-24.5364828082556,-36.3087341522969,
15.));
#23272=CARTESIAN_POINT('Ctrl Pts',(-24.4424997853605,-36.2646168058395,
15.));
#23273=CARTESIAN_POINT('Ctrl Pts',(-24.3488411214068,-36.2201196586696,
15.));
#23274=CARTESIAN_POINT('Ctrl Pts',(-24.2555084095332,-36.1752418704833,
15.));
#23275=CARTESIAN_POINT('Ctrl Pts',(-24.1625038657964,-36.1299825471271,
15.));
#23276=CARTESIAN_POINT('Ctrl Pts',(-24.0698304230588,-36.0843408347974,
15.));
#23277=CARTESIAN_POINT('Ctrl Pts',(-23.9774915680089,-36.0383159101253,
15.));
#23278=CARTESIAN_POINT('Ctrl Pts',(-23.8854911428946,-35.9919069565469,
15.));
#23279=CARTESIAN_POINT('Ctrl Pts',(-23.7938331508737,-35.9451131482488,
15.));
#23280=CARTESIAN_POINT('Ctrl Pts',(-23.7025215735353,-35.8979336336837,
15.));
#23281=CARTESIAN_POINT('Ctrl Pts',(-23.611560139948,-35.8503675222885,15.));
#23282=CARTESIAN_POINT('Ctrl Pts',(-23.5209523746427,-35.8024138716896,
15.));
#23283=CARTESIAN_POINT('Ctrl Pts',(-23.4307017328227,-35.7540716771372,
15.));
#23284=CARTESIAN_POINT('Ctrl Pts',(-23.3408117088762,-35.7053398620512,
15.));
#23285=CARTESIAN_POINT('Ctrl Pts',(-23.2512859425032,-35.6562172725207,
15.));
#23286=CARTESIAN_POINT('Ctrl Pts',(-23.1621283508111,-35.6067026687722,
15.));
#23287=CARTESIAN_POINT('Ctrl Pts',(-23.0733431097058,-35.5567947408311,
15.));
#23288=CARTESIAN_POINT('Ctrl Pts',(-22.9849345572033,-35.5064921357308,
15.));
#23289=CARTESIAN_POINT('Ctrl Pts',(-22.8969071125089,-35.4557934871468,
15.));
#23290=CARTESIAN_POINT('Ctrl Pts',(-22.8092652000706,-35.4046974393492,
15.));
#23291=CARTESIAN_POINT('Ctrl Pts',(-22.7220131336912,-35.3532026952313,
15.));
#23292=CARTESIAN_POINT('Ctrl Pts',(-22.635155167154,-35.3013079759252,15.));
#23293=CARTESIAN_POINT('Ctrl Pts',(-22.5486956608909,-35.2490119207975,
15.));
#23294=CARTESIAN_POINT('Ctrl Pts',(-22.4626392230023,-35.1963130003352,
15.));
#23295=CARTESIAN_POINT('Ctrl Pts',(-22.3769908340843,-35.1432094422642,
15.));
#23296=CARTESIAN_POINT('Ctrl Pts',(-22.2917560356803,-35.0896991159359,
15.));
#23297=CARTESIAN_POINT('Ctrl Pts',(-22.2069408519233,-35.0357795922459,
15.));
#23298=CARTESIAN_POINT('Ctrl Pts',(-22.1225514798584,-34.9814483545602,
15.));
#23299=CARTESIAN_POINT('Ctrl Pts',(-22.0385940162683,-34.9267029879922,
15.));
#23300=CARTESIAN_POINT('Ctrl Pts',(-21.9550742217675,-34.8715413418101,
15.));
#23301=CARTESIAN_POINT('Ctrl Pts',(-21.8719971302817,-34.8159618014436,
15.));
#23302=CARTESIAN_POINT('Ctrl Pts',(-21.7893672401137,-34.7599631530844,
15.));
#23303=CARTESIAN_POINT('Ctrl Pts',(-21.7071892844497,-34.7035440429025,
15.));
#23304=CARTESIAN_POINT('Ctrl Pts',(-21.6254689009796,-34.6467025072367,
15.));
#23305=CARTESIAN_POINT('Ctrl Pts',(-21.5442132160757,-34.5894355639081,
15.));
#23306=CARTESIAN_POINT('Ctrl Pts',(-21.4634317666005,-34.5317385658329,
15.));
#23307=CARTESIAN_POINT('Ctrl Pts',(-21.3831361300104,-34.4736054662052,
15.));
#23308=CARTESIAN_POINT('Ctrl Pts',(-21.3033382073239,-34.4150300340623,
15.));
#23309=CARTESIAN_POINT('Ctrl Pts',(-21.2240487218079,-34.3560069185815,
15.));
#23310=CARTESIAN_POINT('Ctrl Pts',(-21.1452759244399,-34.2965325673384,
15.));
#23311=CARTESIAN_POINT('Ctrl Pts',(-21.0670234747355,-34.2366067284279,
15.));
#23312=CARTESIAN_POINT('Ctrl Pts',(-20.9892914622612,-34.176231731809,15.));
#23313=CARTESIAN_POINT('Ctrl Pts',(-20.9120805673809,-34.1154095510973,
15.));
#23314=CARTESIAN_POINT('Ctrl Pts',(-20.8353957068415,-34.0541392299678,
15.));
#23315=CARTESIAN_POINT('Ctrl Pts',(-20.7592491770603,-33.9924146647395,
15.));
#23316=CARTESIAN_POINT('Ctrl Pts',(-20.683665762903,-33.9302209962425,15.));
#23317=CARTESIAN_POINT('Ctrl Pts',(-20.6086800574386,-33.8675365150454,
15.));
#23318=CARTESIAN_POINT('Ctrl Pts',(-20.5343269914034,-33.8043393734971,
15.));
#23319=CARTESIAN_POINT('Ctrl Pts',(-20.4606334536183,-33.7406135254082,
15.));
#23320=CARTESIAN_POINT('Ctrl Pts',(-20.3876111773341,-33.6763537716992,
15.));
#23321=CARTESIAN_POINT('Ctrl Pts',(-20.3152448035298,-33.6115742164079,
15.));
#23322=CARTESIAN_POINT('Ctrl Pts',(-20.243500298383,-33.5463023319603,15.));
#23323=CARTESIAN_POINT('Ctrl Pts',(-20.1723475154533,-33.480563024813,15.));
#23324=CARTESIAN_POINT('Ctrl Pts',(-20.1017803986381,-33.4143643679979,
15.));
#23325=CARTESIAN_POINT('Ctrl Pts',(-20.0318342617213,-33.3476854048385,
15.));
#23326=CARTESIAN_POINT('Ctrl Pts',(-19.9626141625205,-33.2804560993213,
15.));
#23327=CARTESIAN_POINT('Ctrl Pts',(-19.8942704458546,-33.2125746879471,
15.));
#23328=CARTESIAN_POINT('Ctrl Pts',(-19.8269479776239,-33.1439436707661,
15.));
#23329=CARTESIAN_POINT('Ctrl Pts',(-19.7607398248651,-33.0745026283418,
15.));
#23330=CARTESIAN_POINT('Ctrl Pts',(-19.6956473461873,-33.004256563411,15.));
#23331=CARTESIAN_POINT('Ctrl Pts',(-19.6315161742485,-32.9333211533788,
15.));
#23332=CARTESIAN_POINT('Ctrl Pts',(-19.5681157030437,-32.8618672807884,
15.));
#23333=CARTESIAN_POINT('Ctrl Pts',(-19.5052640847974,-32.7900335943248,
15.));
#23334=CARTESIAN_POINT('Ctrl Pts',(-19.4429429601189,-32.7178463324062,
15.));
#23335=CARTESIAN_POINT('Ctrl Pts',(-19.381405831319,-32.6451434870609,15.));
#23336=CARTESIAN_POINT('Ctrl Pts',(-19.3213180490743,-32.5714771007861,
15.));
#23337=CARTESIAN_POINT('Ctrl Pts',(-19.2635813403783,-32.4962340238036,
15.));
#23338=CARTESIAN_POINT('Ctrl Pts',(-19.2200039764927,-32.4342791270009,
15.));
#23339=CARTESIAN_POINT('Ctrl Pts',(-19.1891139208368,-32.3866012518553,
15.));
#23340=CARTESIAN_POINT('Ctrl Pts',(-19.1693587749508,-32.3542491343753,
15.));
#23341=CARTESIAN_POINT('Ctrl Pts',(-19.1596907609891,-32.3379313568208,
15.));
#23342=CARTESIAN_POINT('',(-24.7254989094229,-36.3957374383337,0.));
#23343=CARTESIAN_POINT('Origin',(-6.66146233219319E-12,-9.16871631793044E-12,
0.));
#23344=CARTESIAN_POINT('',(-26.9738038986838,-34.762248247709,0.));
#23345=CARTESIAN_POINT('Origin',(-6.66146233219319E-12,-9.16871631793044E-12,
0.));
#23346=CARTESIAN_POINT('',(-26.9738038986838,-34.762248247709,15.));
#23347=CARTESIAN_POINT('Origin',(-6.66146233219319E-12,-9.16871631793044E-12,
15.));
#23348=CARTESIAN_POINT('',(-26.9738038986838,-34.762248247709,0.));
#23349=CARTESIAN_POINT('Ctrl Pts',(-24.8345302882955,-28.2149191006268,
0.));
#23350=CARTESIAN_POINT('Ctrl Pts',(-24.8345302882955,-28.2149191006268,
18.));
#23351=CARTESIAN_POINT('Ctrl Pts',(-24.8470618363541,-28.2291563988795,
0.));
#23352=CARTESIAN_POINT('Ctrl Pts',(-24.8470618363541,-28.2291563988795,
18.));
#23353=CARTESIAN_POINT('Ctrl Pts',(-24.8717258526943,-28.2579420132101,
0.));
#23354=CARTESIAN_POINT('Ctrl Pts',(-24.8717258526943,-28.2579420132101,
18.));
#23355=CARTESIAN_POINT('Ctrl Pts',(-24.9075246543798,-28.302053475606,0.));
#23356=CARTESIAN_POINT('Ctrl Pts',(-24.9075246543798,-28.302053475606,18.));
#23357=CARTESIAN_POINT('Ctrl Pts',(-24.9529811166897,-28.3626431274892,
0.));
#23358=CARTESIAN_POINT('Ctrl Pts',(-24.9529811166897,-28.3626431274892,
18.));
#23359=CARTESIAN_POINT('Ctrl Pts',(-25.0066999111736,-28.4408053900206,
0.));
#23360=CARTESIAN_POINT('Ctrl Pts',(-25.0066999111736,-28.4408053900206,
18.));
#23361=CARTESIAN_POINT('Ctrl Pts',(-25.0581926620043,-28.5207164321473,
0.));
#23362=CARTESIAN_POINT('Ctrl Pts',(-25.0581926620043,-28.5207164321473,
18.));
#23363=CARTESIAN_POINT('Ctrl Pts',(-25.108321158239,-28.6017081342376,0.));
#23364=CARTESIAN_POINT('Ctrl Pts',(-25.108321158239,-28.6017081342376,18.));
#23365=CARTESIAN_POINT('Ctrl Pts',(-25.1577170374459,-28.6832861366762,
0.));
#23366=CARTESIAN_POINT('Ctrl Pts',(-25.1577170374459,-28.6832861366762,
18.));
#23367=CARTESIAN_POINT('Ctrl Pts',(-25.2066127148845,-28.7652594076549,
0.));
#23368=CARTESIAN_POINT('Ctrl Pts',(-25.2066127148845,-28.7652594076549,
18.));
#23369=CARTESIAN_POINT('Ctrl Pts',(-25.2549775629725,-28.8476372998748,
0.));
#23370=CARTESIAN_POINT('Ctrl Pts',(-25.2549775629725,-28.8476372998748,
18.));
#23371=CARTESIAN_POINT('Ctrl Pts',(-25.3026235249214,-28.9305499160476,
0.));
#23372=CARTESIAN_POINT('Ctrl Pts',(-25.3026235249214,-28.9305499160476,
18.));
#23373=CARTESIAN_POINT('Ctrl Pts',(-25.3493168206005,-29.0141637699076,
0.));
#23374=CARTESIAN_POINT('Ctrl Pts',(-25.3493168206005,-29.0141637699076,
18.));
#23375=CARTESIAN_POINT('Ctrl Pts',(-25.3948997321279,-29.098589927237,0.));
#23376=CARTESIAN_POINT('Ctrl Pts',(-25.3948997321279,-29.098589927237,18.));
#23377=CARTESIAN_POINT('Ctrl Pts',(-25.4393679214513,-29.183825549991,0.));
#23378=CARTESIAN_POINT('Ctrl Pts',(-25.4393679214513,-29.183825549991,18.));
#23379=CARTESIAN_POINT('Ctrl Pts',(-25.4828076101654,-29.2698007967907,
0.));
#23380=CARTESIAN_POINT('Ctrl Pts',(-25.4828076101654,-29.2698007967907,
18.));
#23381=CARTESIAN_POINT('Ctrl Pts',(-25.5253562922582,-29.356408021119,0.));
#23382=CARTESIAN_POINT('Ctrl Pts',(-25.5253562922582,-29.356408021119,18.));
#23383=CARTESIAN_POINT('Ctrl Pts',(-25.5671572096726,-29.443535683207,0.));
#23384=CARTESIAN_POINT('Ctrl Pts',(-25.5671572096726,-29.443535683207,18.));
#23385=CARTESIAN_POINT('Ctrl Pts',(-25.6083094352667,-29.5311055094509,
0.));
#23386=CARTESIAN_POINT('Ctrl Pts',(-25.6083094352667,-29.5311055094509,
18.));
#23387=CARTESIAN_POINT('Ctrl Pts',(-25.6488438125835,-29.6190903904157,
0.));
#23388=CARTESIAN_POINT('Ctrl Pts',(-25.6488438125835,-29.6190903904157,
18.));
#23389=CARTESIAN_POINT('Ctrl Pts',(-25.6887507922748,-29.7074935910931,
0.));
#23390=CARTESIAN_POINT('Ctrl Pts',(-25.6887507922748,-29.7074935910931,
18.));
#23391=CARTESIAN_POINT('Ctrl Pts',(-25.7279973711305,-29.7963360859334,
0.));
#23392=CARTESIAN_POINT('Ctrl Pts',(-25.7279973711305,-29.7963360859334,
18.));
#23393=CARTESIAN_POINT('Ctrl Pts',(-25.7665469042913,-29.8856417535786,
0.));
#23394=CARTESIAN_POINT('Ctrl Pts',(-25.7665469042913,-29.8856417535786,
18.));
#23395=CARTESIAN_POINT('Ctrl Pts',(-25.8043812318215,-29.9754208429384,
0.));
#23396=CARTESIAN_POINT('Ctrl Pts',(-25.8043812318215,-29.9754208429384,
18.));
#23397=CARTESIAN_POINT('Ctrl Pts',(-25.8415089241134,-30.0656638016321,
0.));
#23398=CARTESIAN_POINT('Ctrl Pts',(-25.8415089241134,-30.0656638016321,
18.));
#23399=CARTESIAN_POINT('Ctrl Pts',(-25.8779535511028,-30.1563500154165,
0.));
#23400=CARTESIAN_POINT('Ctrl Pts',(-25.8779535511028,-30.1563500154165,
18.));
#23401=CARTESIAN_POINT('Ctrl Pts',(-25.9137466853317,-30.2474530144827,
0.));
#23402=CARTESIAN_POINT('Ctrl Pts',(-25.9137466853317,-30.2474530144827,
18.));
#23403=CARTESIAN_POINT('Ctrl Pts',(-25.9489196635424,-30.3389466074503,
0.));
#23404=CARTESIAN_POINT('Ctrl Pts',(-25.9489196635424,-30.3389466074503,
18.));
#23405=CARTESIAN_POINT('Ctrl Pts',(-25.9834942765902,-30.4308118142473,
0.));
#23406=CARTESIAN_POINT('Ctrl Pts',(-25.9834942765902,-30.4308118142473,
18.));
#23407=CARTESIAN_POINT('Ctrl Pts',(-26.0174801292225,-30.5230388264271,
0.));
#23408=CARTESIAN_POINT('Ctrl Pts',(-26.0174801292225,-30.5230388264271,
18.));
#23409=CARTESIAN_POINT('Ctrl Pts',(-26.0508796503166,-30.6156232634061,
0.));
#23410=CARTESIAN_POINT('Ctrl Pts',(-26.0508796503166,-30.6156232634061,
18.));
#23411=CARTESIAN_POINT('Ctrl Pts',(-26.0836911730968,-30.7085638682391,
0.));
#23412=CARTESIAN_POINT('Ctrl Pts',(-26.0836911730968,-30.7085638682391,
18.));
#23413=CARTESIAN_POINT('Ctrl Pts',(-26.1159125093178,-30.8018598357461,
0.));
#23414=CARTESIAN_POINT('Ctrl Pts',(-26.1159125093178,-30.8018598357461,
18.));
#23415=CARTESIAN_POINT('Ctrl Pts',(-26.1475450294082,-30.8955077633644,
0.));
#23416=CARTESIAN_POINT('Ctrl Pts',(-26.1475450294082,-30.8955077633644,
18.));
#23417=CARTESIAN_POINT('Ctrl Pts',(-26.1785946616165,-30.9895009017073,
0.));
#23418=CARTESIAN_POINT('Ctrl Pts',(-26.1785946616165,-30.9895009017073,
18.));
#23419=CARTESIAN_POINT('Ctrl Pts',(-26.2090698085494,-31.0838307058369,
0.));
#23420=CARTESIAN_POINT('Ctrl Pts',(-26.2090698085494,-31.0838307058369,
18.));
#23421=CARTESIAN_POINT('Ctrl Pts',(-26.2389800738215,-31.1784877826858,
0.));
#23422=CARTESIAN_POINT('Ctrl Pts',(-26.2389800738215,-31.1784877826858,
18.));
#23423=CARTESIAN_POINT('Ctrl Pts',(-26.2683347859175,-31.2734629900041,
0.));
#23424=CARTESIAN_POINT('Ctrl Pts',(-26.2683347859175,-31.2734629900041,
18.));
#23425=CARTESIAN_POINT('Ctrl Pts',(-26.2971413115295,-31.3687486937246,
0.));
#23426=CARTESIAN_POINT('Ctrl Pts',(-26.2971413115295,-31.3687486937246,
18.));
#23427=CARTESIAN_POINT('Ctrl Pts',(-26.3254046890485,-31.4643390378084,
0.));
#23428=CARTESIAN_POINT('Ctrl Pts',(-26.3254046890485,-31.4643390378084,
18.));
#23429=CARTESIAN_POINT('Ctrl Pts',(-26.353128528169,-31.5602292672984,0.));
#23430=CARTESIAN_POINT('Ctrl Pts',(-26.353128528169,-31.5602292672984,18.));
#23431=CARTESIAN_POINT('Ctrl Pts',(-26.3803155790949,-31.6564152990236,
0.));
#23432=CARTESIAN_POINT('Ctrl Pts',(-26.3803155790949,-31.6564152990236,
18.));
#23433=CARTESIAN_POINT('Ctrl Pts',(-26.4069683862785,-31.7528932299312,
0.));
#23434=CARTESIAN_POINT('Ctrl Pts',(-26.4069683862785,-31.7528932299312,
18.));
#23435=CARTESIAN_POINT('Ctrl Pts',(-26.433090040836,-31.849658771403,0.));
#23436=CARTESIAN_POINT('Ctrl Pts',(-26.433090040836,-31.849658771403,18.));
#23437=CARTESIAN_POINT('Ctrl Pts',(-26.4586843683627,-31.9467071093816,
0.));
#23438=CARTESIAN_POINT('Ctrl Pts',(-26.4586843683627,-31.9467071093816,
18.));
#23439=CARTESIAN_POINT('Ctrl Pts',(-26.4837555495616,-32.0440331917233,
0.));
#23440=CARTESIAN_POINT('Ctrl Pts',(-26.4837555495616,-32.0440331917233,
18.));
#23441=CARTESIAN_POINT('Ctrl Pts',(-26.5083078928862,-32.1416319023705,
0.));
#23442=CARTESIAN_POINT('Ctrl Pts',(-26.5083078928862,-32.1416319023705,
18.));
#23443=CARTESIAN_POINT('Ctrl Pts',(-26.5323455701117,-32.2394982626669,
0.));
#23444=CARTESIAN_POINT('Ctrl Pts',(-26.5323455701117,-32.2394982626669,
18.));
#23445=CARTESIAN_POINT('Ctrl Pts',(-26.5558723200361,-32.3376276606981,
0.));
#23446=CARTESIAN_POINT('Ctrl Pts',(-26.5558723200361,-32.3376276606981,
18.));
#23447=CARTESIAN_POINT('Ctrl Pts',(-26.5788913672813,-32.4360159072985,
0.));
#23448=CARTESIAN_POINT('Ctrl Pts',(-26.5788913672813,-32.4360159072985,
18.));
#23449=CARTESIAN_POINT('Ctrl Pts',(-26.6014055904817,-32.5346590925498,
0.));
#23450=CARTESIAN_POINT('Ctrl Pts',(-26.6014055904817,-32.5346590925498,
18.));
#23451=CARTESIAN_POINT('Ctrl Pts',(-26.6234176311245,-32.6335534898935,
0.));
#23452=CARTESIAN_POINT('Ctrl Pts',(-26.6234176311245,-32.6335534898935,
18.));
#23453=CARTESIAN_POINT('Ctrl Pts',(-26.6449300199764,-32.7326954489334,
0.));
#23454=CARTESIAN_POINT('Ctrl Pts',(-26.6449300199764,-32.7326954489334,
18.));
#23455=CARTESIAN_POINT('Ctrl Pts',(-26.6659453236976,-32.8320812678271,
0.));
#23456=CARTESIAN_POINT('Ctrl Pts',(-26.6659453236976,-32.8320812678271,
18.));
#23457=CARTESIAN_POINT('Ctrl Pts',(-26.6864661988935,-32.9317071576181,
0.));
#23458=CARTESIAN_POINT('Ctrl Pts',(-26.6864661988935,-32.9317071576181,
18.));
#23459=CARTESIAN_POINT('Ctrl Pts',(-26.7064953106254,-33.03156933761,0.));
#23460=CARTESIAN_POINT('Ctrl Pts',(-26.7064953106254,-33.03156933761,18.));
#23461=CARTESIAN_POINT('Ctrl Pts',(-26.7260352861619,-33.131664100194,0.));
#23462=CARTESIAN_POINT('Ctrl Pts',(-26.7260352861619,-33.131664100194,18.));
#23463=CARTESIAN_POINT('Ctrl Pts',(-26.7450886617884,-33.2319878786519,
0.));
#23464=CARTESIAN_POINT('Ctrl Pts',(-26.7450886617884,-33.2319878786519,
18.));
#23465=CARTESIAN_POINT('Ctrl Pts',(-26.7636578270526,-33.3325373307046,
0.));
#23466=CARTESIAN_POINT('Ctrl Pts',(-26.7636578270526,-33.3325373307046,
18.));
#23467=CARTESIAN_POINT('Ctrl Pts',(-26.7817450041181,-33.4333093513694,
0.));
#23468=CARTESIAN_POINT('Ctrl Pts',(-26.7817450041181,-33.4333093513694,
18.));
#23469=CARTESIAN_POINT('Ctrl Pts',(-26.7993522966985,-33.5343009499673,
0.));
#23470=CARTESIAN_POINT('Ctrl Pts',(-26.7993522966985,-33.5343009499673,
18.));
#23471=CARTESIAN_POINT('Ctrl Pts',(-26.8164817280846,-33.6355091508895,
0.));
#23472=CARTESIAN_POINT('Ctrl Pts',(-26.8164817280846,-33.6355091508895,
18.));
#23473=CARTESIAN_POINT('Ctrl Pts',(-26.8331352836667,-33.7369308933173,
0.));
#23474=CARTESIAN_POINT('Ctrl Pts',(-26.8331352836667,-33.7369308933173,
18.));
#23475=CARTESIAN_POINT('Ctrl Pts',(-26.8493149627661,-33.838562905895,0.));
#23476=CARTESIAN_POINT('Ctrl Pts',(-26.8493149627661,-33.838562905895,18.));
#23477=CARTESIAN_POINT('Ctrl Pts',(-26.8650228056313,-33.9404016650487,
0.));
#23478=CARTESIAN_POINT('Ctrl Pts',(-26.8650228056313,-33.9404016650487,
18.));
#23479=CARTESIAN_POINT('Ctrl Pts',(-26.880260834701,-34.0424436187397,0.));
#23480=CARTESIAN_POINT('Ctrl Pts',(-26.880260834701,-34.0424436187397,18.));
#23481=CARTESIAN_POINT('Ctrl Pts',(-26.895031013894,-34.1446853651051,0.));
#23482=CARTESIAN_POINT('Ctrl Pts',(-26.895031013894,-34.1446853651051,18.));
#23483=CARTESIAN_POINT('Ctrl Pts',(-26.9093352037262,-34.2471238425419,
0.));
#23484=CARTESIAN_POINT('Ctrl Pts',(-26.9093352037262,-34.2471238425419,
18.));
#23485=CARTESIAN_POINT('Ctrl Pts',(-26.9231751225177,-34.3497565255724,
0.));
#23486=CARTESIAN_POINT('Ctrl Pts',(-26.9231751225177,-34.3497565255724,
18.));
#23487=CARTESIAN_POINT('Ctrl Pts',(-26.9365523054581,-34.4525815829097,
0.));
#23488=CARTESIAN_POINT('Ctrl Pts',(-26.9365523054581,-34.4525815829097,
18.));
#23489=CARTESIAN_POINT('Ctrl Pts',(-26.9494680440307,-34.5555977590573,
0.));
#23490=CARTESIAN_POINT('Ctrl Pts',(-26.9494680440307,-34.5555977590573,
18.));
#23491=CARTESIAN_POINT('Ctrl Pts',(-26.9594322726214,-34.6381629799782,
0.));
#23492=CARTESIAN_POINT('Ctrl Pts',(-26.9594322726214,-34.6381629799782,
18.));
#23493=CARTESIAN_POINT('Ctrl Pts',(-26.9666985267609,-34.700172380686,0.));
#23494=CARTESIAN_POINT('Ctrl Pts',(-26.9666985267609,-34.700172380686,18.));
#23495=CARTESIAN_POINT('Ctrl Pts',(-26.9714507634923,-34.7415499619104,
0.));
#23496=CARTESIAN_POINT('Ctrl Pts',(-26.9714507634923,-34.7415499619104,
18.));
#23497=CARTESIAN_POINT('Ctrl Pts',(-26.9738038986838,-34.7622482477091,
0.));
#23498=CARTESIAN_POINT('Ctrl Pts',(-26.9738038986838,-34.7622482477091,
18.));
#23499=CARTESIAN_POINT('Ctrl Pts',(-24.8345302882955,-28.2149191006268,
0.));
#23500=CARTESIAN_POINT('Ctrl Pts',(-24.8470618363541,-28.2291563988795,
0.));
#23501=CARTESIAN_POINT('Ctrl Pts',(-24.8717258526943,-28.2579420132101,
0.));
#23502=CARTESIAN_POINT('Ctrl Pts',(-24.9075246543798,-28.302053475606,0.));
#23503=CARTESIAN_POINT('Ctrl Pts',(-24.9529811166897,-28.3626431274892,
0.));
#23504=CARTESIAN_POINT('Ctrl Pts',(-25.0066999111736,-28.4408053900206,
0.));
#23505=CARTESIAN_POINT('Ctrl Pts',(-25.0581926620043,-28.5207164321473,
0.));
#23506=CARTESIAN_POINT('Ctrl Pts',(-25.108321158239,-28.6017081342376,0.));
#23507=CARTESIAN_POINT('Ctrl Pts',(-25.1577170374459,-28.6832861366762,
0.));
#23508=CARTESIAN_POINT('Ctrl Pts',(-25.2066127148845,-28.7652594076549,
0.));
#23509=CARTESIAN_POINT('Ctrl Pts',(-25.2549775629725,-28.8476372998748,
0.));
#23510=CARTESIAN_POINT('Ctrl Pts',(-25.3026235249214,-28.9305499160476,
0.));
#23511=CARTESIAN_POINT('Ctrl Pts',(-25.3493168206005,-29.0141637699076,
0.));
#23512=CARTESIAN_POINT('Ctrl Pts',(-25.3948997321279,-29.098589927237,0.));
#23513=CARTESIAN_POINT('Ctrl Pts',(-25.4393679214513,-29.183825549991,0.));
#23514=CARTESIAN_POINT('Ctrl Pts',(-25.4828076101654,-29.2698007967907,
0.));
#23515=CARTESIAN_POINT('Ctrl Pts',(-25.5253562922582,-29.356408021119,0.));
#23516=CARTESIAN_POINT('Ctrl Pts',(-25.5671572096726,-29.443535683207,0.));
#23517=CARTESIAN_POINT('Ctrl Pts',(-25.6083094352667,-29.5311055094509,
0.));
#23518=CARTESIAN_POINT('Ctrl Pts',(-25.6488438125835,-29.6190903904157,
0.));
#23519=CARTESIAN_POINT('Ctrl Pts',(-25.6887507922748,-29.7074935910931,
0.));
#23520=CARTESIAN_POINT('Ctrl Pts',(-25.7279973711305,-29.7963360859334,
0.));
#23521=CARTESIAN_POINT('Ctrl Pts',(-25.7665469042913,-29.8856417535786,
0.));
#23522=CARTESIAN_POINT('Ctrl Pts',(-25.8043812318215,-29.9754208429384,
0.));
#23523=CARTESIAN_POINT('Ctrl Pts',(-25.8415089241134,-30.0656638016321,
0.));
#23524=CARTESIAN_POINT('Ctrl Pts',(-25.8779535511028,-30.1563500154165,
0.));
#23525=CARTESIAN_POINT('Ctrl Pts',(-25.9137466853317,-30.2474530144827,
0.));
#23526=CARTESIAN_POINT('Ctrl Pts',(-25.9489196635424,-30.3389466074503,
0.));
#23527=CARTESIAN_POINT('Ctrl Pts',(-25.9834942765902,-30.4308118142473,
0.));
#23528=CARTESIAN_POINT('Ctrl Pts',(-26.0174801292225,-30.5230388264271,
0.));
#23529=CARTESIAN_POINT('Ctrl Pts',(-26.0508796503166,-30.6156232634061,
0.));
#23530=CARTESIAN_POINT('Ctrl Pts',(-26.0836911730968,-30.7085638682391,
0.));
#23531=CARTESIAN_POINT('Ctrl Pts',(-26.1159125093178,-30.8018598357461,
0.));
#23532=CARTESIAN_POINT('Ctrl Pts',(-26.1475450294082,-30.8955077633644,
0.));
#23533=CARTESIAN_POINT('Ctrl Pts',(-26.1785946616165,-30.9895009017073,
0.));
#23534=CARTESIAN_POINT('Ctrl Pts',(-26.2090698085494,-31.0838307058369,
0.));
#23535=CARTESIAN_POINT('Ctrl Pts',(-26.2389800738215,-31.1784877826858,
0.));
#23536=CARTESIAN_POINT('Ctrl Pts',(-26.2683347859175,-31.2734629900041,
0.));
#23537=CARTESIAN_POINT('Ctrl Pts',(-26.2971413115295,-31.3687486937246,
0.));
#23538=CARTESIAN_POINT('Ctrl Pts',(-26.3254046890485,-31.4643390378084,
0.));
#23539=CARTESIAN_POINT('Ctrl Pts',(-26.353128528169,-31.5602292672984,0.));
#23540=CARTESIAN_POINT('Ctrl Pts',(-26.3803155790949,-31.6564152990236,
0.));
#23541=CARTESIAN_POINT('Ctrl Pts',(-26.4069683862785,-31.7528932299312,
0.));
#23542=CARTESIAN_POINT('Ctrl Pts',(-26.433090040836,-31.849658771403,0.));
#23543=CARTESIAN_POINT('Ctrl Pts',(-26.4586843683627,-31.9467071093816,
0.));
#23544=CARTESIAN_POINT('Ctrl Pts',(-26.4837555495616,-32.0440331917233,
0.));
#23545=CARTESIAN_POINT('Ctrl Pts',(-26.5083078928862,-32.1416319023705,
0.));
#23546=CARTESIAN_POINT('Ctrl Pts',(-26.5323455701117,-32.2394982626669,
0.));
#23547=CARTESIAN_POINT('Ctrl Pts',(-26.5558723200361,-32.3376276606981,
0.));
#23548=CARTESIAN_POINT('Ctrl Pts',(-26.5788913672813,-32.4360159072985,
0.));
#23549=CARTESIAN_POINT('Ctrl Pts',(-26.6014055904817,-32.5346590925498,
0.));
#23550=CARTESIAN_POINT('Ctrl Pts',(-26.6234176311245,-32.6335534898935,
0.));
#23551=CARTESIAN_POINT('Ctrl Pts',(-26.6449300199764,-32.7326954489334,
0.));
#23552=CARTESIAN_POINT('Ctrl Pts',(-26.6659453236976,-32.8320812678271,
0.));
#23553=CARTESIAN_POINT('Ctrl Pts',(-26.6864661988935,-32.9317071576181,
0.));
#23554=CARTESIAN_POINT('Ctrl Pts',(-26.7064953106254,-33.03156933761,0.));
#23555=CARTESIAN_POINT('Ctrl Pts',(-26.7260352861619,-33.131664100194,0.));
#23556=CARTESIAN_POINT('Ctrl Pts',(-26.7450886617884,-33.2319878786519,
0.));
#23557=CARTESIAN_POINT('Ctrl Pts',(-26.7636578270526,-33.3325373307046,
0.));
#23558=CARTESIAN_POINT('Ctrl Pts',(-26.7817450041181,-33.4333093513694,
0.));
#23559=CARTESIAN_POINT('Ctrl Pts',(-26.7993522966985,-33.5343009499673,
0.));
#23560=CARTESIAN_POINT('Ctrl Pts',(-26.8164817280846,-33.6355091508895,
0.));
#23561=CARTESIAN_POINT('Ctrl Pts',(-26.8331352836667,-33.7369308933173,
0.));
#23562=CARTESIAN_POINT('Ctrl Pts',(-26.8493149627661,-33.838562905895,0.));
#23563=CARTESIAN_POINT('Ctrl Pts',(-26.8650228056313,-33.9404016650487,
0.));
#23564=CARTESIAN_POINT('Ctrl Pts',(-26.880260834701,-34.0424436187397,0.));
#23565=CARTESIAN_POINT('Ctrl Pts',(-26.895031013894,-34.1446853651051,0.));
#23566=CARTESIAN_POINT('Ctrl Pts',(-26.9093352037262,-34.2471238425419,
0.));
#23567=CARTESIAN_POINT('Ctrl Pts',(-26.9231751225177,-34.3497565255724,
0.));
#23568=CARTESIAN_POINT('Ctrl Pts',(-26.9392277420462,-34.4731465943772,
0.));
#23569=CARTESIAN_POINT('Ctrl Pts',(-26.9520281195268,-34.5762105502273,
0.));
#23570=CARTESIAN_POINT('Ctrl Pts',(-26.9619003236529,-34.6588137898952,
0.));
#23571=CARTESIAN_POINT('Ctrl Pts',(-26.9690976283149,-34.7208516760814,
0.));
#23572=CARTESIAN_POINT('Ctrl Pts',(-26.9738038986838,-34.7622482477091,
0.));
#23573=CARTESIAN_POINT('Ctrl Pts',(-24.8345302882955,-28.2149191006268,
15.));
#23574=CARTESIAN_POINT('Ctrl Pts',(-24.8470618363541,-28.2291563988795,
15.));
#23575=CARTESIAN_POINT('Ctrl Pts',(-24.8717258526943,-28.2579420132101,
15.));
#23576=CARTESIAN_POINT('Ctrl Pts',(-24.9075246543798,-28.302053475606,15.));
#23577=CARTESIAN_POINT('Ctrl Pts',(-24.9529811166897,-28.3626431274892,
15.));
#23578=CARTESIAN_POINT('Ctrl Pts',(-25.0066999111736,-28.4408053900206,
15.));
#23579=CARTESIAN_POINT('Ctrl Pts',(-25.0581926620043,-28.5207164321473,
15.));
#23580=CARTESIAN_POINT('Ctrl Pts',(-25.108321158239,-28.6017081342376,15.));
#23581=CARTESIAN_POINT('Ctrl Pts',(-25.1577170374459,-28.6832861366762,
15.));
#23582=CARTESIAN_POINT('Ctrl Pts',(-25.2066127148845,-28.7652594076549,
15.));
#23583=CARTESIAN_POINT('Ctrl Pts',(-25.2549775629725,-28.8476372998748,
15.));
#23584=CARTESIAN_POINT('Ctrl Pts',(-25.3026235249214,-28.9305499160476,
15.));
#23585=CARTESIAN_POINT('Ctrl Pts',(-25.3493168206005,-29.0141637699076,
15.));
#23586=CARTESIAN_POINT('Ctrl Pts',(-25.3948997321279,-29.098589927237,15.));
#23587=CARTESIAN_POINT('Ctrl Pts',(-25.4393679214513,-29.183825549991,15.));
#23588=CARTESIAN_POINT('Ctrl Pts',(-25.4828076101654,-29.2698007967907,
15.));
#23589=CARTESIAN_POINT('Ctrl Pts',(-25.5253562922582,-29.356408021119,15.));
#23590=CARTESIAN_POINT('Ctrl Pts',(-25.5671572096726,-29.443535683207,15.));
#23591=CARTESIAN_POINT('Ctrl Pts',(-25.6083094352667,-29.5311055094509,
15.));
#23592=CARTESIAN_POINT('Ctrl Pts',(-25.6488438125835,-29.6190903904157,
15.));
#23593=CARTESIAN_POINT('Ctrl Pts',(-25.6887507922748,-29.7074935910931,
15.));
#23594=CARTESIAN_POINT('Ctrl Pts',(-25.7279973711305,-29.7963360859334,
15.));
#23595=CARTESIAN_POINT('Ctrl Pts',(-25.7665469042913,-29.8856417535786,
15.));
#23596=CARTESIAN_POINT('Ctrl Pts',(-25.8043812318215,-29.9754208429384,
15.));
#23597=CARTESIAN_POINT('Ctrl Pts',(-25.8415089241134,-30.0656638016321,
15.));
#23598=CARTESIAN_POINT('Ctrl Pts',(-25.8779535511028,-30.1563500154165,
15.));
#23599=CARTESIAN_POINT('Ctrl Pts',(-25.9137466853317,-30.2474530144827,
15.));
#23600=CARTESIAN_POINT('Ctrl Pts',(-25.9489196635424,-30.3389466074503,
15.));
#23601=CARTESIAN_POINT('Ctrl Pts',(-25.9834942765902,-30.4308118142473,
15.));
#23602=CARTESIAN_POINT('Ctrl Pts',(-26.0174801292225,-30.5230388264271,
15.));
#23603=CARTESIAN_POINT('Ctrl Pts',(-26.0508796503166,-30.6156232634061,
15.));
#23604=CARTESIAN_POINT('Ctrl Pts',(-26.0836911730968,-30.7085638682391,
15.));
#23605=CARTESIAN_POINT('Ctrl Pts',(-26.1159125093178,-30.8018598357461,
15.));
#23606=CARTESIAN_POINT('Ctrl Pts',(-26.1475450294082,-30.8955077633644,
15.));
#23607=CARTESIAN_POINT('Ctrl Pts',(-26.1785946616165,-30.9895009017073,
15.));
#23608=CARTESIAN_POINT('Ctrl Pts',(-26.2090698085494,-31.0838307058369,
15.));
#23609=CARTESIAN_POINT('Ctrl Pts',(-26.2389800738215,-31.1784877826858,
15.));
#23610=CARTESIAN_POINT('Ctrl Pts',(-26.2683347859175,-31.2734629900041,
15.));
#23611=CARTESIAN_POINT('Ctrl Pts',(-26.2971413115295,-31.3687486937246,
15.));
#23612=CARTESIAN_POINT('Ctrl Pts',(-26.3254046890485,-31.4643390378084,
15.));
#23613=CARTESIAN_POINT('Ctrl Pts',(-26.353128528169,-31.5602292672984,15.));
#23614=CARTESIAN_POINT('Ctrl Pts',(-26.3803155790949,-31.6564152990236,
15.));
#23615=CARTESIAN_POINT('Ctrl Pts',(-26.4069683862785,-31.7528932299312,
15.));
#23616=CARTESIAN_POINT('Ctrl Pts',(-26.433090040836,-31.849658771403,15.));
#23617=CARTESIAN_POINT('Ctrl Pts',(-26.4586843683627,-31.9467071093816,
15.));
#23618=CARTESIAN_POINT('Ctrl Pts',(-26.4837555495616,-32.0440331917233,
15.));
#23619=CARTESIAN_POINT('Ctrl Pts',(-26.5083078928862,-32.1416319023705,
15.));
#23620=CARTESIAN_POINT('Ctrl Pts',(-26.5323455701117,-32.2394982626669,
15.));
#23621=CARTESIAN_POINT('Ctrl Pts',(-26.5558723200361,-32.3376276606981,
15.));
#23622=CARTESIAN_POINT('Ctrl Pts',(-26.5788913672813,-32.4360159072985,
15.));
#23623=CARTESIAN_POINT('Ctrl Pts',(-26.6014055904817,-32.5346590925498,
15.));
#23624=CARTESIAN_POINT('Ctrl Pts',(-26.6234176311245,-32.6335534898935,
15.));
#23625=CARTESIAN_POINT('Ctrl Pts',(-26.6449300199764,-32.7326954489334,
15.));
#23626=CARTESIAN_POINT('Ctrl Pts',(-26.6659453236976,-32.8320812678271,
15.));
#23627=CARTESIAN_POINT('Ctrl Pts',(-26.6864661988935,-32.9317071576181,
15.));
#23628=CARTESIAN_POINT('Ctrl Pts',(-26.7064953106254,-33.03156933761,15.));
#23629=CARTESIAN_POINT('Ctrl Pts',(-26.7260352861619,-33.131664100194,15.));
#23630=CARTESIAN_POINT('Ctrl Pts',(-26.7450886617884,-33.2319878786519,
15.));
#23631=CARTESIAN_POINT('Ctrl Pts',(-26.7636578270526,-33.3325373307046,
15.));
#23632=CARTESIAN_POINT('Ctrl Pts',(-26.7817450041181,-33.4333093513694,
15.));
#23633=CARTESIAN_POINT('Ctrl Pts',(-26.7993522966985,-33.5343009499673,
15.));
#23634=CARTESIAN_POINT('Ctrl Pts',(-26.8164817280846,-33.6355091508895,
15.));
#23635=CARTESIAN_POINT('Ctrl Pts',(-26.8331352836667,-33.7369308933173,
15.));
#23636=CARTESIAN_POINT('Ctrl Pts',(-26.8493149627661,-33.838562905895,15.));
#23637=CARTESIAN_POINT('Ctrl Pts',(-26.8650228056313,-33.9404016650487,
15.));
#23638=CARTESIAN_POINT('Ctrl Pts',(-26.880260834701,-34.0424436187397,15.));
#23639=CARTESIAN_POINT('Ctrl Pts',(-26.895031013894,-34.1446853651051,15.));
#23640=CARTESIAN_POINT('Ctrl Pts',(-26.9093352037262,-34.2471238425419,
15.));
#23641=CARTESIAN_POINT('Ctrl Pts',(-26.9231751225177,-34.3497565255724,
15.));
#23642=CARTESIAN_POINT('Ctrl Pts',(-26.9392277420462,-34.4731465943772,
15.));
#23643=CARTESIAN_POINT('Ctrl Pts',(-26.9520281195268,-34.5762105502273,
15.));
#23644=CARTESIAN_POINT('Ctrl Pts',(-26.9619003236529,-34.6588137898952,
15.));
#23645=CARTESIAN_POINT('Ctrl Pts',(-26.9690976283149,-34.7208516760814,
15.));
#23646=CARTESIAN_POINT('Ctrl Pts',(-26.9738038986838,-34.7622482477091,
15.));
#23647=CARTESIAN_POINT('Ctrl Pts',(-34.7622482477091,-26.9738038986838,
0.));
#23648=CARTESIAN_POINT('Ctrl Pts',(-34.7622482477091,-26.9738038986838,
18.));
#23649=CARTESIAN_POINT('Ctrl Pts',(-34.7415499619104,-26.9714507634923,
0.));
#23650=CARTESIAN_POINT('Ctrl Pts',(-34.7415499619104,-26.9714507634923,
18.));
#23651=CARTESIAN_POINT('Ctrl Pts',(-34.700172380686,-26.9666985267608,0.));
#23652=CARTESIAN_POINT('Ctrl Pts',(-34.700172380686,-26.9666985267608,18.));
#23653=CARTESIAN_POINT('Ctrl Pts',(-34.6381629799782,-26.9594322726214,
0.));
#23654=CARTESIAN_POINT('Ctrl Pts',(-34.6381629799782,-26.9594322726214,
18.));
#23655=CARTESIAN_POINT('Ctrl Pts',(-34.5555977590573,-26.9494680440307,
0.));
#23656=CARTESIAN_POINT('Ctrl Pts',(-34.5555977590573,-26.9494680440307,
18.));
#23657=CARTESIAN_POINT('Ctrl Pts',(-34.4525815829097,-26.9365523054581,
0.));
#23658=CARTESIAN_POINT('Ctrl Pts',(-34.4525815829097,-26.9365523054581,
18.));
#23659=CARTESIAN_POINT('Ctrl Pts',(-34.3497565255724,-26.9231751225177,
0.));
#23660=CARTESIAN_POINT('Ctrl Pts',(-34.3497565255724,-26.9231751225177,
18.));
#23661=CARTESIAN_POINT('Ctrl Pts',(-34.2471238425419,-26.9093352037262,
0.));
#23662=CARTESIAN_POINT('Ctrl Pts',(-34.2471238425419,-26.9093352037262,
18.));
#23663=CARTESIAN_POINT('Ctrl Pts',(-34.1446853651051,-26.8950310138939,
0.));
#23664=CARTESIAN_POINT('Ctrl Pts',(-34.1446853651051,-26.8950310138939,
18.));
#23665=CARTESIAN_POINT('Ctrl Pts',(-34.0424436187397,-26.880260834701,0.));
#23666=CARTESIAN_POINT('Ctrl Pts',(-34.0424436187397,-26.880260834701,18.));
#23667=CARTESIAN_POINT('Ctrl Pts',(-33.9404016650487,-26.8650228056313,
0.));
#23668=CARTESIAN_POINT('Ctrl Pts',(-33.9404016650487,-26.8650228056313,
18.));
#23669=CARTESIAN_POINT('Ctrl Pts',(-33.838562905895,-26.8493149627661,0.));
#23670=CARTESIAN_POINT('Ctrl Pts',(-33.838562905895,-26.8493149627661,18.));
#23671=CARTESIAN_POINT('Ctrl Pts',(-33.7369308933173,-26.8331352836666,
0.));
#23672=CARTESIAN_POINT('Ctrl Pts',(-33.7369308933173,-26.8331352836666,
18.));
#23673=CARTESIAN_POINT('Ctrl Pts',(-33.6355091508895,-26.8164817280846,
0.));
#23674=CARTESIAN_POINT('Ctrl Pts',(-33.6355091508895,-26.8164817280846,
18.));
#23675=CARTESIAN_POINT('Ctrl Pts',(-33.5343009499673,-26.7993522966985,
0.));
#23676=CARTESIAN_POINT('Ctrl Pts',(-33.5343009499673,-26.7993522966985,
18.));
#23677=CARTESIAN_POINT('Ctrl Pts',(-33.4333093513694,-26.7817450041181,
0.));
#23678=CARTESIAN_POINT('Ctrl Pts',(-33.4333093513694,-26.7817450041181,
18.));
#23679=CARTESIAN_POINT('Ctrl Pts',(-33.3325373307046,-26.7636578270526,
0.));
#23680=CARTESIAN_POINT('Ctrl Pts',(-33.3325373307046,-26.7636578270526,
18.));
#23681=CARTESIAN_POINT('Ctrl Pts',(-33.2319878786519,-26.7450886617884,
0.));
#23682=CARTESIAN_POINT('Ctrl Pts',(-33.2319878786519,-26.7450886617884,
18.));
#23683=CARTESIAN_POINT('Ctrl Pts',(-33.131664100194,-26.7260352861619,0.));
#23684=CARTESIAN_POINT('Ctrl Pts',(-33.131664100194,-26.7260352861619,18.));
#23685=CARTESIAN_POINT('Ctrl Pts',(-33.03156933761,-26.7064953106254,0.));
#23686=CARTESIAN_POINT('Ctrl Pts',(-33.03156933761,-26.7064953106254,18.));
#23687=CARTESIAN_POINT('Ctrl Pts',(-32.9317071576181,-26.6864661988935,
0.));
#23688=CARTESIAN_POINT('Ctrl Pts',(-32.9317071576181,-26.6864661988935,
18.));
#23689=CARTESIAN_POINT('Ctrl Pts',(-32.8320812678271,-26.6659453236976,
0.));
#23690=CARTESIAN_POINT('Ctrl Pts',(-32.8320812678271,-26.6659453236976,
18.));
#23691=CARTESIAN_POINT('Ctrl Pts',(-32.7326954489334,-26.6449300199763,
0.));
#23692=CARTESIAN_POINT('Ctrl Pts',(-32.7326954489334,-26.6449300199763,
18.));
#23693=CARTESIAN_POINT('Ctrl Pts',(-32.6335534898936,-26.6234176311245,
0.));
#23694=CARTESIAN_POINT('Ctrl Pts',(-32.6335534898936,-26.6234176311245,
18.));
#23695=CARTESIAN_POINT('Ctrl Pts',(-32.5346590925498,-26.6014055904817,
0.));
#23696=CARTESIAN_POINT('Ctrl Pts',(-32.5346590925498,-26.6014055904817,
18.));
#23697=CARTESIAN_POINT('Ctrl Pts',(-32.4360159072985,-26.5788913672813,
0.));
#23698=CARTESIAN_POINT('Ctrl Pts',(-32.4360159072985,-26.5788913672813,
18.));
#23699=CARTESIAN_POINT('Ctrl Pts',(-32.3376276606981,-26.5558723200361,
0.));
#23700=CARTESIAN_POINT('Ctrl Pts',(-32.3376276606981,-26.5558723200361,
18.));
#23701=CARTESIAN_POINT('Ctrl Pts',(-32.2394982626669,-26.5323455701117,
0.));
#23702=CARTESIAN_POINT('Ctrl Pts',(-32.2394982626669,-26.5323455701117,
18.));
#23703=CARTESIAN_POINT('Ctrl Pts',(-32.1416319023705,-26.5083078928862,
0.));
#23704=CARTESIAN_POINT('Ctrl Pts',(-32.1416319023705,-26.5083078928862,
18.));
#23705=CARTESIAN_POINT('Ctrl Pts',(-32.0440331917233,-26.4837555495616,
0.));
#23706=CARTESIAN_POINT('Ctrl Pts',(-32.0440331917233,-26.4837555495616,
18.));
#23707=CARTESIAN_POINT('Ctrl Pts',(-31.9467071093816,-26.4586843683627,
0.));
#23708=CARTESIAN_POINT('Ctrl Pts',(-31.9467071093816,-26.4586843683627,
18.));
#23709=CARTESIAN_POINT('Ctrl Pts',(-31.849658771403,-26.433090040836,0.));
#23710=CARTESIAN_POINT('Ctrl Pts',(-31.849658771403,-26.433090040836,18.));
#23711=CARTESIAN_POINT('Ctrl Pts',(-31.7528932299312,-26.4069683862784,
0.));
#23712=CARTESIAN_POINT('Ctrl Pts',(-31.7528932299312,-26.4069683862784,
18.));
#23713=CARTESIAN_POINT('Ctrl Pts',(-31.6564152990236,-26.3803155790949,
0.));
#23714=CARTESIAN_POINT('Ctrl Pts',(-31.6564152990236,-26.3803155790949,
18.));
#23715=CARTESIAN_POINT('Ctrl Pts',(-31.5602292672984,-26.353128528169,0.));
#23716=CARTESIAN_POINT('Ctrl Pts',(-31.5602292672984,-26.353128528169,18.));
#23717=CARTESIAN_POINT('Ctrl Pts',(-31.4643390378084,-26.3254046890485,
0.));
#23718=CARTESIAN_POINT('Ctrl Pts',(-31.4643390378084,-26.3254046890485,
18.));
#23719=CARTESIAN_POINT('Ctrl Pts',(-31.3687486937246,-26.2971413115295,
0.));
#23720=CARTESIAN_POINT('Ctrl Pts',(-31.3687486937246,-26.2971413115295,
18.));
#23721=CARTESIAN_POINT('Ctrl Pts',(-31.2734629900041,-26.2683347859175,
0.));
#23722=CARTESIAN_POINT('Ctrl Pts',(-31.2734629900041,-26.2683347859175,
18.));
#23723=CARTESIAN_POINT('Ctrl Pts',(-31.1784877826858,-26.2389800738215,
0.));
#23724=CARTESIAN_POINT('Ctrl Pts',(-31.1784877826858,-26.2389800738215,
18.));
#23725=CARTESIAN_POINT('Ctrl Pts',(-31.0838307058369,-26.2090698085494,
0.));
#23726=CARTESIAN_POINT('Ctrl Pts',(-31.0838307058369,-26.2090698085494,
18.));
#23727=CARTESIAN_POINT('Ctrl Pts',(-30.9895009017073,-26.1785946616165,
0.));
#23728=CARTESIAN_POINT('Ctrl Pts',(-30.9895009017073,-26.1785946616165,
18.));
#23729=CARTESIAN_POINT('Ctrl Pts',(-30.8955077633644,-26.1475450294082,
0.));
#23730=CARTESIAN_POINT('Ctrl Pts',(-30.8955077633644,-26.1475450294082,
18.));
#23731=CARTESIAN_POINT('Ctrl Pts',(-30.8018598357461,-26.1159125093178,
0.));
#23732=CARTESIAN_POINT('Ctrl Pts',(-30.8018598357461,-26.1159125093178,
18.));
#23733=CARTESIAN_POINT('Ctrl Pts',(-30.7085638682391,-26.0836911730968,
0.));
#23734=CARTESIAN_POINT('Ctrl Pts',(-30.7085638682391,-26.0836911730968,
18.));
#23735=CARTESIAN_POINT('Ctrl Pts',(-30.6156232634061,-26.0508796503166,
0.));
#23736=CARTESIAN_POINT('Ctrl Pts',(-30.6156232634061,-26.0508796503166,
18.));
#23737=CARTESIAN_POINT('Ctrl Pts',(-30.5230388264271,-26.0174801292225,
0.));
#23738=CARTESIAN_POINT('Ctrl Pts',(-30.5230388264271,-26.0174801292225,
18.));
#23739=CARTESIAN_POINT('Ctrl Pts',(-30.4308118142473,-25.9834942765902,
0.));
#23740=CARTESIAN_POINT('Ctrl Pts',(-30.4308118142473,-25.9834942765902,
18.));
#23741=CARTESIAN_POINT('Ctrl Pts',(-30.3389466074503,-25.9489196635424,
0.));
#23742=CARTESIAN_POINT('Ctrl Pts',(-30.3389466074503,-25.9489196635424,
18.));
#23743=CARTESIAN_POINT('Ctrl Pts',(-30.2474530144827,-25.9137466853317,
0.));
#23744=CARTESIAN_POINT('Ctrl Pts',(-30.2474530144827,-25.9137466853317,
18.));
#23745=CARTESIAN_POINT('Ctrl Pts',(-30.1563500154165,-25.8779535511027,
0.));
#23746=CARTESIAN_POINT('Ctrl Pts',(-30.1563500154165,-25.8779535511027,
18.));
#23747=CARTESIAN_POINT('Ctrl Pts',(-30.0656638016321,-25.8415089241134,
0.));
#23748=CARTESIAN_POINT('Ctrl Pts',(-30.0656638016321,-25.8415089241134,
18.));
#23749=CARTESIAN_POINT('Ctrl Pts',(-29.9754208429384,-25.8043812318214,
0.));
#23750=CARTESIAN_POINT('Ctrl Pts',(-29.9754208429384,-25.8043812318214,
18.));
#23751=CARTESIAN_POINT('Ctrl Pts',(-29.8856417535786,-25.7665469042913,
0.));
#23752=CARTESIAN_POINT('Ctrl Pts',(-29.8856417535786,-25.7665469042913,
18.));
#23753=CARTESIAN_POINT('Ctrl Pts',(-29.7963360859334,-25.7279973711305,
0.));
#23754=CARTESIAN_POINT('Ctrl Pts',(-29.7963360859334,-25.7279973711305,
18.));
#23755=CARTESIAN_POINT('Ctrl Pts',(-29.7074935910931,-25.6887507922748,
0.));
#23756=CARTESIAN_POINT('Ctrl Pts',(-29.7074935910931,-25.6887507922748,
18.));
#23757=CARTESIAN_POINT('Ctrl Pts',(-29.6190903904157,-25.6488438125835,
0.));
#23758=CARTESIAN_POINT('Ctrl Pts',(-29.6190903904157,-25.6488438125835,
18.));
#23759=CARTESIAN_POINT('Ctrl Pts',(-29.5311055094509,-25.6083094352667,
0.));
#23760=CARTESIAN_POINT('Ctrl Pts',(-29.5311055094509,-25.6083094352667,
18.));
#23761=CARTESIAN_POINT('Ctrl Pts',(-29.443535683207,-25.5671572096726,0.));
#23762=CARTESIAN_POINT('Ctrl Pts',(-29.443535683207,-25.5671572096726,18.));
#23763=CARTESIAN_POINT('Ctrl Pts',(-29.356408021119,-25.5253562922582,0.));
#23764=CARTESIAN_POINT('Ctrl Pts',(-29.356408021119,-25.5253562922582,18.));
#23765=CARTESIAN_POINT('Ctrl Pts',(-29.2698007967907,-25.4828076101654,
0.));
#23766=CARTESIAN_POINT('Ctrl Pts',(-29.2698007967907,-25.4828076101654,
18.));
#23767=CARTESIAN_POINT('Ctrl Pts',(-29.183825549991,-25.4393679214513,0.));
#23768=CARTESIAN_POINT('Ctrl Pts',(-29.183825549991,-25.4393679214513,18.));
#23769=CARTESIAN_POINT('Ctrl Pts',(-29.098589927237,-25.3948997321279,0.));
#23770=CARTESIAN_POINT('Ctrl Pts',(-29.098589927237,-25.3948997321279,18.));
#23771=CARTESIAN_POINT('Ctrl Pts',(-29.0141637699076,-25.3493168206005,
0.));
#23772=CARTESIAN_POINT('Ctrl Pts',(-29.0141637699076,-25.3493168206005,
18.));
#23773=CARTESIAN_POINT('Ctrl Pts',(-28.9305499160476,-25.3026235249214,
0.));
#23774=CARTESIAN_POINT('Ctrl Pts',(-28.9305499160476,-25.3026235249214,
18.));
#23775=CARTESIAN_POINT('Ctrl Pts',(-28.8476372998748,-25.2549775629725,
0.));
#23776=CARTESIAN_POINT('Ctrl Pts',(-28.8476372998748,-25.2549775629725,
18.));
#23777=CARTESIAN_POINT('Ctrl Pts',(-28.7652594076549,-25.2066127148845,
0.));
#23778=CARTESIAN_POINT('Ctrl Pts',(-28.7652594076549,-25.2066127148845,
18.));
#23779=CARTESIAN_POINT('Ctrl Pts',(-28.6832861366762,-25.1577170374459,
0.));
#23780=CARTESIAN_POINT('Ctrl Pts',(-28.6832861366762,-25.1577170374459,
18.));
#23781=CARTESIAN_POINT('Ctrl Pts',(-28.6017081342376,-25.108321158239,0.));
#23782=CARTESIAN_POINT('Ctrl Pts',(-28.6017081342376,-25.108321158239,18.));
#23783=CARTESIAN_POINT('Ctrl Pts',(-28.5207164321473,-25.0581926620043,
0.));
#23784=CARTESIAN_POINT('Ctrl Pts',(-28.5207164321473,-25.0581926620043,
18.));
#23785=CARTESIAN_POINT('Ctrl Pts',(-28.4408053900206,-25.0066999111736,
0.));
#23786=CARTESIAN_POINT('Ctrl Pts',(-28.4408053900206,-25.0066999111736,
18.));
#23787=CARTESIAN_POINT('Ctrl Pts',(-28.3626431274892,-24.9529811166897,
0.));
#23788=CARTESIAN_POINT('Ctrl Pts',(-28.3626431274892,-24.9529811166897,
18.));
#23789=CARTESIAN_POINT('Ctrl Pts',(-28.3020534756061,-24.9075246543798,
0.));
#23790=CARTESIAN_POINT('Ctrl Pts',(-28.3020534756061,-24.9075246543798,
18.));
#23791=CARTESIAN_POINT('Ctrl Pts',(-28.2579420132101,-24.8717258526943,
0.));
#23792=CARTESIAN_POINT('Ctrl Pts',(-28.2579420132101,-24.8717258526943,
18.));
#23793=CARTESIAN_POINT('Ctrl Pts',(-28.2291563988796,-24.8470618363541,
0.));
#23794=CARTESIAN_POINT('Ctrl Pts',(-28.2291563988796,-24.8470618363541,
18.));
#23795=CARTESIAN_POINT('Ctrl Pts',(-28.2149191006269,-24.8345302882955,
0.));
#23796=CARTESIAN_POINT('Ctrl Pts',(-28.2149191006269,-24.8345302882955,
18.));
#23797=CARTESIAN_POINT('',(-34.762248247709,-26.9738038986839,0.));
#23798=CARTESIAN_POINT('Ctrl Pts',(-28.2149191006269,-24.8345302882955,
0.));
#23799=CARTESIAN_POINT('Ctrl Pts',(-28.2291563988796,-24.8470618363541,
0.));
#23800=CARTESIAN_POINT('Ctrl Pts',(-28.2579420132101,-24.8717258526943,
0.));
#23801=CARTESIAN_POINT('Ctrl Pts',(-28.3020534756061,-24.9075246543798,
0.));
#23802=CARTESIAN_POINT('Ctrl Pts',(-28.3626431274892,-24.9529811166897,
0.));
#23803=CARTESIAN_POINT('Ctrl Pts',(-28.4408053900206,-25.0066999111736,
0.));
#23804=CARTESIAN_POINT('Ctrl Pts',(-28.5207164321473,-25.0581926620043,
0.));
#23805=CARTESIAN_POINT('Ctrl Pts',(-28.6017081342376,-25.108321158239,0.));
#23806=CARTESIAN_POINT('Ctrl Pts',(-28.6832861366762,-25.1577170374459,
0.));
#23807=CARTESIAN_POINT('Ctrl Pts',(-28.7652594076549,-25.2066127148845,
0.));
#23808=CARTESIAN_POINT('Ctrl Pts',(-28.8476372998748,-25.2549775629725,
0.));
#23809=CARTESIAN_POINT('Ctrl Pts',(-28.9305499160476,-25.3026235249214,
0.));
#23810=CARTESIAN_POINT('Ctrl Pts',(-29.0141637699076,-25.3493168206005,
0.));
#23811=CARTESIAN_POINT('Ctrl Pts',(-29.098589927237,-25.3948997321279,0.));
#23812=CARTESIAN_POINT('Ctrl Pts',(-29.183825549991,-25.4393679214513,0.));
#23813=CARTESIAN_POINT('Ctrl Pts',(-29.2698007967907,-25.4828076101654,
0.));
#23814=CARTESIAN_POINT('Ctrl Pts',(-29.356408021119,-25.5253562922582,0.));
#23815=CARTESIAN_POINT('Ctrl Pts',(-29.443535683207,-25.5671572096726,0.));
#23816=CARTESIAN_POINT('Ctrl Pts',(-29.5311055094509,-25.6083094352667,
0.));
#23817=CARTESIAN_POINT('Ctrl Pts',(-29.6190903904157,-25.6488438125835,
0.));
#23818=CARTESIAN_POINT('Ctrl Pts',(-29.7074935910931,-25.6887507922748,
0.));
#23819=CARTESIAN_POINT('Ctrl Pts',(-29.7963360859334,-25.7279973711305,
0.));
#23820=CARTESIAN_POINT('Ctrl Pts',(-29.8856417535786,-25.7665469042913,
0.));
#23821=CARTESIAN_POINT('Ctrl Pts',(-29.9754208429384,-25.8043812318214,
0.));
#23822=CARTESIAN_POINT('Ctrl Pts',(-30.0656638016321,-25.8415089241134,
0.));
#23823=CARTESIAN_POINT('Ctrl Pts',(-30.1563500154165,-25.8779535511027,
0.));
#23824=CARTESIAN_POINT('Ctrl Pts',(-30.2474530144827,-25.9137466853317,
0.));
#23825=CARTESIAN_POINT('Ctrl Pts',(-30.3389466074503,-25.9489196635424,
0.));
#23826=CARTESIAN_POINT('Ctrl Pts',(-30.4308118142473,-25.9834942765902,
0.));
#23827=CARTESIAN_POINT('Ctrl Pts',(-30.5230388264271,-26.0174801292225,
0.));
#23828=CARTESIAN_POINT('Ctrl Pts',(-30.6156232634061,-26.0508796503166,
0.));
#23829=CARTESIAN_POINT('Ctrl Pts',(-30.7085638682391,-26.0836911730968,
0.));
#23830=CARTESIAN_POINT('Ctrl Pts',(-30.8018598357461,-26.1159125093178,
0.));
#23831=CARTESIAN_POINT('Ctrl Pts',(-30.8955077633644,-26.1475450294082,
0.));
#23832=CARTESIAN_POINT('Ctrl Pts',(-30.9895009017073,-26.1785946616165,
0.));
#23833=CARTESIAN_POINT('Ctrl Pts',(-31.0838307058369,-26.2090698085494,
0.));
#23834=CARTESIAN_POINT('Ctrl Pts',(-31.1784877826858,-26.2389800738215,
0.));
#23835=CARTESIAN_POINT('Ctrl Pts',(-31.2734629900041,-26.2683347859175,
0.));
#23836=CARTESIAN_POINT('Ctrl Pts',(-31.3687486937246,-26.2971413115295,
0.));
#23837=CARTESIAN_POINT('Ctrl Pts',(-31.4643390378084,-26.3254046890485,
0.));
#23838=CARTESIAN_POINT('Ctrl Pts',(-31.5602292672984,-26.353128528169,0.));
#23839=CARTESIAN_POINT('Ctrl Pts',(-31.6564152990236,-26.3803155790949,
0.));
#23840=CARTESIAN_POINT('Ctrl Pts',(-31.7528932299312,-26.4069683862784,
0.));
#23841=CARTESIAN_POINT('Ctrl Pts',(-31.849658771403,-26.433090040836,0.));
#23842=CARTESIAN_POINT('Ctrl Pts',(-31.9467071093816,-26.4586843683627,
0.));
#23843=CARTESIAN_POINT('Ctrl Pts',(-32.0440331917233,-26.4837555495616,
0.));
#23844=CARTESIAN_POINT('Ctrl Pts',(-32.1416319023705,-26.5083078928862,
0.));
#23845=CARTESIAN_POINT('Ctrl Pts',(-32.2394982626669,-26.5323455701117,
0.));
#23846=CARTESIAN_POINT('Ctrl Pts',(-32.3376276606981,-26.5558723200361,
0.));
#23847=CARTESIAN_POINT('Ctrl Pts',(-32.4360159072985,-26.5788913672813,
0.));
#23848=CARTESIAN_POINT('Ctrl Pts',(-32.5346590925498,-26.6014055904817,
0.));
#23849=CARTESIAN_POINT('Ctrl Pts',(-32.6335534898936,-26.6234176311245,
0.));
#23850=CARTESIAN_POINT('Ctrl Pts',(-32.7326954489334,-26.6449300199763,
0.));
#23851=CARTESIAN_POINT('Ctrl Pts',(-32.8320812678271,-26.6659453236976,
0.));
#23852=CARTESIAN_POINT('Ctrl Pts',(-32.9317071576181,-26.6864661988935,
0.));
#23853=CARTESIAN_POINT('Ctrl Pts',(-33.03156933761,-26.7064953106254,0.));
#23854=CARTESIAN_POINT('Ctrl Pts',(-33.131664100194,-26.7260352861619,0.));
#23855=CARTESIAN_POINT('Ctrl Pts',(-33.2319878786519,-26.7450886617884,
0.));
#23856=CARTESIAN_POINT('Ctrl Pts',(-33.3325373307046,-26.7636578270526,
0.));
#23857=CARTESIAN_POINT('Ctrl Pts',(-33.4333093513694,-26.7817450041181,
0.));
#23858=CARTESIAN_POINT('Ctrl Pts',(-33.5343009499673,-26.7993522966985,
0.));
#23859=CARTESIAN_POINT('Ctrl Pts',(-33.6355091508895,-26.8164817280846,
0.));
#23860=CARTESIAN_POINT('Ctrl Pts',(-33.7369308933173,-26.8331352836666,
0.));
#23861=CARTESIAN_POINT('Ctrl Pts',(-33.838562905895,-26.8493149627661,0.));
#23862=CARTESIAN_POINT('Ctrl Pts',(-33.9404016650487,-26.8650228056313,
0.));
#23863=CARTESIAN_POINT('Ctrl Pts',(-34.0424436187397,-26.880260834701,0.));
#23864=CARTESIAN_POINT('Ctrl Pts',(-34.1446853651051,-26.8950310138939,
0.));
#23865=CARTESIAN_POINT('Ctrl Pts',(-34.2471238425419,-26.9093352037262,
0.));
#23866=CARTESIAN_POINT('Ctrl Pts',(-34.3497565255724,-26.9231751225177,
0.));
#23867=CARTESIAN_POINT('Ctrl Pts',(-34.4731465943772,-26.9392277420462,
0.));
#23868=CARTESIAN_POINT('Ctrl Pts',(-34.5762105502273,-26.9520281195268,
0.));
#23869=CARTESIAN_POINT('Ctrl Pts',(-34.6588137898952,-26.9619003236529,
0.));
#23870=CARTESIAN_POINT('Ctrl Pts',(-34.7208516760814,-26.9690976283147,
0.));
#23871=CARTESIAN_POINT('Ctrl Pts',(-34.7622482477091,-26.9738038986838,
0.));
#23872=CARTESIAN_POINT('',(-34.762248247709,-26.9738038986839,15.));
#23873=CARTESIAN_POINT('Ctrl Pts',(-34.7622482477091,-26.9738038986838,
15.));
#23874=CARTESIAN_POINT('Ctrl Pts',(-34.7415499619104,-26.9714507634923,
15.));
#23875=CARTESIAN_POINT('Ctrl Pts',(-34.700172380686,-26.9666985267608,15.));
#23876=CARTESIAN_POINT('Ctrl Pts',(-34.6381629799782,-26.9594322726214,
15.));
#23877=CARTESIAN_POINT('Ctrl Pts',(-34.5555977590573,-26.9494680440307,
15.));
#23878=CARTESIAN_POINT('Ctrl Pts',(-34.4525815829097,-26.9365523054581,
15.));
#23879=CARTESIAN_POINT('Ctrl Pts',(-34.3497565255724,-26.9231751225177,
15.));
#23880=CARTESIAN_POINT('Ctrl Pts',(-34.2471238425419,-26.9093352037262,
15.));
#23881=CARTESIAN_POINT('Ctrl Pts',(-34.1446853651051,-26.8950310138939,
15.));
#23882=CARTESIAN_POINT('Ctrl Pts',(-34.0424436187397,-26.880260834701,15.));
#23883=CARTESIAN_POINT('Ctrl Pts',(-33.9404016650487,-26.8650228056313,
15.));
#23884=CARTESIAN_POINT('Ctrl Pts',(-33.838562905895,-26.8493149627661,15.));
#23885=CARTESIAN_POINT('Ctrl Pts',(-33.7369308933173,-26.8331352836666,
15.));
#23886=CARTESIAN_POINT('Ctrl Pts',(-33.6355091508895,-26.8164817280846,
15.));
#23887=CARTESIAN_POINT('Ctrl Pts',(-33.5343009499673,-26.7993522966985,
15.));
#23888=CARTESIAN_POINT('Ctrl Pts',(-33.4333093513694,-26.7817450041181,
15.));
#23889=CARTESIAN_POINT('Ctrl Pts',(-33.3325373307046,-26.7636578270526,
15.));
#23890=CARTESIAN_POINT('Ctrl Pts',(-33.2319878786519,-26.7450886617884,
15.));
#23891=CARTESIAN_POINT('Ctrl Pts',(-33.131664100194,-26.7260352861619,15.));
#23892=CARTESIAN_POINT('Ctrl Pts',(-33.03156933761,-26.7064953106254,15.));
#23893=CARTESIAN_POINT('Ctrl Pts',(-32.9317071576181,-26.6864661988935,
15.));
#23894=CARTESIAN_POINT('Ctrl Pts',(-32.8320812678271,-26.6659453236976,
15.));
#23895=CARTESIAN_POINT('Ctrl Pts',(-32.7326954489334,-26.6449300199763,
15.));
#23896=CARTESIAN_POINT('Ctrl Pts',(-32.6335534898936,-26.6234176311245,
15.));
#23897=CARTESIAN_POINT('Ctrl Pts',(-32.5346590925498,-26.6014055904817,
15.));
#23898=CARTESIAN_POINT('Ctrl Pts',(-32.4360159072985,-26.5788913672813,
15.));
#23899=CARTESIAN_POINT('Ctrl Pts',(-32.3376276606981,-26.5558723200361,
15.));
#23900=CARTESIAN_POINT('Ctrl Pts',(-32.2394982626669,-26.5323455701117,
15.));
#23901=CARTESIAN_POINT('Ctrl Pts',(-32.1416319023705,-26.5083078928862,
15.));
#23902=CARTESIAN_POINT('Ctrl Pts',(-32.0440331917233,-26.4837555495616,
15.));
#23903=CARTESIAN_POINT('Ctrl Pts',(-31.9467071093816,-26.4586843683627,
15.));
#23904=CARTESIAN_POINT('Ctrl Pts',(-31.849658771403,-26.433090040836,15.));
#23905=CARTESIAN_POINT('Ctrl Pts',(-31.7528932299312,-26.4069683862784,
15.));
#23906=CARTESIAN_POINT('Ctrl Pts',(-31.6564152990236,-26.3803155790949,
15.));
#23907=CARTESIAN_POINT('Ctrl Pts',(-31.5602292672984,-26.353128528169,15.));
#23908=CARTESIAN_POINT('Ctrl Pts',(-31.4643390378084,-26.3254046890485,
15.));
#23909=CARTESIAN_POINT('Ctrl Pts',(-31.3687486937246,-26.2971413115295,
15.));
#23910=CARTESIAN_POINT('Ctrl Pts',(-31.2734629900041,-26.2683347859175,
15.));
#23911=CARTESIAN_POINT('Ctrl Pts',(-31.1784877826858,-26.2389800738215,
15.));
#23912=CARTESIAN_POINT('Ctrl Pts',(-31.0838307058369,-26.2090698085494,
15.));
#23913=CARTESIAN_POINT('Ctrl Pts',(-30.9895009017073,-26.1785946616165,
15.));
#23914=CARTESIAN_POINT('Ctrl Pts',(-30.8955077633644,-26.1475450294082,
15.));
#23915=CARTESIAN_POINT('Ctrl Pts',(-30.8018598357461,-26.1159125093178,
15.));
#23916=CARTESIAN_POINT('Ctrl Pts',(-30.7085638682391,-26.0836911730968,
15.));
#23917=CARTESIAN_POINT('Ctrl Pts',(-30.6156232634061,-26.0508796503166,
15.));
#23918=CARTESIAN_POINT('Ctrl Pts',(-30.5230388264271,-26.0174801292225,
15.));
#23919=CARTESIAN_POINT('Ctrl Pts',(-30.4308118142473,-25.9834942765902,
15.));
#23920=CARTESIAN_POINT('Ctrl Pts',(-30.3389466074503,-25.9489196635424,
15.));
#23921=CARTESIAN_POINT('Ctrl Pts',(-30.2474530144827,-25.9137466853317,
15.));
#23922=CARTESIAN_POINT('Ctrl Pts',(-30.1563500154165,-25.8779535511027,
15.));
#23923=CARTESIAN_POINT('Ctrl Pts',(-30.0656638016321,-25.8415089241134,
15.));
#23924=CARTESIAN_POINT('Ctrl Pts',(-29.9754208429384,-25.8043812318214,
15.));
#23925=CARTESIAN_POINT('Ctrl Pts',(-29.8856417535786,-25.7665469042913,
15.));
#23926=CARTESIAN_POINT('Ctrl Pts',(-29.7963360859334,-25.7279973711305,
15.));
#23927=CARTESIAN_POINT('Ctrl Pts',(-29.7074935910931,-25.6887507922748,
15.));
#23928=CARTESIAN_POINT('Ctrl Pts',(-29.6190903904157,-25.6488438125835,
15.));
#23929=CARTESIAN_POINT('Ctrl Pts',(-29.5311055094509,-25.6083094352667,
15.));
#23930=CARTESIAN_POINT('Ctrl Pts',(-29.443535683207,-25.5671572096726,15.));
#23931=CARTESIAN_POINT('Ctrl Pts',(-29.356408021119,-25.5253562922582,15.));
#23932=CARTESIAN_POINT('Ctrl Pts',(-29.2698007967907,-25.4828076101654,
15.));
#23933=CARTESIAN_POINT('Ctrl Pts',(-29.183825549991,-25.4393679214513,15.));
#23934=CARTESIAN_POINT('Ctrl Pts',(-29.098589927237,-25.3948997321279,15.));
#23935=CARTESIAN_POINT('Ctrl Pts',(-29.0141637699076,-25.3493168206005,
15.));
#23936=CARTESIAN_POINT('Ctrl Pts',(-28.9305499160476,-25.3026235249214,
15.));
#23937=CARTESIAN_POINT('Ctrl Pts',(-28.8476372998748,-25.2549775629725,
15.));
#23938=CARTESIAN_POINT('Ctrl Pts',(-28.7652594076549,-25.2066127148845,
15.));
#23939=CARTESIAN_POINT('Ctrl Pts',(-28.6832861366762,-25.1577170374459,
15.));
#23940=CARTESIAN_POINT('Ctrl Pts',(-28.6017081342376,-25.108321158239,15.));
#23941=CARTESIAN_POINT('Ctrl Pts',(-28.5207164321473,-25.0581926620043,
15.));
#23942=CARTESIAN_POINT('Ctrl Pts',(-28.4408053900206,-25.0066999111736,
15.));
#23943=CARTESIAN_POINT('Ctrl Pts',(-28.3626431274892,-24.9529811166897,
15.));
#23944=CARTESIAN_POINT('Ctrl Pts',(-28.3020534756061,-24.9075246543798,
15.));
#23945=CARTESIAN_POINT('Ctrl Pts',(-28.2579420132101,-24.8717258526943,
15.));
#23946=CARTESIAN_POINT('Ctrl Pts',(-28.2291563988796,-24.8470618363541,
15.));
#23947=CARTESIAN_POINT('Ctrl Pts',(-28.2149191006269,-24.8345302882955,
15.));
#23948=CARTESIAN_POINT('',(-34.762248247709,-26.9738038986839,0.));
#23949=CARTESIAN_POINT('Origin',(-9.16871631793044E-12,-6.66146233219319E-12,
0.));
#23950=CARTESIAN_POINT('',(-36.3957374383337,-24.725498909423,0.));
#23951=CARTESIAN_POINT('Origin',(-9.16871631793044E-12,-6.66146233219319E-12,
0.));
#23952=CARTESIAN_POINT('',(-36.3957374383337,-24.725498909423,15.));
#23953=CARTESIAN_POINT('Origin',(-9.16871631793044E-12,-6.66146233219319E-12,
15.));
#23954=CARTESIAN_POINT('',(-36.3957374383337,-24.725498909423,0.));
#23955=CARTESIAN_POINT('Ctrl Pts',(-32.3379313568208,-19.1596907609891,
0.));
#23956=CARTESIAN_POINT('Ctrl Pts',(-32.3379313568208,-19.1596907609891,
18.));
#23957=CARTESIAN_POINT('Ctrl Pts',(-32.3542491343753,-19.1693587749508,
0.));
#23958=CARTESIAN_POINT('Ctrl Pts',(-32.3542491343753,-19.1693587749508,
18.));
#23959=CARTESIAN_POINT('Ctrl Pts',(-32.3866012518553,-19.1891139208368,
0.));
#23960=CARTESIAN_POINT('Ctrl Pts',(-32.3866012518553,-19.1891139208368,
18.));
#23961=CARTESIAN_POINT('Ctrl Pts',(-32.4342791270009,-19.2200039764927,
0.));
#23962=CARTESIAN_POINT('Ctrl Pts',(-32.4342791270009,-19.2200039764927,
18.));
#23963=CARTESIAN_POINT('Ctrl Pts',(-32.4962340238036,-19.2635813403783,
0.));
#23964=CARTESIAN_POINT('Ctrl Pts',(-32.4962340238036,-19.2635813403783,
18.));
#23965=CARTESIAN_POINT('Ctrl Pts',(-32.5714771007861,-19.3213180490743,
0.));
#23966=CARTESIAN_POINT('Ctrl Pts',(-32.5714771007861,-19.3213180490743,
18.));
#23967=CARTESIAN_POINT('Ctrl Pts',(-32.6451434870609,-19.381405831319,0.));
#23968=CARTESIAN_POINT('Ctrl Pts',(-32.6451434870609,-19.381405831319,18.));
#23969=CARTESIAN_POINT('Ctrl Pts',(-32.7178463324062,-19.4429429601189,
0.));
#23970=CARTESIAN_POINT('Ctrl Pts',(-32.7178463324062,-19.4429429601189,
18.));
#23971=CARTESIAN_POINT('Ctrl Pts',(-32.7900335943248,-19.5052640847974,
0.));
#23972=CARTESIAN_POINT('Ctrl Pts',(-32.7900335943248,-19.5052640847974,
18.));
#23973=CARTESIAN_POINT('Ctrl Pts',(-32.8618672807884,-19.5681157030437,
0.));
#23974=CARTESIAN_POINT('Ctrl Pts',(-32.8618672807884,-19.5681157030437,
18.));
#23975=CARTESIAN_POINT('Ctrl Pts',(-32.9333211533788,-19.6315161742485,
0.));
#23976=CARTESIAN_POINT('Ctrl Pts',(-32.9333211533788,-19.6315161742485,
18.));
#23977=CARTESIAN_POINT('Ctrl Pts',(-33.004256563411,-19.6956473461873,0.));
#23978=CARTESIAN_POINT('Ctrl Pts',(-33.004256563411,-19.6956473461873,18.));
#23979=CARTESIAN_POINT('Ctrl Pts',(-33.0745026283418,-19.7607398248651,
0.));
#23980=CARTESIAN_POINT('Ctrl Pts',(-33.0745026283418,-19.7607398248651,
18.));
#23981=CARTESIAN_POINT('Ctrl Pts',(-33.1439436707661,-19.8269479776239,
0.));
#23982=CARTESIAN_POINT('Ctrl Pts',(-33.1439436707661,-19.8269479776239,
18.));
#23983=CARTESIAN_POINT('Ctrl Pts',(-33.2125746879472,-19.8942704458546,
0.));
#23984=CARTESIAN_POINT('Ctrl Pts',(-33.2125746879472,-19.8942704458546,
18.));
#23985=CARTESIAN_POINT('Ctrl Pts',(-33.2804560993213,-19.9626141625205,
0.));
#23986=CARTESIAN_POINT('Ctrl Pts',(-33.2804560993213,-19.9626141625205,
18.));
#23987=CARTESIAN_POINT('Ctrl Pts',(-33.3476854048385,-20.0318342617212,
0.));
#23988=CARTESIAN_POINT('Ctrl Pts',(-33.3476854048385,-20.0318342617212,
18.));
#23989=CARTESIAN_POINT('Ctrl Pts',(-33.4143643679979,-20.1017803986381,
0.));
#23990=CARTESIAN_POINT('Ctrl Pts',(-33.4143643679979,-20.1017803986381,
18.));
#23991=CARTESIAN_POINT('Ctrl Pts',(-33.480563024813,-20.1723475154533,0.));
#23992=CARTESIAN_POINT('Ctrl Pts',(-33.480563024813,-20.1723475154533,18.));
#23993=CARTESIAN_POINT('Ctrl Pts',(-33.5463023319603,-20.243500298383,0.));
#23994=CARTESIAN_POINT('Ctrl Pts',(-33.5463023319603,-20.243500298383,18.));
#23995=CARTESIAN_POINT('Ctrl Pts',(-33.6115742164079,-20.3152448035298,
0.));
#23996=CARTESIAN_POINT('Ctrl Pts',(-33.6115742164079,-20.3152448035298,
18.));
#23997=CARTESIAN_POINT('Ctrl Pts',(-33.6763537716992,-20.3876111773341,
0.));
#23998=CARTESIAN_POINT('Ctrl Pts',(-33.6763537716992,-20.3876111773341,
18.));
#23999=CARTESIAN_POINT('Ctrl Pts',(-33.7406135254083,-20.4606334536183,
0.));
#24000=CARTESIAN_POINT('Ctrl Pts',(-33.7406135254083,-20.4606334536183,
18.));
#24001=CARTESIAN_POINT('Ctrl Pts',(-33.8043393734971,-20.5343269914034,
0.));
#24002=CARTESIAN_POINT('Ctrl Pts',(-33.8043393734971,-20.5343269914034,
18.));
#24003=CARTESIAN_POINT('Ctrl Pts',(-33.8675365150454,-20.6086800574386,
0.));
#24004=CARTESIAN_POINT('Ctrl Pts',(-33.8675365150454,-20.6086800574386,
18.));
#24005=CARTESIAN_POINT('Ctrl Pts',(-33.9302209962425,-20.683665762903,0.));
#24006=CARTESIAN_POINT('Ctrl Pts',(-33.9302209962425,-20.683665762903,18.));
#24007=CARTESIAN_POINT('Ctrl Pts',(-33.9924146647395,-20.7592491770603,
0.));
#24008=CARTESIAN_POINT('Ctrl Pts',(-33.9924146647395,-20.7592491770603,
18.));
#24009=CARTESIAN_POINT('Ctrl Pts',(-34.0541392299678,-20.8353957068415,
0.));
#24010=CARTESIAN_POINT('Ctrl Pts',(-34.0541392299678,-20.8353957068415,
18.));
#24011=CARTESIAN_POINT('Ctrl Pts',(-34.1154095510973,-20.9120805673809,
0.));
#24012=CARTESIAN_POINT('Ctrl Pts',(-34.1154095510973,-20.9120805673809,
18.));
#24013=CARTESIAN_POINT('Ctrl Pts',(-34.176231731809,-20.9892914622612,0.));
#24014=CARTESIAN_POINT('Ctrl Pts',(-34.176231731809,-20.9892914622612,18.));
#24015=CARTESIAN_POINT('Ctrl Pts',(-34.2366067284279,-21.0670234747355,
0.));
#24016=CARTESIAN_POINT('Ctrl Pts',(-34.2366067284279,-21.0670234747355,
18.));
#24017=CARTESIAN_POINT('Ctrl Pts',(-34.2965325673384,-21.1452759244399,
0.));
#24018=CARTESIAN_POINT('Ctrl Pts',(-34.2965325673384,-21.1452759244399,
18.));
#24019=CARTESIAN_POINT('Ctrl Pts',(-34.3560069185815,-21.2240487218079,
0.));
#24020=CARTESIAN_POINT('Ctrl Pts',(-34.3560069185815,-21.2240487218079,
18.));
#24021=CARTESIAN_POINT('Ctrl Pts',(-34.4150300340623,-21.3033382073239,
0.));
#24022=CARTESIAN_POINT('Ctrl Pts',(-34.4150300340623,-21.3033382073239,
18.));
#24023=CARTESIAN_POINT('Ctrl Pts',(-34.4736054662052,-21.3831361300104,
0.));
#24024=CARTESIAN_POINT('Ctrl Pts',(-34.4736054662052,-21.3831361300104,
18.));
#24025=CARTESIAN_POINT('Ctrl Pts',(-34.5317385658329,-21.4634317666005,
0.));
#24026=CARTESIAN_POINT('Ctrl Pts',(-34.5317385658329,-21.4634317666005,
18.));
#24027=CARTESIAN_POINT('Ctrl Pts',(-34.5894355639082,-21.5442132160757,
0.));
#24028=CARTESIAN_POINT('Ctrl Pts',(-34.5894355639082,-21.5442132160757,
18.));
#24029=CARTESIAN_POINT('Ctrl Pts',(-34.6467025072367,-21.6254689009796,
0.));
#24030=CARTESIAN_POINT('Ctrl Pts',(-34.6467025072367,-21.6254689009796,
18.));
#24031=CARTESIAN_POINT('Ctrl Pts',(-34.7035440429025,-21.7071892844497,
0.));
#24032=CARTESIAN_POINT('Ctrl Pts',(-34.7035440429025,-21.7071892844497,
18.));
#24033=CARTESIAN_POINT('Ctrl Pts',(-34.7599631530844,-21.7893672401137,
0.));
#24034=CARTESIAN_POINT('Ctrl Pts',(-34.7599631530844,-21.7893672401137,
18.));
#24035=CARTESIAN_POINT('Ctrl Pts',(-34.8159618014436,-21.8719971302817,
0.));
#24036=CARTESIAN_POINT('Ctrl Pts',(-34.8159618014436,-21.8719971302817,
18.));
#24037=CARTESIAN_POINT('Ctrl Pts',(-34.8715413418101,-21.9550742217675,
0.));
#24038=CARTESIAN_POINT('Ctrl Pts',(-34.8715413418101,-21.9550742217675,
18.));
#24039=CARTESIAN_POINT('Ctrl Pts',(-34.9267029879922,-22.0385940162683,
0.));
#24040=CARTESIAN_POINT('Ctrl Pts',(-34.9267029879922,-22.0385940162683,
18.));
#24041=CARTESIAN_POINT('Ctrl Pts',(-34.9814483545602,-22.1225514798584,
0.));
#24042=CARTESIAN_POINT('Ctrl Pts',(-34.9814483545602,-22.1225514798584,
18.));
#24043=CARTESIAN_POINT('Ctrl Pts',(-35.0357795922459,-22.2069408519232,
0.));
#24044=CARTESIAN_POINT('Ctrl Pts',(-35.0357795922459,-22.2069408519232,
18.));
#24045=CARTESIAN_POINT('Ctrl Pts',(-35.0896991159359,-22.2917560356803,
0.));
#24046=CARTESIAN_POINT('Ctrl Pts',(-35.0896991159359,-22.2917560356803,
18.));
#24047=CARTESIAN_POINT('Ctrl Pts',(-35.1432094422642,-22.3769908340843,
0.));
#24048=CARTESIAN_POINT('Ctrl Pts',(-35.1432094422642,-22.3769908340843,
18.));
#24049=CARTESIAN_POINT('Ctrl Pts',(-35.1963130003352,-22.4626392230023,
0.));
#24050=CARTESIAN_POINT('Ctrl Pts',(-35.1963130003352,-22.4626392230023,
18.));
#24051=CARTESIAN_POINT('Ctrl Pts',(-35.2490119207975,-22.5486956608909,
0.));
#24052=CARTESIAN_POINT('Ctrl Pts',(-35.2490119207975,-22.5486956608909,
18.));
#24053=CARTESIAN_POINT('Ctrl Pts',(-35.3013079759252,-22.635155167154,0.));
#24054=CARTESIAN_POINT('Ctrl Pts',(-35.3013079759252,-22.635155167154,18.));
#24055=CARTESIAN_POINT('Ctrl Pts',(-35.3532026952313,-22.7220131336912,
0.));
#24056=CARTESIAN_POINT('Ctrl Pts',(-35.3532026952313,-22.7220131336912,
18.));
#24057=CARTESIAN_POINT('Ctrl Pts',(-35.4046974393492,-22.8092652000706,
0.));
#24058=CARTESIAN_POINT('Ctrl Pts',(-35.4046974393492,-22.8092652000706,
18.));
#24059=CARTESIAN_POINT('Ctrl Pts',(-35.4557934871468,-22.8969071125089,
0.));
#24060=CARTESIAN_POINT('Ctrl Pts',(-35.4557934871468,-22.8969071125089,
18.));
#24061=CARTESIAN_POINT('Ctrl Pts',(-35.5064921357308,-22.9849345572033,
0.));
#24062=CARTESIAN_POINT('Ctrl Pts',(-35.5064921357308,-22.9849345572033,
18.));
#24063=CARTESIAN_POINT('Ctrl Pts',(-35.5567947408311,-23.0733431097058,
0.));
#24064=CARTESIAN_POINT('Ctrl Pts',(-35.5567947408311,-23.0733431097058,
18.));
#24065=CARTESIAN_POINT('Ctrl Pts',(-35.6067026687722,-23.1621283508111,
0.));
#24066=CARTESIAN_POINT('Ctrl Pts',(-35.6067026687722,-23.1621283508111,
18.));
#24067=CARTESIAN_POINT('Ctrl Pts',(-35.6562172725207,-23.2512859425032,
0.));
#24068=CARTESIAN_POINT('Ctrl Pts',(-35.6562172725207,-23.2512859425032,
18.));
#24069=CARTESIAN_POINT('Ctrl Pts',(-35.7053398620512,-23.3408117088761,
0.));
#24070=CARTESIAN_POINT('Ctrl Pts',(-35.7053398620512,-23.3408117088761,
18.));
#24071=CARTESIAN_POINT('Ctrl Pts',(-35.7540716771372,-23.4307017328227,
0.));
#24072=CARTESIAN_POINT('Ctrl Pts',(-35.7540716771372,-23.4307017328227,
18.));
#24073=CARTESIAN_POINT('Ctrl Pts',(-35.8024138716897,-23.5209523746427,
0.));
#24074=CARTESIAN_POINT('Ctrl Pts',(-35.8024138716897,-23.5209523746427,
18.));
#24075=CARTESIAN_POINT('Ctrl Pts',(-35.8503675222885,-23.611560139948,0.));
#24076=CARTESIAN_POINT('Ctrl Pts',(-35.8503675222885,-23.611560139948,18.));
#24077=CARTESIAN_POINT('Ctrl Pts',(-35.8979336336837,-23.7025215735353,
0.));
#24078=CARTESIAN_POINT('Ctrl Pts',(-35.8979336336837,-23.7025215735353,
18.));
#24079=CARTESIAN_POINT('Ctrl Pts',(-35.9451131482488,-23.7938331508737,
0.));
#24080=CARTESIAN_POINT('Ctrl Pts',(-35.9451131482488,-23.7938331508737,
18.));
#24081=CARTESIAN_POINT('Ctrl Pts',(-35.991906956547,-23.8854911428946,0.));
#24082=CARTESIAN_POINT('Ctrl Pts',(-35.991906956547,-23.8854911428946,18.));
#24083=CARTESIAN_POINT('Ctrl Pts',(-36.0383159101254,-23.9774915680089,
0.));
#24084=CARTESIAN_POINT('Ctrl Pts',(-36.0383159101254,-23.9774915680089,
18.));
#24085=CARTESIAN_POINT('Ctrl Pts',(-36.0843408347974,-24.0698304230588,
0.));
#24086=CARTESIAN_POINT('Ctrl Pts',(-36.0843408347974,-24.0698304230588,
18.));
#24087=CARTESIAN_POINT('Ctrl Pts',(-36.1299825471271,-24.1625038657964,
0.));
#24088=CARTESIAN_POINT('Ctrl Pts',(-36.1299825471271,-24.1625038657964,
18.));
#24089=CARTESIAN_POINT('Ctrl Pts',(-36.1752418704833,-24.2555084095332,
0.));
#24090=CARTESIAN_POINT('Ctrl Pts',(-36.1752418704833,-24.2555084095332,
18.));
#24091=CARTESIAN_POINT('Ctrl Pts',(-36.2201196586697,-24.3488411214068,
0.));
#24092=CARTESIAN_POINT('Ctrl Pts',(-36.2201196586697,-24.3488411214068,
18.));
#24093=CARTESIAN_POINT('Ctrl Pts',(-36.2646168058396,-24.4424997853605,
0.));
#24094=CARTESIAN_POINT('Ctrl Pts',(-36.2646168058396,-24.4424997853605,
18.));
#24095=CARTESIAN_POINT('Ctrl Pts',(-36.308734152297,-24.5364828082556,0.));
#24096=CARTESIAN_POINT('Ctrl Pts',(-36.308734152297,-24.5364828082556,18.));
#24097=CARTESIAN_POINT('Ctrl Pts',(-36.3437247532369,-24.6119278836614,
0.));
#24098=CARTESIAN_POINT('Ctrl Pts',(-36.3437247532369,-24.6119278836614,
18.));
#24099=CARTESIAN_POINT('Ctrl Pts',(-36.369797330215,-24.6686569322616,0.));
#24100=CARTESIAN_POINT('Ctrl Pts',(-36.369797330215,-24.6686569322616,18.));
#24101=CARTESIAN_POINT('Ctrl Pts',(-36.3871033517098,-24.7065408286023,
0.));
#24102=CARTESIAN_POINT('Ctrl Pts',(-36.3871033517098,-24.7065408286023,
18.));
#24103=CARTESIAN_POINT('Ctrl Pts',(-36.3957374383337,-24.725498909423,0.));
#24104=CARTESIAN_POINT('Ctrl Pts',(-36.3957374383337,-24.725498909423,18.));
#24105=CARTESIAN_POINT('Ctrl Pts',(-32.3379313568208,-19.1596907609891,
0.));
#24106=CARTESIAN_POINT('Ctrl Pts',(-32.3542491343753,-19.1693587749508,
0.));
#24107=CARTESIAN_POINT('Ctrl Pts',(-32.3866012518553,-19.1891139208368,
0.));
#24108=CARTESIAN_POINT('Ctrl Pts',(-32.4342791270009,-19.2200039764927,
0.));
#24109=CARTESIAN_POINT('Ctrl Pts',(-32.4962340238036,-19.2635813403783,
0.));
#24110=CARTESIAN_POINT('Ctrl Pts',(-32.5714771007861,-19.3213180490743,
0.));
#24111=CARTESIAN_POINT('Ctrl Pts',(-32.6451434870609,-19.381405831319,0.));
#24112=CARTESIAN_POINT('Ctrl Pts',(-32.7178463324062,-19.4429429601189,
0.));
#24113=CARTESIAN_POINT('Ctrl Pts',(-32.7900335943248,-19.5052640847974,
0.));
#24114=CARTESIAN_POINT('Ctrl Pts',(-32.8618672807884,-19.5681157030437,
0.));
#24115=CARTESIAN_POINT('Ctrl Pts',(-32.9333211533788,-19.6315161742485,
0.));
#24116=CARTESIAN_POINT('Ctrl Pts',(-33.004256563411,-19.6956473461873,0.));
#24117=CARTESIAN_POINT('Ctrl Pts',(-33.0745026283418,-19.7607398248651,
0.));
#24118=CARTESIAN_POINT('Ctrl Pts',(-33.1439436707661,-19.8269479776239,
0.));
#24119=CARTESIAN_POINT('Ctrl Pts',(-33.2125746879472,-19.8942704458546,
0.));
#24120=CARTESIAN_POINT('Ctrl Pts',(-33.2804560993213,-19.9626141625205,
0.));
#24121=CARTESIAN_POINT('Ctrl Pts',(-33.3476854048385,-20.0318342617212,
0.));
#24122=CARTESIAN_POINT('Ctrl Pts',(-33.4143643679979,-20.1017803986381,
0.));
#24123=CARTESIAN_POINT('Ctrl Pts',(-33.480563024813,-20.1723475154533,0.));
#24124=CARTESIAN_POINT('Ctrl Pts',(-33.5463023319603,-20.243500298383,0.));
#24125=CARTESIAN_POINT('Ctrl Pts',(-33.6115742164079,-20.3152448035298,
0.));
#24126=CARTESIAN_POINT('Ctrl Pts',(-33.6763537716992,-20.3876111773341,
0.));
#24127=CARTESIAN_POINT('Ctrl Pts',(-33.7406135254083,-20.4606334536183,
0.));
#24128=CARTESIAN_POINT('Ctrl Pts',(-33.8043393734971,-20.5343269914034,
0.));
#24129=CARTESIAN_POINT('Ctrl Pts',(-33.8675365150454,-20.6086800574386,
0.));
#24130=CARTESIAN_POINT('Ctrl Pts',(-33.9302209962425,-20.683665762903,0.));
#24131=CARTESIAN_POINT('Ctrl Pts',(-33.9924146647395,-20.7592491770603,
0.));
#24132=CARTESIAN_POINT('Ctrl Pts',(-34.0541392299678,-20.8353957068415,
0.));
#24133=CARTESIAN_POINT('Ctrl Pts',(-34.1154095510973,-20.9120805673809,
0.));
#24134=CARTESIAN_POINT('Ctrl Pts',(-34.176231731809,-20.9892914622612,0.));
#24135=CARTESIAN_POINT('Ctrl Pts',(-34.2366067284279,-21.0670234747355,
0.));
#24136=CARTESIAN_POINT('Ctrl Pts',(-34.2965325673384,-21.1452759244399,
0.));
#24137=CARTESIAN_POINT('Ctrl Pts',(-34.3560069185815,-21.2240487218079,
0.));
#24138=CARTESIAN_POINT('Ctrl Pts',(-34.4150300340623,-21.3033382073239,
0.));
#24139=CARTESIAN_POINT('Ctrl Pts',(-34.4736054662052,-21.3831361300104,
0.));
#24140=CARTESIAN_POINT('Ctrl Pts',(-34.5317385658329,-21.4634317666005,
0.));
#24141=CARTESIAN_POINT('Ctrl Pts',(-34.5894355639082,-21.5442132160757,
0.));
#24142=CARTESIAN_POINT('Ctrl Pts',(-34.6467025072367,-21.6254689009796,
0.));
#24143=CARTESIAN_POINT('Ctrl Pts',(-34.7035440429025,-21.7071892844497,
0.));
#24144=CARTESIAN_POINT('Ctrl Pts',(-34.7599631530844,-21.7893672401137,
0.));
#24145=CARTESIAN_POINT('Ctrl Pts',(-34.8159618014436,-21.8719971302817,
0.));
#24146=CARTESIAN_POINT('Ctrl Pts',(-34.8715413418101,-21.9550742217675,
0.));
#24147=CARTESIAN_POINT('Ctrl Pts',(-34.9267029879922,-22.0385940162683,
0.));
#24148=CARTESIAN_POINT('Ctrl Pts',(-34.9814483545602,-22.1225514798584,
0.));
#24149=CARTESIAN_POINT('Ctrl Pts',(-35.0357795922459,-22.2069408519232,
0.));
#24150=CARTESIAN_POINT('Ctrl Pts',(-35.0896991159359,-22.2917560356803,
0.));
#24151=CARTESIAN_POINT('Ctrl Pts',(-35.1432094422642,-22.3769908340843,
0.));
#24152=CARTESIAN_POINT('Ctrl Pts',(-35.1963130003352,-22.4626392230023,
0.));
#24153=CARTESIAN_POINT('Ctrl Pts',(-35.2490119207975,-22.5486956608909,
0.));
#24154=CARTESIAN_POINT('Ctrl Pts',(-35.3013079759252,-22.635155167154,0.));
#24155=CARTESIAN_POINT('Ctrl Pts',(-35.3532026952313,-22.7220131336912,
0.));
#24156=CARTESIAN_POINT('Ctrl Pts',(-35.4046974393492,-22.8092652000706,
0.));
#24157=CARTESIAN_POINT('Ctrl Pts',(-35.4557934871468,-22.8969071125089,
0.));
#24158=CARTESIAN_POINT('Ctrl Pts',(-35.5064921357308,-22.9849345572033,
0.));
#24159=CARTESIAN_POINT('Ctrl Pts',(-35.5567947408311,-23.0733431097058,
0.));
#24160=CARTESIAN_POINT('Ctrl Pts',(-35.6067026687722,-23.1621283508111,
0.));
#24161=CARTESIAN_POINT('Ctrl Pts',(-35.6562172725207,-23.2512859425032,
0.));
#24162=CARTESIAN_POINT('Ctrl Pts',(-35.7053398620512,-23.3408117088761,
0.));
#24163=CARTESIAN_POINT('Ctrl Pts',(-35.7540716771372,-23.4307017328227,
0.));
#24164=CARTESIAN_POINT('Ctrl Pts',(-35.8024138716897,-23.5209523746427,
0.));
#24165=CARTESIAN_POINT('Ctrl Pts',(-35.8503675222885,-23.611560139948,0.));
#24166=CARTESIAN_POINT('Ctrl Pts',(-35.8979336336837,-23.7025215735353,
0.));
#24167=CARTESIAN_POINT('Ctrl Pts',(-35.9451131482488,-23.7938331508737,
0.));
#24168=CARTESIAN_POINT('Ctrl Pts',(-35.991906956547,-23.8854911428946,0.));
#24169=CARTESIAN_POINT('Ctrl Pts',(-36.0383159101254,-23.9774915680089,
0.));
#24170=CARTESIAN_POINT('Ctrl Pts',(-36.0843408347974,-24.0698304230588,
0.));
#24171=CARTESIAN_POINT('Ctrl Pts',(-36.1299825471271,-24.1625038657964,
0.));
#24172=CARTESIAN_POINT('Ctrl Pts',(-36.1752418704833,-24.2555084095332,
0.));
#24173=CARTESIAN_POINT('Ctrl Pts',(-36.2201196586697,-24.3488411214068,
0.));
#24174=CARTESIAN_POINT('Ctrl Pts',(-36.2735162352736,-24.4612315181512,
0.));
#24175=CARTESIAN_POINT('Ctrl Pts',(-36.3175386315529,-24.5552956307817,
0.));
#24176=CARTESIAN_POINT('Ctrl Pts',(-36.3524534604649,-24.630805301288,0.));
#24177=CARTESIAN_POINT('Ctrl Pts',(-36.37846926509,-24.6875827477484,0.));
#24178=CARTESIAN_POINT('Ctrl Pts',(-36.3957374383337,-24.725498909423,0.));
#24179=CARTESIAN_POINT('Ctrl Pts',(-32.3379313568208,-19.1596907609891,
15.));
#24180=CARTESIAN_POINT('Ctrl Pts',(-32.3542491343753,-19.1693587749508,
15.));
#24181=CARTESIAN_POINT('Ctrl Pts',(-32.3866012518553,-19.1891139208368,
15.));
#24182=CARTESIAN_POINT('Ctrl Pts',(-32.4342791270009,-19.2200039764927,
15.));
#24183=CARTESIAN_POINT('Ctrl Pts',(-32.4962340238036,-19.2635813403783,
15.));
#24184=CARTESIAN_POINT('Ctrl Pts',(-32.5714771007861,-19.3213180490743,
15.));
#24185=CARTESIAN_POINT('Ctrl Pts',(-32.6451434870609,-19.381405831319,15.));
#24186=CARTESIAN_POINT('Ctrl Pts',(-32.7178463324062,-19.4429429601189,
15.));
#24187=CARTESIAN_POINT('Ctrl Pts',(-32.7900335943248,-19.5052640847974,
15.));
#24188=CARTESIAN_POINT('Ctrl Pts',(-32.8618672807884,-19.5681157030437,
15.));
#24189=CARTESIAN_POINT('Ctrl Pts',(-32.9333211533788,-19.6315161742485,
15.));
#24190=CARTESIAN_POINT('Ctrl Pts',(-33.004256563411,-19.6956473461873,15.));
#24191=CARTESIAN_POINT('Ctrl Pts',(-33.0745026283418,-19.7607398248651,
15.));
#24192=CARTESIAN_POINT('Ctrl Pts',(-33.1439436707661,-19.8269479776239,
15.));
#24193=CARTESIAN_POINT('Ctrl Pts',(-33.2125746879472,-19.8942704458546,
15.));
#24194=CARTESIAN_POINT('Ctrl Pts',(-33.2804560993213,-19.9626141625205,
15.));
#24195=CARTESIAN_POINT('Ctrl Pts',(-33.3476854048385,-20.0318342617212,
15.));
#24196=CARTESIAN_POINT('Ctrl Pts',(-33.4143643679979,-20.1017803986381,
15.));
#24197=CARTESIAN_POINT('Ctrl Pts',(-33.480563024813,-20.1723475154533,15.));
#24198=CARTESIAN_POINT('Ctrl Pts',(-33.5463023319603,-20.243500298383,15.));
#24199=CARTESIAN_POINT('Ctrl Pts',(-33.6115742164079,-20.3152448035298,
15.));
#24200=CARTESIAN_POINT('Ctrl Pts',(-33.6763537716992,-20.3876111773341,
15.));
#24201=CARTESIAN_POINT('Ctrl Pts',(-33.7406135254083,-20.4606334536183,
15.));
#24202=CARTESIAN_POINT('Ctrl Pts',(-33.8043393734971,-20.5343269914034,
15.));
#24203=CARTESIAN_POINT('Ctrl Pts',(-33.8675365150454,-20.6086800574386,
15.));
#24204=CARTESIAN_POINT('Ctrl Pts',(-33.9302209962425,-20.683665762903,15.));
#24205=CARTESIAN_POINT('Ctrl Pts',(-33.9924146647395,-20.7592491770603,
15.));
#24206=CARTESIAN_POINT('Ctrl Pts',(-34.0541392299678,-20.8353957068415,
15.));
#24207=CARTESIAN_POINT('Ctrl Pts',(-34.1154095510973,-20.9120805673809,
15.));
#24208=CARTESIAN_POINT('Ctrl Pts',(-34.176231731809,-20.9892914622612,15.));
#24209=CARTESIAN_POINT('Ctrl Pts',(-34.2366067284279,-21.0670234747355,
15.));
#24210=CARTESIAN_POINT('Ctrl Pts',(-34.2965325673384,-21.1452759244399,
15.));
#24211=CARTESIAN_POINT('Ctrl Pts',(-34.3560069185815,-21.2240487218079,
15.));
#24212=CARTESIAN_POINT('Ctrl Pts',(-34.4150300340623,-21.3033382073239,
15.));
#24213=CARTESIAN_POINT('Ctrl Pts',(-34.4736054662052,-21.3831361300104,
15.));
#24214=CARTESIAN_POINT('Ctrl Pts',(-34.5317385658329,-21.4634317666005,
15.));
#24215=CARTESIAN_POINT('Ctrl Pts',(-34.5894355639082,-21.5442132160757,
15.));
#24216=CARTESIAN_POINT('Ctrl Pts',(-34.6467025072367,-21.6254689009796,
15.));
#24217=CARTESIAN_POINT('Ctrl Pts',(-34.7035440429025,-21.7071892844497,
15.));
#24218=CARTESIAN_POINT('Ctrl Pts',(-34.7599631530844,-21.7893672401137,
15.));
#24219=CARTESIAN_POINT('Ctrl Pts',(-34.8159618014436,-21.8719971302817,
15.));
#24220=CARTESIAN_POINT('Ctrl Pts',(-34.8715413418101,-21.9550742217675,
15.));
#24221=CARTESIAN_POINT('Ctrl Pts',(-34.9267029879922,-22.0385940162683,
15.));
#24222=CARTESIAN_POINT('Ctrl Pts',(-34.9814483545602,-22.1225514798584,
15.));
#24223=CARTESIAN_POINT('Ctrl Pts',(-35.0357795922459,-22.2069408519232,
15.));
#24224=CARTESIAN_POINT('Ctrl Pts',(-35.0896991159359,-22.2917560356803,
15.));
#24225=CARTESIAN_POINT('Ctrl Pts',(-35.1432094422642,-22.3769908340843,
15.));
#24226=CARTESIAN_POINT('Ctrl Pts',(-35.1963130003352,-22.4626392230023,
15.));
#24227=CARTESIAN_POINT('Ctrl Pts',(-35.2490119207975,-22.5486956608909,
15.));
#24228=CARTESIAN_POINT('Ctrl Pts',(-35.3013079759252,-22.635155167154,15.));
#24229=CARTESIAN_POINT('Ctrl Pts',(-35.3532026952313,-22.7220131336912,
15.));
#24230=CARTESIAN_POINT('Ctrl Pts',(-35.4046974393492,-22.8092652000706,
15.));
#24231=CARTESIAN_POINT('Ctrl Pts',(-35.4557934871468,-22.8969071125089,
15.));
#24232=CARTESIAN_POINT('Ctrl Pts',(-35.5064921357308,-22.9849345572033,
15.));
#24233=CARTESIAN_POINT('Ctrl Pts',(-35.5567947408311,-23.0733431097058,
15.));
#24234=CARTESIAN_POINT('Ctrl Pts',(-35.6067026687722,-23.1621283508111,
15.));
#24235=CARTESIAN_POINT('Ctrl Pts',(-35.6562172725207,-23.2512859425032,
15.));
#24236=CARTESIAN_POINT('Ctrl Pts',(-35.7053398620512,-23.3408117088761,
15.));
#24237=CARTESIAN_POINT('Ctrl Pts',(-35.7540716771372,-23.4307017328227,
15.));
#24238=CARTESIAN_POINT('Ctrl Pts',(-35.8024138716897,-23.5209523746427,
15.));
#24239=CARTESIAN_POINT('Ctrl Pts',(-35.8503675222885,-23.611560139948,15.));
#24240=CARTESIAN_POINT('Ctrl Pts',(-35.8979336336837,-23.7025215735353,
15.));
#24241=CARTESIAN_POINT('Ctrl Pts',(-35.9451131482488,-23.7938331508737,
15.));
#24242=CARTESIAN_POINT('Ctrl Pts',(-35.991906956547,-23.8854911428946,15.));
#24243=CARTESIAN_POINT('Ctrl Pts',(-36.0383159101254,-23.9774915680089,
15.));
#24244=CARTESIAN_POINT('Ctrl Pts',(-36.0843408347974,-24.0698304230588,
15.));
#24245=CARTESIAN_POINT('Ctrl Pts',(-36.1299825471271,-24.1625038657964,
15.));
#24246=CARTESIAN_POINT('Ctrl Pts',(-36.1752418704833,-24.2555084095332,
15.));
#24247=CARTESIAN_POINT('Ctrl Pts',(-36.2201196586697,-24.3488411214068,
15.));
#24248=CARTESIAN_POINT('Ctrl Pts',(-36.2735162352736,-24.4612315181512,
15.));
#24249=CARTESIAN_POINT('Ctrl Pts',(-36.3175386315529,-24.5552956307817,
15.));
#24250=CARTESIAN_POINT('Ctrl Pts',(-36.3524534604649,-24.630805301288,15.));
#24251=CARTESIAN_POINT('Ctrl Pts',(-36.37846926509,-24.6875827477484,15.));
#24252=CARTESIAN_POINT('Ctrl Pts',(-36.3957374383337,-24.725498909423,15.));
#24253=CARTESIAN_POINT('Ctrl Pts',(-41.396226524684,-14.911486495888,0.));
#24254=CARTESIAN_POINT('Ctrl Pts',(-41.396226524684,-14.911486495888,18.));
#24255=CARTESIAN_POINT('Ctrl Pts',(-41.3758141263348,-14.9156446533966,
0.));
#24256=CARTESIAN_POINT('Ctrl Pts',(-41.3758141263348,-14.9156446533966,
18.));
#24257=CARTESIAN_POINT('Ctrl Pts',(-41.3349931861715,-14.9239113834707,
0.));
#24258=CARTESIAN_POINT('Ctrl Pts',(-41.3349931861715,-14.9239113834707,
18.));
#24259=CARTESIAN_POINT('Ctrl Pts',(-41.2737733455422,-14.936162723752,0.));
#24260=CARTESIAN_POINT('Ctrl Pts',(-41.2737733455422,-14.936162723752,18.));
#24261=CARTESIAN_POINT('Ctrl Pts',(-41.1921700381957,-14.9522002356298,
0.));
#24262=CARTESIAN_POINT('Ctrl Pts',(-41.1921700381957,-14.9522002356298,
18.));
#24263=CARTESIAN_POINT('Ctrl Pts',(-41.0902046498729,-14.9717503874227,
0.));
#24264=CARTESIAN_POINT('Ctrl Pts',(-41.0902046498729,-14.9717503874227,
18.));
#24265=CARTESIAN_POINT('Ctrl Pts',(-40.9882784321884,-14.9908026205824,
0.));
#24266=CARTESIAN_POINT('Ctrl Pts',(-40.9882784321884,-14.9908026205824,
18.));
#24267=CARTESIAN_POINT('Ctrl Pts',(-40.8863921801,-15.0093553188655,0.));
#24268=CARTESIAN_POINT('Ctrl Pts',(-40.8863921801,-15.0093553188655,18.));
#24269=CARTESIAN_POINT('Ctrl Pts',(-40.7845471608654,-15.0274064563211,
0.));
#24270=CARTESIAN_POINT('Ctrl Pts',(-40.7845471608654,-15.0274064563211,
18.));
#24271=CARTESIAN_POINT('Ctrl Pts',(-40.6827452453667,-15.0449536183143,
0.));
#24272=CARTESIAN_POINT('Ctrl Pts',(-40.6827452453667,-15.0449536183143,
18.));
#24273=CARTESIAN_POINT('Ctrl Pts',(-40.58098877043,-15.0619940893017,0.));
#24274=CARTESIAN_POINT('Ctrl Pts',(-40.58098877043,-15.0619940893017,18.));
#24275=CARTESIAN_POINT('Ctrl Pts',(-40.4792803645352,-15.0785249502524,
0.));
#24276=CARTESIAN_POINT('Ctrl Pts',(-40.4792803645352,-15.0785249502524,
18.));
#24277=CARTESIAN_POINT('Ctrl Pts',(-40.3776227809037,-15.0945431800723,
0.));
#24278=CARTESIAN_POINT('Ctrl Pts',(-40.3776227809037,-15.0945431800723,
18.));
#24279=CARTESIAN_POINT('Ctrl Pts',(-40.2760187401821,-15.1100457495259,
0.));
#24280=CARTESIAN_POINT('Ctrl Pts',(-40.2760187401821,-15.1100457495259,
18.));
#24281=CARTESIAN_POINT('Ctrl Pts',(-40.1744707357902,-15.1250297462408,
0.));
#24282=CARTESIAN_POINT('Ctrl Pts',(-40.1744707357902,-15.1250297462408,
18.));
#24283=CARTESIAN_POINT('Ctrl Pts',(-40.0729810652204,-15.1394923361537,
0.));
#24284=CARTESIAN_POINT('Ctrl Pts',(-40.0729810652204,-15.1394923361537,
18.));
#24285=CARTESIAN_POINT('Ctrl Pts',(-39.9715519332134,-15.1534306754871,
0.));
#24286=CARTESIAN_POINT('Ctrl Pts',(-39.9715519332134,-15.1534306754871,
18.));
#24287=CARTESIAN_POINT('Ctrl Pts',(-39.8701855339908,-15.1668418393198,
0.));
#24288=CARTESIAN_POINT('Ctrl Pts',(-39.8701855339908,-15.1668418393198,
18.));
#24289=CARTESIAN_POINT('Ctrl Pts',(-39.7688841338802,-15.1797227547561,
0.));
#24290=CARTESIAN_POINT('Ctrl Pts',(-39.7688841338802,-15.1797227547561,
18.));
#24291=CARTESIAN_POINT('Ctrl Pts',(-39.6676501731673,-15.1920701163803,
0.));
#24292=CARTESIAN_POINT('Ctrl Pts',(-39.6676501731673,-15.1920701163803,
18.));
#24293=CARTESIAN_POINT('Ctrl Pts',(-39.5664862602472,-15.2038804098649,
0.));
#24294=CARTESIAN_POINT('Ctrl Pts',(-39.5664862602472,-15.2038804098649,
18.));
#24295=CARTESIAN_POINT('Ctrl Pts',(-39.4653951093947,-15.2151499908149,
0.));
#24296=CARTESIAN_POINT('Ctrl Pts',(-39.4653951093947,-15.2151499908149,
18.));
#24297=CARTESIAN_POINT('Ctrl Pts',(-39.3643794927167,-15.2258751563069,
0.));
#24298=CARTESIAN_POINT('Ctrl Pts',(-39.3643794927167,-15.2258751563069,
18.));
#24299=CARTESIAN_POINT('Ctrl Pts',(-39.2634421927888,-15.2360522089072,
0.));
#24300=CARTESIAN_POINT('Ctrl Pts',(-39.2634421927888,-15.2360522089072,
18.));
#24301=CARTESIAN_POINT('Ctrl Pts',(-39.1625859371304,-15.2456775636447,
0.));
#24302=CARTESIAN_POINT('Ctrl Pts',(-39.1625859371304,-15.2456775636447,
18.));
#24303=CARTESIAN_POINT('Ctrl Pts',(-39.061813415425,-15.2547476855825,0.));
#24304=CARTESIAN_POINT('Ctrl Pts',(-39.061813415425,-15.2547476855825,18.));
#24305=CARTESIAN_POINT('Ctrl Pts',(-38.9611273555758,-15.2632589109473,
0.));
#24306=CARTESIAN_POINT('Ctrl Pts',(-38.9611273555758,-15.2632589109473,
18.));
#24307=CARTESIAN_POINT('Ctrl Pts',(-38.860530586589,-15.2712072937639,0.));
#24308=CARTESIAN_POINT('Ctrl Pts',(-38.860530586589,-15.2712072937639,18.));
#24309=CARTESIAN_POINT('Ctrl Pts',(-38.7600260961351,-15.2785884727112,
0.));
#24310=CARTESIAN_POINT('Ctrl Pts',(-38.7600260961351,-15.2785884727112,
18.));
#24311=CARTESIAN_POINT('Ctrl Pts',(-38.659617115053,-15.2853974668211,0.));
#24312=CARTESIAN_POINT('Ctrl Pts',(-38.659617115053,-15.2853974668211,18.));
#24313=CARTESIAN_POINT('Ctrl Pts',(-38.5593070891769,-15.2916287700102,
0.));
#24314=CARTESIAN_POINT('Ctrl Pts',(-38.5593070891769,-15.2916287700102,
18.));
#24315=CARTESIAN_POINT('Ctrl Pts',(-38.4590995527814,-15.2972767037469,
0.));
#24316=CARTESIAN_POINT('Ctrl Pts',(-38.4590995527814,-15.2972767037469,
18.));
#24317=CARTESIAN_POINT('Ctrl Pts',(-38.3589980188324,-15.3023357307483,
0.));
#24318=CARTESIAN_POINT('Ctrl Pts',(-38.3589980188324,-15.3023357307483,
18.));
#24319=CARTESIAN_POINT('Ctrl Pts',(-38.2590058835965,-15.3068007250314,
0.));
#24320=CARTESIAN_POINT('Ctrl Pts',(-38.2590058835965,-15.3068007250314,
18.));
#24321=CARTESIAN_POINT('Ctrl Pts',(-38.1591262705847,-15.310667421514,0.));
#24322=CARTESIAN_POINT('Ctrl Pts',(-38.1591262705847,-15.310667421514,18.));
#24323=CARTESIAN_POINT('Ctrl Pts',(-38.0593621055415,-15.3139321941687,
0.));
#24324=CARTESIAN_POINT('Ctrl Pts',(-38.0593621055415,-15.3139321941687,
18.));
#24325=CARTESIAN_POINT('Ctrl Pts',(-37.959716421934,-15.3165911656268,0.));
#24326=CARTESIAN_POINT('Ctrl Pts',(-37.959716421934,-15.3165911656268,18.));
#24327=CARTESIAN_POINT('Ctrl Pts',(-37.8601926265378,-15.3186394335023,
0.));
#24328=CARTESIAN_POINT('Ctrl Pts',(-37.8601926265378,-15.3186394335023,
18.));
#24329=CARTESIAN_POINT('Ctrl Pts',(-37.7607947318286,-15.320070396385,0.));
#24330=CARTESIAN_POINT('Ctrl Pts',(-37.7607947318286,-15.320070396385,18.));
#24331=CARTESIAN_POINT('Ctrl Pts',(-37.6615277218027,-15.320874689078,0.));
#24332=CARTESIAN_POINT('Ctrl Pts',(-37.6615277218027,-15.320874689078,18.));
#24333=CARTESIAN_POINT('Ctrl Pts',(-37.562397408596,-15.3210406145546,0.));
#24334=CARTESIAN_POINT('Ctrl Pts',(-37.562397408596,-15.3210406145546,18.));
#24335=CARTESIAN_POINT('Ctrl Pts',(-37.4634097578665,-15.3205561366169,
0.));
#24336=CARTESIAN_POINT('Ctrl Pts',(-37.4634097578665,-15.3205561366169,
18.));
#24337=CARTESIAN_POINT('Ctrl Pts',(-37.3645702997848,-15.3194106233801,
0.));
#24338=CARTESIAN_POINT('Ctrl Pts',(-37.3645702997848,-15.3194106233801,
18.));
#24339=CARTESIAN_POINT('Ctrl Pts',(-37.2658836214694,-15.3175963510697,
0.));
#24340=CARTESIAN_POINT('Ctrl Pts',(-37.2658836214694,-15.3175963510697,
18.));
#24341=CARTESIAN_POINT('Ctrl Pts',(-37.1673525354642,-15.3151109648809,
0.));
#24342=CARTESIAN_POINT('Ctrl Pts',(-37.1673525354642,-15.3151109648809,
18.));
#24343=CARTESIAN_POINT('Ctrl Pts',(-37.0689784837457,-15.3119562971444,
0.));
#24344=CARTESIAN_POINT('Ctrl Pts',(-37.0689784837457,-15.3119562971444,
18.));
#24345=CARTESIAN_POINT('Ctrl Pts',(-36.970763176802,-15.3081335446406,0.));
#24346=CARTESIAN_POINT('Ctrl Pts',(-36.970763176802,-15.3081335446406,18.));
#24347=CARTESIAN_POINT('Ctrl Pts',(-36.8727100302512,-15.3036390436952,
0.));
#24348=CARTESIAN_POINT('Ctrl Pts',(-36.8727100302512,-15.3036390436952,
18.));
#24349=CARTESIAN_POINT('Ctrl Pts',(-36.7748254044502,-15.2984606286737,
0.));
#24350=CARTESIAN_POINT('Ctrl Pts',(-36.7748254044502,-15.2984606286737,
18.));
#24351=CARTESIAN_POINT('Ctrl Pts',(-36.6771206167756,-15.2925717100767,
0.));
#24352=CARTESIAN_POINT('Ctrl Pts',(-36.6771206167756,-15.2925717100767,
18.));
#24353=CARTESIAN_POINT('Ctrl Pts',(-36.5796108931244,-15.2859343913094,
0.));
#24354=CARTESIAN_POINT('Ctrl Pts',(-36.5796108931244,-15.2859343913094,
18.));
#24355=CARTESIAN_POINT('Ctrl Pts',(-36.4823116513289,-15.2785104654792,
0.));
#24356=CARTESIAN_POINT('Ctrl Pts',(-36.4823116513289,-15.2785104654792,
18.));
#24357=CARTESIAN_POINT('Ctrl Pts',(-36.3852352131887,-15.2702711460937,
0.));
#24358=CARTESIAN_POINT('Ctrl Pts',(-36.3852352131887,-15.2702711460937,
18.));
#24359=CARTESIAN_POINT('Ctrl Pts',(-36.2883880151607,-15.2612053303773,
0.));
#24360=CARTESIAN_POINT('Ctrl Pts',(-36.2883880151607,-15.2612053303773,
18.));
#24361=CARTESIAN_POINT('Ctrl Pts',(-36.1917659216814,-15.2513334565427,
0.));
#24362=CARTESIAN_POINT('Ctrl Pts',(-36.1917659216814,-15.2513334565427,
18.));
#24363=CARTESIAN_POINT('Ctrl Pts',(-36.095357546697,-15.240697754828,0.));
#24364=CARTESIAN_POINT('Ctrl Pts',(-36.095357546697,-15.240697754828,18.));
#24365=CARTESIAN_POINT('Ctrl Pts',(-35.9991531408727,-15.2293360946131,
0.));
#24366=CARTESIAN_POINT('Ctrl Pts',(-35.9991531408727,-15.2293360946131,
18.));
#24367=CARTESIAN_POINT('Ctrl Pts',(-35.9031525499277,-15.2172585668056,
0.));
#24368=CARTESIAN_POINT('Ctrl Pts',(-35.9031525499277,-15.2172585668056,
18.));
#24369=CARTESIAN_POINT('Ctrl Pts',(-35.8073720252878,-15.2044274601769,
0.));
#24370=CARTESIAN_POINT('Ctrl Pts',(-35.8073720252878,-15.2044274601769,
18.));
#24371=CARTESIAN_POINT('Ctrl Pts',(-35.7118553943773,-15.1907243629658,
0.));
#24372=CARTESIAN_POINT('Ctrl Pts',(-35.7118553943773,-15.1907243629658,
18.));
#24373=CARTESIAN_POINT('Ctrl Pts',(-35.6166644736253,-15.1759785763051,
0.));
#24374=CARTESIAN_POINT('Ctrl Pts',(-35.6166644736253,-15.1759785763051,
18.));
#24375=CARTESIAN_POINT('Ctrl Pts',(-35.5218591529745,-15.1600260710383,
0.));
#24376=CARTESIAN_POINT('Ctrl Pts',(-35.5218591529745,-15.1600260710383,
18.));
#24377=CARTESIAN_POINT('Ctrl Pts',(-35.4274792115856,-15.1427632633831,
0.));
#24378=CARTESIAN_POINT('Ctrl Pts',(-35.4274792115856,-15.1427632633831,
18.));
#24379=CARTESIAN_POINT('Ctrl Pts',(-35.3335286891314,-15.1241934020681,
0.));
#24380=CARTESIAN_POINT('Ctrl Pts',(-35.3335286891314,-15.1241934020681,
18.));
#24381=CARTESIAN_POINT('Ctrl Pts',(-35.2399506932815,-15.104500806927,0.));
#24382=CARTESIAN_POINT('Ctrl Pts',(-35.2399506932815,-15.104500806927,18.));
#24383=CARTESIAN_POINT('Ctrl Pts',(-35.1466591020976,-15.08395927165,0.));
#24384=CARTESIAN_POINT('Ctrl Pts',(-35.1466591020976,-15.08395927165,18.));
#24385=CARTESIAN_POINT('Ctrl Pts',(-35.0535882932913,-15.0627878528202,
0.));
#24386=CARTESIAN_POINT('Ctrl Pts',(-35.0535882932913,-15.0627878528202,
18.));
#24387=CARTESIAN_POINT('Ctrl Pts',(-34.9607388363587,-15.041018569143,0.));
#24388=CARTESIAN_POINT('Ctrl Pts',(-34.9607388363587,-15.041018569143,18.));
#24389=CARTESIAN_POINT('Ctrl Pts',(-34.8682205930809,-15.0183713484962,
0.));
#24390=CARTESIAN_POINT('Ctrl Pts',(-34.8682205930809,-15.0183713484962,
18.));
#24391=CARTESIAN_POINT('Ctrl Pts',(-34.7763085406486,-14.9940927023321,
0.));
#24392=CARTESIAN_POINT('Ctrl Pts',(-34.7763085406486,-14.9940927023321,
18.));
#24393=CARTESIAN_POINT('Ctrl Pts',(-34.6853717911268,-14.9671565602316,
0.));
#24394=CARTESIAN_POINT('Ctrl Pts',(-34.6853717911268,-14.9671565602316,
18.));
#24395=CARTESIAN_POINT('Ctrl Pts',(-34.6137007885254,-14.9426481276593,
0.));
#24396=CARTESIAN_POINT('Ctrl Pts',(-34.6137007885254,-14.9426481276593,
18.));
#24397=CARTESIAN_POINT('Ctrl Pts',(-34.5606858566713,-14.9222326355678,
0.));
#24398=CARTESIAN_POINT('Ctrl Pts',(-34.5606858566713,-14.9222326355678,
18.));
#24399=CARTESIAN_POINT('Ctrl Pts',(-34.525687510388,-14.9076710061311,0.));
#24400=CARTESIAN_POINT('Ctrl Pts',(-34.525687510388,-14.9076710061311,18.));
#24401=CARTESIAN_POINT('Ctrl Pts',(-34.5082745737944,-14.9001523628048,
0.));
#24402=CARTESIAN_POINT('Ctrl Pts',(-34.5082745737944,-14.9001523628048,
18.));
#24403=CARTESIAN_POINT('',(-41.3962265246839,-14.9114864958881,0.));
#24404=CARTESIAN_POINT('Ctrl Pts',(-34.5082745737944,-14.9001523628048,
0.));
#24405=CARTESIAN_POINT('Ctrl Pts',(-34.525687510388,-14.9076710061311,0.));
#24406=CARTESIAN_POINT('Ctrl Pts',(-34.5606858566713,-14.9222326355678,
0.));
#24407=CARTESIAN_POINT('Ctrl Pts',(-34.6137007885254,-14.9426481276593,
0.));
#24408=CARTESIAN_POINT('Ctrl Pts',(-34.6853717911268,-14.9671565602316,
0.));
#24409=CARTESIAN_POINT('Ctrl Pts',(-34.7763085406486,-14.9940927023321,
0.));
#24410=CARTESIAN_POINT('Ctrl Pts',(-34.8682205930809,-15.0183713484962,
0.));
#24411=CARTESIAN_POINT('Ctrl Pts',(-34.9607388363587,-15.041018569143,0.));
#24412=CARTESIAN_POINT('Ctrl Pts',(-35.0535882932913,-15.0627878528202,
0.));
#24413=CARTESIAN_POINT('Ctrl Pts',(-35.1466591020976,-15.08395927165,0.));
#24414=CARTESIAN_POINT('Ctrl Pts',(-35.2399506932815,-15.104500806927,0.));
#24415=CARTESIAN_POINT('Ctrl Pts',(-35.3335286891314,-15.1241934020681,
0.));
#24416=CARTESIAN_POINT('Ctrl Pts',(-35.4274792115856,-15.1427632633831,
0.));
#24417=CARTESIAN_POINT('Ctrl Pts',(-35.5218591529745,-15.1600260710383,
0.));
#24418=CARTESIAN_POINT('Ctrl Pts',(-35.6166644736253,-15.1759785763051,
0.));
#24419=CARTESIAN_POINT('Ctrl Pts',(-35.7118553943773,-15.1907243629658,
0.));
#24420=CARTESIAN_POINT('Ctrl Pts',(-35.8073720252878,-15.2044274601769,
0.));
#24421=CARTESIAN_POINT('Ctrl Pts',(-35.9031525499277,-15.2172585668056,
0.));
#24422=CARTESIAN_POINT('Ctrl Pts',(-35.9991531408727,-15.2293360946131,
0.));
#24423=CARTESIAN_POINT('Ctrl Pts',(-36.095357546697,-15.240697754828,0.));
#24424=CARTESIAN_POINT('Ctrl Pts',(-36.1917659216814,-15.2513334565427,
0.));
#24425=CARTESIAN_POINT('Ctrl Pts',(-36.2883880151607,-15.2612053303773,
0.));
#24426=CARTESIAN_POINT('Ctrl Pts',(-36.3852352131887,-15.2702711460937,
0.));
#24427=CARTESIAN_POINT('Ctrl Pts',(-36.4823116513289,-15.2785104654792,
0.));
#24428=CARTESIAN_POINT('Ctrl Pts',(-36.5796108931244,-15.2859343913094,
0.));
#24429=CARTESIAN_POINT('Ctrl Pts',(-36.6771206167756,-15.2925717100767,
0.));
#24430=CARTESIAN_POINT('Ctrl Pts',(-36.7748254044502,-15.2984606286737,
0.));
#24431=CARTESIAN_POINT('Ctrl Pts',(-36.8727100302512,-15.3036390436952,
0.));
#24432=CARTESIAN_POINT('Ctrl Pts',(-36.970763176802,-15.3081335446406,0.));
#24433=CARTESIAN_POINT('Ctrl Pts',(-37.0689784837457,-15.3119562971444,
0.));
#24434=CARTESIAN_POINT('Ctrl Pts',(-37.1673525354642,-15.3151109648809,
0.));
#24435=CARTESIAN_POINT('Ctrl Pts',(-37.2658836214694,-15.3175963510697,
0.));
#24436=CARTESIAN_POINT('Ctrl Pts',(-37.3645702997848,-15.3194106233801,
0.));
#24437=CARTESIAN_POINT('Ctrl Pts',(-37.4634097578665,-15.3205561366169,
0.));
#24438=CARTESIAN_POINT('Ctrl Pts',(-37.562397408596,-15.3210406145546,0.));
#24439=CARTESIAN_POINT('Ctrl Pts',(-37.6615277218027,-15.320874689078,0.));
#24440=CARTESIAN_POINT('Ctrl Pts',(-37.7607947318286,-15.320070396385,0.));
#24441=CARTESIAN_POINT('Ctrl Pts',(-37.8601926265378,-15.3186394335023,
0.));
#24442=CARTESIAN_POINT('Ctrl Pts',(-37.959716421934,-15.3165911656268,0.));
#24443=CARTESIAN_POINT('Ctrl Pts',(-38.0593621055415,-15.3139321941687,
0.));
#24444=CARTESIAN_POINT('Ctrl Pts',(-38.1591262705847,-15.310667421514,0.));
#24445=CARTESIAN_POINT('Ctrl Pts',(-38.2590058835965,-15.3068007250314,
0.));
#24446=CARTESIAN_POINT('Ctrl Pts',(-38.3589980188324,-15.3023357307483,
0.));
#24447=CARTESIAN_POINT('Ctrl Pts',(-38.4590995527814,-15.2972767037469,
0.));
#24448=CARTESIAN_POINT('Ctrl Pts',(-38.5593070891769,-15.2916287700102,
0.));
#24449=CARTESIAN_POINT('Ctrl Pts',(-38.659617115053,-15.2853974668211,0.));
#24450=CARTESIAN_POINT('Ctrl Pts',(-38.7600260961351,-15.2785884727112,
0.));
#24451=CARTESIAN_POINT('Ctrl Pts',(-38.860530586589,-15.2712072937639,0.));
#24452=CARTESIAN_POINT('Ctrl Pts',(-38.9611273555758,-15.2632589109473,
0.));
#24453=CARTESIAN_POINT('Ctrl Pts',(-39.061813415425,-15.2547476855825,0.));
#24454=CARTESIAN_POINT('Ctrl Pts',(-39.1625859371304,-15.2456775636447,
0.));
#24455=CARTESIAN_POINT('Ctrl Pts',(-39.2634421927888,-15.2360522089072,
0.));
#24456=CARTESIAN_POINT('Ctrl Pts',(-39.3643794927167,-15.2258751563069,
0.));
#24457=CARTESIAN_POINT('Ctrl Pts',(-39.4653951093947,-15.2151499908149,
0.));
#24458=CARTESIAN_POINT('Ctrl Pts',(-39.5664862602472,-15.2038804098649,
0.));
#24459=CARTESIAN_POINT('Ctrl Pts',(-39.6676501731673,-15.1920701163803,
0.));
#24460=CARTESIAN_POINT('Ctrl Pts',(-39.7688841338802,-15.1797227547561,
0.));
#24461=CARTESIAN_POINT('Ctrl Pts',(-39.8701855339908,-15.1668418393198,
0.));
#24462=CARTESIAN_POINT('Ctrl Pts',(-39.9715519332134,-15.1534306754871,
0.));
#24463=CARTESIAN_POINT('Ctrl Pts',(-40.0729810652204,-15.1394923361537,
0.));
#24464=CARTESIAN_POINT('Ctrl Pts',(-40.1744707357902,-15.1250297462408,
0.));
#24465=CARTESIAN_POINT('Ctrl Pts',(-40.2760187401821,-15.1100457495259,
0.));
#24466=CARTESIAN_POINT('Ctrl Pts',(-40.3776227809037,-15.0945431800723,
0.));
#24467=CARTESIAN_POINT('Ctrl Pts',(-40.4792803645352,-15.0785249502524,
0.));
#24468=CARTESIAN_POINT('Ctrl Pts',(-40.58098877043,-15.0619940893017,0.));
#24469=CARTESIAN_POINT('Ctrl Pts',(-40.6827452453667,-15.0449536183143,
0.));
#24470=CARTESIAN_POINT('Ctrl Pts',(-40.7845471608654,-15.0274064563211,
0.));
#24471=CARTESIAN_POINT('Ctrl Pts',(-40.8863921801,-15.0093553188655,0.));
#24472=CARTESIAN_POINT('Ctrl Pts',(-40.9882784321884,-14.9908026205824,
0.));
#24473=CARTESIAN_POINT('Ctrl Pts',(-41.1105898934098,-14.9679399407908,
0.));
#24474=CARTESIAN_POINT('Ctrl Pts',(-41.2125650743922,-14.9482653093396,
0.));
#24475=CARTESIAN_POINT('Ctrl Pts',(-41.2941761025922,-14.9321285285561,
0.));
#24476=CARTESIAN_POINT('Ctrl Pts',(-41.3554017279611,-14.919802810928,0.));
#24477=CARTESIAN_POINT('Ctrl Pts',(-41.396226524684,-14.911486495888,0.));
#24478=CARTESIAN_POINT('',(-41.3962265246839,-14.9114864958881,15.));
#24479=CARTESIAN_POINT('Ctrl Pts',(-41.396226524684,-14.911486495888,15.));
#24480=CARTESIAN_POINT('Ctrl Pts',(-41.3758141263348,-14.9156446533966,
15.));
#24481=CARTESIAN_POINT('Ctrl Pts',(-41.3349931861715,-14.9239113834707,
15.));
#24482=CARTESIAN_POINT('Ctrl Pts',(-41.2737733455422,-14.936162723752,15.));
#24483=CARTESIAN_POINT('Ctrl Pts',(-41.1921700381957,-14.9522002356298,
15.));
#24484=CARTESIAN_POINT('Ctrl Pts',(-41.0902046498729,-14.9717503874227,
15.));
#24485=CARTESIAN_POINT('Ctrl Pts',(-40.9882784321884,-14.9908026205824,
15.));
#24486=CARTESIAN_POINT('Ctrl Pts',(-40.8863921801,-15.0093553188655,15.));
#24487=CARTESIAN_POINT('Ctrl Pts',(-40.7845471608654,-15.0274064563211,
15.));
#24488=CARTESIAN_POINT('Ctrl Pts',(-40.6827452453667,-15.0449536183143,
15.));
#24489=CARTESIAN_POINT('Ctrl Pts',(-40.58098877043,-15.0619940893017,15.));
#24490=CARTESIAN_POINT('Ctrl Pts',(-40.4792803645352,-15.0785249502524,
15.));
#24491=CARTESIAN_POINT('Ctrl Pts',(-40.3776227809037,-15.0945431800723,
15.));
#24492=CARTESIAN_POINT('Ctrl Pts',(-40.2760187401821,-15.1100457495259,
15.));
#24493=CARTESIAN_POINT('Ctrl Pts',(-40.1744707357902,-15.1250297462408,
15.));
#24494=CARTESIAN_POINT('Ctrl Pts',(-40.0729810652204,-15.1394923361537,
15.));
#24495=CARTESIAN_POINT('Ctrl Pts',(-39.9715519332134,-15.1534306754871,
15.));
#24496=CARTESIAN_POINT('Ctrl Pts',(-39.8701855339908,-15.1668418393198,
15.));
#24497=CARTESIAN_POINT('Ctrl Pts',(-39.7688841338802,-15.1797227547561,
15.));
#24498=CARTESIAN_POINT('Ctrl Pts',(-39.6676501731673,-15.1920701163803,
15.));
#24499=CARTESIAN_POINT('Ctrl Pts',(-39.5664862602472,-15.2038804098649,
15.));
#24500=CARTESIAN_POINT('Ctrl Pts',(-39.4653951093947,-15.2151499908149,
15.));
#24501=CARTESIAN_POINT('Ctrl Pts',(-39.3643794927167,-15.2258751563069,
15.));
#24502=CARTESIAN_POINT('Ctrl Pts',(-39.2634421927888,-15.2360522089072,
15.));
#24503=CARTESIAN_POINT('Ctrl Pts',(-39.1625859371304,-15.2456775636447,
15.));
#24504=CARTESIAN_POINT('Ctrl Pts',(-39.061813415425,-15.2547476855825,15.));
#24505=CARTESIAN_POINT('Ctrl Pts',(-38.9611273555758,-15.2632589109473,
15.));
#24506=CARTESIAN_POINT('Ctrl Pts',(-38.860530586589,-15.2712072937639,15.));
#24507=CARTESIAN_POINT('Ctrl Pts',(-38.7600260961351,-15.2785884727112,
15.));
#24508=CARTESIAN_POINT('Ctrl Pts',(-38.659617115053,-15.2853974668211,15.));
#24509=CARTESIAN_POINT('Ctrl Pts',(-38.5593070891769,-15.2916287700102,
15.));
#24510=CARTESIAN_POINT('Ctrl Pts',(-38.4590995527814,-15.2972767037469,
15.));
#24511=CARTESIAN_POINT('Ctrl Pts',(-38.3589980188324,-15.3023357307483,
15.));
#24512=CARTESIAN_POINT('Ctrl Pts',(-38.2590058835965,-15.3068007250314,
15.));
#24513=CARTESIAN_POINT('Ctrl Pts',(-38.1591262705847,-15.310667421514,15.));
#24514=CARTESIAN_POINT('Ctrl Pts',(-38.0593621055415,-15.3139321941687,
15.));
#24515=CARTESIAN_POINT('Ctrl Pts',(-37.959716421934,-15.3165911656268,15.));
#24516=CARTESIAN_POINT('Ctrl Pts',(-37.8601926265378,-15.3186394335023,
15.));
#24517=CARTESIAN_POINT('Ctrl Pts',(-37.7607947318286,-15.320070396385,15.));
#24518=CARTESIAN_POINT('Ctrl Pts',(-37.6615277218027,-15.320874689078,15.));
#24519=CARTESIAN_POINT('Ctrl Pts',(-37.562397408596,-15.3210406145546,15.));
#24520=CARTESIAN_POINT('Ctrl Pts',(-37.4634097578665,-15.3205561366169,
15.));
#24521=CARTESIAN_POINT('Ctrl Pts',(-37.3645702997848,-15.3194106233801,
15.));
#24522=CARTESIAN_POINT('Ctrl Pts',(-37.2658836214694,-15.3175963510697,
15.));
#24523=CARTESIAN_POINT('Ctrl Pts',(-37.1673525354642,-15.3151109648809,
15.));
#24524=CARTESIAN_POINT('Ctrl Pts',(-37.0689784837457,-15.3119562971444,
15.));
#24525=CARTESIAN_POINT('Ctrl Pts',(-36.970763176802,-15.3081335446406,15.));
#24526=CARTESIAN_POINT('Ctrl Pts',(-36.8727100302512,-15.3036390436952,
15.));
#24527=CARTESIAN_POINT('Ctrl Pts',(-36.7748254044502,-15.2984606286737,
15.));
#24528=CARTESIAN_POINT('Ctrl Pts',(-36.6771206167756,-15.2925717100767,
15.));
#24529=CARTESIAN_POINT('Ctrl Pts',(-36.5796108931244,-15.2859343913094,
15.));
#24530=CARTESIAN_POINT('Ctrl Pts',(-36.4823116513289,-15.2785104654792,
15.));
#24531=CARTESIAN_POINT('Ctrl Pts',(-36.3852352131887,-15.2702711460937,
15.));
#24532=CARTESIAN_POINT('Ctrl Pts',(-36.2883880151607,-15.2612053303773,
15.));
#24533=CARTESIAN_POINT('Ctrl Pts',(-36.1917659216814,-15.2513334565427,
15.));
#24534=CARTESIAN_POINT('Ctrl Pts',(-36.095357546697,-15.240697754828,15.));
#24535=CARTESIAN_POINT('Ctrl Pts',(-35.9991531408727,-15.2293360946131,
15.));
#24536=CARTESIAN_POINT('Ctrl Pts',(-35.9031525499277,-15.2172585668056,
15.));
#24537=CARTESIAN_POINT('Ctrl Pts',(-35.8073720252878,-15.2044274601769,
15.));
#24538=CARTESIAN_POINT('Ctrl Pts',(-35.7118553943773,-15.1907243629658,
15.));
#24539=CARTESIAN_POINT('Ctrl Pts',(-35.6166644736253,-15.1759785763051,
15.));
#24540=CARTESIAN_POINT('Ctrl Pts',(-35.5218591529745,-15.1600260710383,
15.));
#24541=CARTESIAN_POINT('Ctrl Pts',(-35.4274792115856,-15.1427632633831,
15.));
#24542=CARTESIAN_POINT('Ctrl Pts',(-35.3335286891314,-15.1241934020681,
15.));
#24543=CARTESIAN_POINT('Ctrl Pts',(-35.2399506932815,-15.104500806927,15.));
#24544=CARTESIAN_POINT('Ctrl Pts',(-35.1466591020976,-15.08395927165,15.));
#24545=CARTESIAN_POINT('Ctrl Pts',(-35.0535882932913,-15.0627878528202,
15.));
#24546=CARTESIAN_POINT('Ctrl Pts',(-34.9607388363587,-15.041018569143,15.));
#24547=CARTESIAN_POINT('Ctrl Pts',(-34.8682205930809,-15.0183713484962,
15.));
#24548=CARTESIAN_POINT('Ctrl Pts',(-34.7763085406486,-14.9940927023321,
15.));
#24549=CARTESIAN_POINT('Ctrl Pts',(-34.6853717911268,-14.9671565602316,
15.));
#24550=CARTESIAN_POINT('Ctrl Pts',(-34.6137007885254,-14.9426481276593,
15.));
#24551=CARTESIAN_POINT('Ctrl Pts',(-34.5606858566713,-14.9222326355678,
15.));
#24552=CARTESIAN_POINT('Ctrl Pts',(-34.525687510388,-14.9076710061311,15.));
#24553=CARTESIAN_POINT('Ctrl Pts',(-34.5082745737944,-14.9001523628048,
15.));
#24554=CARTESIAN_POINT('',(-41.3962265246839,-14.9114864958881,0.));
#24555=CARTESIAN_POINT('Origin',(-1.07784724682657E-11,-3.50213800024364E-12,
0.));
#24556=CARTESIAN_POINT('',(-42.2550026135057,-12.2684454652018,0.));
#24557=CARTESIAN_POINT('Origin',(-1.07784724682657E-11,-3.50213800024364E-12,
0.));
#24558=CARTESIAN_POINT('',(-42.2550026135057,-12.2684454652018,15.));
#24559=CARTESIAN_POINT('Origin',(-1.07784724682657E-11,-3.50213800024364E-12,
15.));
#24560=CARTESIAN_POINT('',(-42.2550026135057,-12.2684454652018,0.));
#24561=CARTESIAN_POINT('Ctrl Pts',(-36.6758703925241,-8.2289783962506,0.));
#24562=CARTESIAN_POINT('Ctrl Pts',(-36.6758703925241,-8.2289783962506,18.));
#24563=CARTESIAN_POINT('Ctrl Pts',(-36.6943771018148,-8.23313075335376,
0.));
#24564=CARTESIAN_POINT('Ctrl Pts',(-36.6943771018148,-8.23313075335376,
18.));
#24565=CARTESIAN_POINT('Ctrl Pts',(-36.7312504697652,-8.24192165947367,
0.));
#24566=CARTESIAN_POINT('Ctrl Pts',(-36.7312504697652,-8.24192165947367,
18.));
#24567=CARTESIAN_POINT('Ctrl Pts',(-36.7861403757604,-8.2565665745182,0.));
#24568=CARTESIAN_POINT('Ctrl Pts',(-36.7861403757604,-8.2565665745182,18.));
#24569=CARTESIAN_POINT('Ctrl Pts',(-36.8585291300917,-8.27886599440784,
0.));
#24570=CARTESIAN_POINT('Ctrl Pts',(-36.8585291300917,-8.27886599440784,
18.));
#24571=CARTESIAN_POINT('Ctrl Pts',(-36.9479311729484,-8.31052547794591,
0.));
#24572=CARTESIAN_POINT('Ctrl Pts',(-36.9479311729484,-8.31052547794591,
18.));
#24573=CARTESIAN_POINT('Ctrl Pts',(-37.0365602155148,-8.34490818952639,
0.));
#24574=CARTESIAN_POINT('Ctrl Pts',(-37.0365602155148,-8.34490818952639,
18.));
#24575=CARTESIAN_POINT('Ctrl Pts',(-37.1247207489179,-8.38096706211447,
0.));
#24576=CARTESIAN_POINT('Ctrl Pts',(-37.1247207489179,-8.38096706211447,
18.));
#24577=CARTESIAN_POINT('Ctrl Pts',(-37.2126332013933,-8.41793088313259,
0.));
#24578=CARTESIAN_POINT('Ctrl Pts',(-37.2126332013933,-8.41793088313259,
18.));
#24579=CARTESIAN_POINT('Ctrl Pts',(-37.3003733151561,-8.45550849433959,
0.));
#24580=CARTESIAN_POINT('Ctrl Pts',(-37.3003733151561,-8.45550849433959,
18.));
#24581=CARTESIAN_POINT('Ctrl Pts',(-37.3879218093514,-8.49372546467075,
0.));
#24582=CARTESIAN_POINT('Ctrl Pts',(-37.3879218093514,-8.49372546467075,
18.));
#24583=CARTESIAN_POINT('Ctrl Pts',(-37.4752030152968,-8.53279758643783,
0.));
#24584=CARTESIAN_POINT('Ctrl Pts',(-37.4752030152968,-8.53279758643783,
18.));
#24585=CARTESIAN_POINT('Ctrl Pts',(-37.5621256752108,-8.57299698459465,
0.));
#24586=CARTESIAN_POINT('Ctrl Pts',(-37.5621256752108,-8.57299698459465,
18.));
#24587=CARTESIAN_POINT('Ctrl Pts',(-37.6486274754754,-8.61450621749154,
0.));
#24588=CARTESIAN_POINT('Ctrl Pts',(-37.6486274754754,-8.61450621749154,
18.));
#24589=CARTESIAN_POINT('Ctrl Pts',(-37.7347032383719,-8.65732553894524,
0.));
#24590=CARTESIAN_POINT('Ctrl Pts',(-37.7347032383719,-8.65732553894524,
18.));
#24591=CARTESIAN_POINT('Ctrl Pts',(-37.8203816669031,-8.70134776631143,
0.));
#24592=CARTESIAN_POINT('Ctrl Pts',(-37.8203816669031,-8.70134776631143,
18.));
#24593=CARTESIAN_POINT('Ctrl Pts',(-37.9057107230066,-8.74640499479002,
0.));
#24594=CARTESIAN_POINT('Ctrl Pts',(-37.9057107230066,-8.74640499479002,
18.));
#24595=CARTESIAN_POINT('Ctrl Pts',(-37.9907407304174,-8.79232279131091,
0.));
#24596=CARTESIAN_POINT('Ctrl Pts',(-37.9907407304174,-8.79232279131091,
18.));
#24597=CARTESIAN_POINT('Ctrl Pts',(-38.0755058326913,-8.83897959763348,
0.));
#24598=CARTESIAN_POINT('Ctrl Pts',(-38.0755058326913,-8.83897959763348,
18.));
#24599=CARTESIAN_POINT('Ctrl Pts',(-38.1600150482528,-8.88633535238434,
0.));
#24600=CARTESIAN_POINT('Ctrl Pts',(-38.1600150482528,-8.88633535238434,
18.));
#24601=CARTESIAN_POINT('Ctrl Pts',(-38.2442625706309,-8.93439830996338,
0.));
#24602=CARTESIAN_POINT('Ctrl Pts',(-38.2442625706309,-8.93439830996338,
18.));
#24603=CARTESIAN_POINT('Ctrl Pts',(-38.3282340281403,-8.98320483785759,
0.));
#24604=CARTESIAN_POINT('Ctrl Pts',(-38.3282340281403,-8.98320483785759,
18.));
#24605=CARTESIAN_POINT('Ctrl Pts',(-38.4119138099805,-9.0327957936019,0.));
#24606=CARTESIAN_POINT('Ctrl Pts',(-38.4119138099805,-9.0327957936019,18.));
#24607=CARTESIAN_POINT('Ctrl Pts',(-38.4952932486131,-9.08319014288085,
0.));
#24608=CARTESIAN_POINT('Ctrl Pts',(-38.4952932486131,-9.08319014288085,
18.));
#24609=CARTESIAN_POINT('Ctrl Pts',(-38.5783736628826,-9.13437512010585,
0.));
#24610=CARTESIAN_POINT('Ctrl Pts',(-38.5783736628826,-9.13437512010585,
18.));
#24611=CARTESIAN_POINT('Ctrl Pts',(-38.6611620045193,-9.18632019394329,
0.));
#24612=CARTESIAN_POINT('Ctrl Pts',(-38.6611620045193,-9.18632019394329,
18.));
#24613=CARTESIAN_POINT('Ctrl Pts',(-38.7436682576832,-9.23898539199331,
0.));
#24614=CARTESIAN_POINT('Ctrl Pts',(-38.7436682576832,-9.23898539199331,
18.));
#24615=CARTESIAN_POINT('Ctrl Pts',(-38.8259023794241,-9.29233110570902,
0.));
#24616=CARTESIAN_POINT('Ctrl Pts',(-38.8259023794241,-9.29233110570902,
18.));
#24617=CARTESIAN_POINT('Ctrl Pts',(-38.9078708427078,-9.34632917154636,
0.));
#24618=CARTESIAN_POINT('Ctrl Pts',(-38.9078708427078,-9.34632917154636,
18.));
#24619=CARTESIAN_POINT('Ctrl Pts',(-38.9895756526779,-9.40096600877643,
0.));
#24620=CARTESIAN_POINT('Ctrl Pts',(-38.9895756526779,-9.40096600877643,
18.));
#24621=CARTESIAN_POINT('Ctrl Pts',(-39.0710161994951,-9.45623664577431,
0.));
#24622=CARTESIAN_POINT('Ctrl Pts',(-39.0710161994951,-9.45623664577431,
18.));
#24623=CARTESIAN_POINT('Ctrl Pts',(-39.1521903958955,-9.5121410453562,0.));
#24624=CARTESIAN_POINT('Ctrl Pts',(-39.1521903958955,-9.5121410453562,18.));
#24625=CARTESIAN_POINT('Ctrl Pts',(-39.2330959982788,-9.56867984233622,
0.));
#24626=CARTESIAN_POINT('Ctrl Pts',(-39.2330959982788,-9.56867984233622,
18.));
#24627=CARTESIAN_POINT('Ctrl Pts',(-39.3137321153686,-9.62584947846543,
0.));
#24628=CARTESIAN_POINT('Ctrl Pts',(-39.3137321153686,-9.62584947846543,
18.));
#24629=CARTESIAN_POINT('Ctrl Pts',(-39.3940995760289,-9.68364100883826,
0.));
#24630=CARTESIAN_POINT('Ctrl Pts',(-39.3940995760289,-9.68364100883826,
18.));
#24631=CARTESIAN_POINT('Ctrl Pts',(-39.4742001555227,-9.74204258152662,
0.));
#24632=CARTESIAN_POINT('Ctrl Pts',(-39.4742001555227,-9.74204258152662,
18.));
#24633=CARTESIAN_POINT('Ctrl Pts',(-39.5540361022309,-9.80104095251613,
0.));
#24634=CARTESIAN_POINT('Ctrl Pts',(-39.5540361022309,-9.80104095251613,
18.));
#24635=CARTESIAN_POINT('Ctrl Pts',(-39.6336095893767,-9.86062324242559,
0.));
#24636=CARTESIAN_POINT('Ctrl Pts',(-39.6336095893767,-9.86062324242559,
18.));
#24637=CARTESIAN_POINT('Ctrl Pts',(-39.712922089547,-9.92077894513191,0.));
#24638=CARTESIAN_POINT('Ctrl Pts',(-39.712922089547,-9.92077894513191,18.));
#24639=CARTESIAN_POINT('Ctrl Pts',(-39.7919742367922,-9.98150036150822,
0.));
#24640=CARTESIAN_POINT('Ctrl Pts',(-39.7919742367922,-9.98150036150822,
18.));
#24641=CARTESIAN_POINT('Ctrl Pts',(-39.8707661565233,-10.0427815229883,
0.));
#24642=CARTESIAN_POINT('Ctrl Pts',(-39.8707661565233,-10.0427815229883,
18.));
#24643=CARTESIAN_POINT('Ctrl Pts',(-39.9492976736738,-10.1046175096878,
0.));
#24644=CARTESIAN_POINT('Ctrl Pts',(-39.9492976736738,-10.1046175096878,
18.));
#24645=CARTESIAN_POINT('Ctrl Pts',(-40.0275685525923,-10.1670036683795,
0.));
#24646=CARTESIAN_POINT('Ctrl Pts',(-40.0275685525923,-10.1670036683795,
18.));
#24647=CARTESIAN_POINT('Ctrl Pts',(-40.1055787732578,-10.2299347125857,
0.));
#24648=CARTESIAN_POINT('Ctrl Pts',(-40.1055787732578,-10.2299347125857,
18.));
#24649=CARTESIAN_POINT('Ctrl Pts',(-40.1833286010098,-10.2934044990237,
0.));
#24650=CARTESIAN_POINT('Ctrl Pts',(-40.1833286010098,-10.2934044990237,
18.));
#24651=CARTESIAN_POINT('Ctrl Pts',(-40.2608184485326,-10.3574064830678,
0.));
#24652=CARTESIAN_POINT('Ctrl Pts',(-40.2608184485326,-10.3574064830678,
18.));
#24653=CARTESIAN_POINT('Ctrl Pts',(-40.3380487942952,-10.421933993295,0.));
#24654=CARTESIAN_POINT('Ctrl Pts',(-40.3380487942952,-10.421933993295,18.));
#24655=CARTESIAN_POINT('Ctrl Pts',(-40.4150200869536,-10.48698054978,0.));
#24656=CARTESIAN_POINT('Ctrl Pts',(-40.4150200869536,-10.48698054978,18.));
#24657=CARTESIAN_POINT('Ctrl Pts',(-40.4917326404439,-10.5525402237951,
0.));
#24658=CARTESIAN_POINT('Ctrl Pts',(-40.4917326404439,-10.5525402237951,
18.));
#24659=CARTESIAN_POINT('Ctrl Pts',(-40.5681866012103,-10.618607730849,0.));
#24660=CARTESIAN_POINT('Ctrl Pts',(-40.5681866012103,-10.618607730849,18.));
#24661=CARTESIAN_POINT('Ctrl Pts',(-40.6443819999244,-10.6851782157325,
0.));
#24662=CARTESIAN_POINT('Ctrl Pts',(-40.6443819999244,-10.6851782157325,
18.));
#24663=CARTESIAN_POINT('Ctrl Pts',(-40.7203187831783,-10.7522471109694,
0.));
#24664=CARTESIAN_POINT('Ctrl Pts',(-40.7203187831783,-10.7522471109694,
18.));
#24665=CARTESIAN_POINT('Ctrl Pts',(-40.7959968527561,-10.8198099757795,
0.));
#24666=CARTESIAN_POINT('Ctrl Pts',(-40.7959968527561,-10.8198099757795,
18.));
#24667=CARTESIAN_POINT('Ctrl Pts',(-40.8714161092412,-10.8878623066646,
0.));
#24668=CARTESIAN_POINT('Ctrl Pts',(-40.8714161092412,-10.8878623066646,
18.));
#24669=CARTESIAN_POINT('Ctrl Pts',(-40.9465764747798,-10.956399476781,0.));
#24670=CARTESIAN_POINT('Ctrl Pts',(-40.9465764747798,-10.956399476781,18.));
#24671=CARTESIAN_POINT('Ctrl Pts',(-41.0214778832142,-11.0254168609972,
0.));
#24672=CARTESIAN_POINT('Ctrl Pts',(-41.0214778832142,-11.0254168609972,
18.));
#24673=CARTESIAN_POINT('Ctrl Pts',(-41.0961202807715,-11.0949099155251,
0.));
#24674=CARTESIAN_POINT('Ctrl Pts',(-41.0961202807715,-11.0949099155251,
18.));
#24675=CARTESIAN_POINT('Ctrl Pts',(-41.1705036228854,-11.1648742640378,
0.));
#24676=CARTESIAN_POINT('Ctrl Pts',(-41.1705036228854,-11.1648742640378,
18.));
#24677=CARTESIAN_POINT('Ctrl Pts',(-41.2446278781981,-11.2353057980338,
0.));
#24678=CARTESIAN_POINT('Ctrl Pts',(-41.2446278781981,-11.2353057980338,
18.));
#24679=CARTESIAN_POINT('Ctrl Pts',(-41.3184930194148,-11.3062006993745,
0.));
#24680=CARTESIAN_POINT('Ctrl Pts',(-41.3184930194148,-11.3062006993745,
18.));
#24681=CARTESIAN_POINT('Ctrl Pts',(-41.3920989905986,-11.3775553120176,
0.));
#24682=CARTESIAN_POINT('Ctrl Pts',(-41.3920989905986,-11.3775553120176,
18.));
#24683=CARTESIAN_POINT('Ctrl Pts',(-41.4654456796071,-11.4493660393849,
0.));
#24684=CARTESIAN_POINT('Ctrl Pts',(-41.4654456796071,-11.4493660393849,
18.));
#24685=CARTESIAN_POINT('Ctrl Pts',(-41.5385328935506,-11.5216292382388,
0.));
#24686=CARTESIAN_POINT('Ctrl Pts',(-41.5385328935506,-11.5216292382388,
18.));
#24687=CARTESIAN_POINT('Ctrl Pts',(-41.6113603270596,-11.5943410868252,
0.));
#24688=CARTESIAN_POINT('Ctrl Pts',(-41.6113603270596,-11.5943410868252,
18.));
#24689=CARTESIAN_POINT('Ctrl Pts',(-41.6839275596248,-11.6674975352851,
0.));
#24690=CARTESIAN_POINT('Ctrl Pts',(-41.6839275596248,-11.6674975352851,
18.));
#24691=CARTESIAN_POINT('Ctrl Pts',(-41.7562341395977,-11.7410945211992,
0.));
#24692=CARTESIAN_POINT('Ctrl Pts',(-41.7562341395977,-11.7410945211992,
18.));
#24693=CARTESIAN_POINT('Ctrl Pts',(-41.8282796562569,-11.81512813804,0.));
#24694=CARTESIAN_POINT('Ctrl Pts',(-41.8282796562569,-11.81512813804,18.));
#24695=CARTESIAN_POINT('Ctrl Pts',(-41.9000638152266,-11.8895948153349,
0.));
#24696=CARTESIAN_POINT('Ctrl Pts',(-41.9000638152266,-11.8895948153349,
18.));
#24697=CARTESIAN_POINT('Ctrl Pts',(-41.9715865222182,-11.9644914999263,
0.));
#24698=CARTESIAN_POINT('Ctrl Pts',(-41.9715865222182,-11.9644914999263,
18.));
#24699=CARTESIAN_POINT('Ctrl Pts',(-42.0428479428228,-12.0398158079102,
0.));
#24700=CARTESIAN_POINT('Ctrl Pts',(-42.0428479428228,-12.0398158079102,
18.));
#24701=CARTESIAN_POINT('Ctrl Pts',(-42.1138483839101,-12.1155659644537,
0.));
#24702=CARTESIAN_POINT('Ctrl Pts',(-42.1138483839101,-12.1155659644537,
18.));
#24703=CARTESIAN_POINT('Ctrl Pts',(-42.1704402333854,-12.1765058047069,
0.));
#24704=CARTESIAN_POINT('Ctrl Pts',(-42.1704402333854,-12.1765058047069,
18.));
#24705=CARTESIAN_POINT('Ctrl Pts',(-42.2127669677092,-12.2224014666679,
0.));
#24706=CARTESIAN_POINT('Ctrl Pts',(-42.2127669677092,-12.2224014666679,
18.));
#24707=CARTESIAN_POINT('Ctrl Pts',(-42.2409327400055,-12.2530833383985,
0.));
#24708=CARTESIAN_POINT('Ctrl Pts',(-42.2409327400055,-12.2530833383985,
18.));
#24709=CARTESIAN_POINT('Ctrl Pts',(-42.2550026135057,-12.2684454652018,
0.));
#24710=CARTESIAN_POINT('Ctrl Pts',(-42.2550026135057,-12.2684454652018,
18.));
#24711=CARTESIAN_POINT('Ctrl Pts',(-36.6758703925241,-8.2289783962506,0.));
#24712=CARTESIAN_POINT('Ctrl Pts',(-36.6943771018148,-8.23313075335376,
0.));
#24713=CARTESIAN_POINT('Ctrl Pts',(-36.7312504697652,-8.24192165947367,
0.));
#24714=CARTESIAN_POINT('Ctrl Pts',(-36.7861403757604,-8.2565665745182,0.));
#24715=CARTESIAN_POINT('Ctrl Pts',(-36.8585291300917,-8.27886599440784,
0.));
#24716=CARTESIAN_POINT('Ctrl Pts',(-36.9479311729484,-8.31052547794591,
0.));
#24717=CARTESIAN_POINT('Ctrl Pts',(-37.0365602155148,-8.34490818952639,
0.));
#24718=CARTESIAN_POINT('Ctrl Pts',(-37.1247207489179,-8.38096706211447,
0.));
#24719=CARTESIAN_POINT('Ctrl Pts',(-37.2126332013933,-8.41793088313259,
0.));
#24720=CARTESIAN_POINT('Ctrl Pts',(-37.3003733151561,-8.45550849433959,
0.));
#24721=CARTESIAN_POINT('Ctrl Pts',(-37.3879218093514,-8.49372546467075,
0.));
#24722=CARTESIAN_POINT('Ctrl Pts',(-37.4752030152968,-8.53279758643783,
0.));
#24723=CARTESIAN_POINT('Ctrl Pts',(-37.5621256752108,-8.57299698459465,
0.));
#24724=CARTESIAN_POINT('Ctrl Pts',(-37.6486274754754,-8.61450621749154,
0.));
#24725=CARTESIAN_POINT('Ctrl Pts',(-37.7347032383719,-8.65732553894524,
0.));
#24726=CARTESIAN_POINT('Ctrl Pts',(-37.8203816669031,-8.70134776631143,
0.));
#24727=CARTESIAN_POINT('Ctrl Pts',(-37.9057107230066,-8.74640499479002,
0.));
#24728=CARTESIAN_POINT('Ctrl Pts',(-37.9907407304174,-8.79232279131091,
0.));
#24729=CARTESIAN_POINT('Ctrl Pts',(-38.0755058326913,-8.83897959763348,
0.));
#24730=CARTESIAN_POINT('Ctrl Pts',(-38.1600150482528,-8.88633535238434,
0.));
#24731=CARTESIAN_POINT('Ctrl Pts',(-38.2442625706309,-8.93439830996338,
0.));
#24732=CARTESIAN_POINT('Ctrl Pts',(-38.3282340281403,-8.98320483785759,
0.));
#24733=CARTESIAN_POINT('Ctrl Pts',(-38.4119138099805,-9.0327957936019,0.));
#24734=CARTESIAN_POINT('Ctrl Pts',(-38.4952932486131,-9.08319014288085,
0.));
#24735=CARTESIAN_POINT('Ctrl Pts',(-38.5783736628826,-9.13437512010585,
0.));
#24736=CARTESIAN_POINT('Ctrl Pts',(-38.6611620045193,-9.18632019394329,
0.));
#24737=CARTESIAN_POINT('Ctrl Pts',(-38.7436682576832,-9.23898539199331,
0.));
#24738=CARTESIAN_POINT('Ctrl Pts',(-38.8259023794241,-9.29233110570902,
0.));
#24739=CARTESIAN_POINT('Ctrl Pts',(-38.9078708427078,-9.34632917154636,
0.));
#24740=CARTESIAN_POINT('Ctrl Pts',(-38.9895756526779,-9.40096600877643,
0.));
#24741=CARTESIAN_POINT('Ctrl Pts',(-39.0710161994951,-9.45623664577431,
0.));
#24742=CARTESIAN_POINT('Ctrl Pts',(-39.1521903958955,-9.5121410453562,0.));
#24743=CARTESIAN_POINT('Ctrl Pts',(-39.2330959982788,-9.56867984233622,
0.));
#24744=CARTESIAN_POINT('Ctrl Pts',(-39.3137321153686,-9.62584947846543,
0.));
#24745=CARTESIAN_POINT('Ctrl Pts',(-39.3940995760289,-9.68364100883826,
0.));
#24746=CARTESIAN_POINT('Ctrl Pts',(-39.4742001555227,-9.74204258152662,
0.));
#24747=CARTESIAN_POINT('Ctrl Pts',(-39.5540361022309,-9.80104095251613,
0.));
#24748=CARTESIAN_POINT('Ctrl Pts',(-39.6336095893767,-9.86062324242559,
0.));
#24749=CARTESIAN_POINT('Ctrl Pts',(-39.712922089547,-9.92077894513191,0.));
#24750=CARTESIAN_POINT('Ctrl Pts',(-39.7919742367922,-9.98150036150822,
0.));
#24751=CARTESIAN_POINT('Ctrl Pts',(-39.8707661565233,-10.0427815229883,
0.));
#24752=CARTESIAN_POINT('Ctrl Pts',(-39.9492976736738,-10.1046175096878,
0.));
#24753=CARTESIAN_POINT('Ctrl Pts',(-40.0275685525923,-10.1670036683795,
0.));
#24754=CARTESIAN_POINT('Ctrl Pts',(-40.1055787732578,-10.2299347125857,
0.));
#24755=CARTESIAN_POINT('Ctrl Pts',(-40.1833286010098,-10.2934044990237,
0.));
#24756=CARTESIAN_POINT('Ctrl Pts',(-40.2608184485326,-10.3574064830678,
0.));
#24757=CARTESIAN_POINT('Ctrl Pts',(-40.3380487942952,-10.421933993295,0.));
#24758=CARTESIAN_POINT('Ctrl Pts',(-40.4150200869536,-10.48698054978,0.));
#24759=CARTESIAN_POINT('Ctrl Pts',(-40.4917326404439,-10.5525402237951,
0.));
#24760=CARTESIAN_POINT('Ctrl Pts',(-40.5681866012103,-10.618607730849,0.));
#24761=CARTESIAN_POINT('Ctrl Pts',(-40.6443819999244,-10.6851782157325,
0.));
#24762=CARTESIAN_POINT('Ctrl Pts',(-40.7203187831783,-10.7522471109694,
0.));
#24763=CARTESIAN_POINT('Ctrl Pts',(-40.7959968527561,-10.8198099757795,
0.));
#24764=CARTESIAN_POINT('Ctrl Pts',(-40.8714161092412,-10.8878623066646,
0.));
#24765=CARTESIAN_POINT('Ctrl Pts',(-40.9465764747798,-10.956399476781,0.));
#24766=CARTESIAN_POINT('Ctrl Pts',(-41.0214778832142,-11.0254168609972,
0.));
#24767=CARTESIAN_POINT('Ctrl Pts',(-41.0961202807715,-11.0949099155251,
0.));
#24768=CARTESIAN_POINT('Ctrl Pts',(-41.1705036228854,-11.1648742640378,
0.));
#24769=CARTESIAN_POINT('Ctrl Pts',(-41.2446278781981,-11.2353057980338,
0.));
#24770=CARTESIAN_POINT('Ctrl Pts',(-41.3184930194148,-11.3062006993745,
0.));
#24771=CARTESIAN_POINT('Ctrl Pts',(-41.3920989905986,-11.3775553120176,
0.));
#24772=CARTESIAN_POINT('Ctrl Pts',(-41.4654456796071,-11.4493660393849,
0.));
#24773=CARTESIAN_POINT('Ctrl Pts',(-41.5385328935506,-11.5216292382388,
0.));
#24774=CARTESIAN_POINT('Ctrl Pts',(-41.6113603270596,-11.5943410868252,
0.));
#24775=CARTESIAN_POINT('Ctrl Pts',(-41.6839275596248,-11.6674975352851,
0.));
#24776=CARTESIAN_POINT('Ctrl Pts',(-41.7562341395977,-11.7410945211992,
0.));
#24777=CARTESIAN_POINT('Ctrl Pts',(-41.8282796562569,-11.81512813804,0.));
#24778=CARTESIAN_POINT('Ctrl Pts',(-41.9000638152266,-11.8895948153349,
0.));
#24779=CARTESIAN_POINT('Ctrl Pts',(-41.9715865222182,-11.9644914999263,
0.));
#24780=CARTESIAN_POINT('Ctrl Pts',(-42.0571002269437,-12.054880669507,0.));
#24781=CARTESIAN_POINT('Ctrl Pts',(-42.1280354231517,-12.1307372881904,
0.));
#24782=CARTESIAN_POINT('Ctrl Pts',(-42.18457517013,-12.1917619768791,0.));
#24783=CARTESIAN_POINT('Ctrl Pts',(-42.2268628664988,-12.2377212115623,
0.));
#24784=CARTESIAN_POINT('Ctrl Pts',(-42.2550026135057,-12.2684454652018,
0.));
#24785=CARTESIAN_POINT('Ctrl Pts',(-36.6758703925241,-8.2289783962506,15.));
#24786=CARTESIAN_POINT('Ctrl Pts',(-36.6943771018148,-8.23313075335376,
15.));
#24787=CARTESIAN_POINT('Ctrl Pts',(-36.7312504697652,-8.24192165947367,
15.));
#24788=CARTESIAN_POINT('Ctrl Pts',(-36.7861403757604,-8.2565665745182,15.));
#24789=CARTESIAN_POINT('Ctrl Pts',(-36.8585291300917,-8.27886599440784,
15.));
#24790=CARTESIAN_POINT('Ctrl Pts',(-36.9479311729484,-8.31052547794591,
15.));
#24791=CARTESIAN_POINT('Ctrl Pts',(-37.0365602155148,-8.34490818952639,
15.));
#24792=CARTESIAN_POINT('Ctrl Pts',(-37.1247207489179,-8.38096706211447,
15.));
#24793=CARTESIAN_POINT('Ctrl Pts',(-37.2126332013933,-8.41793088313259,
15.));
#24794=CARTESIAN_POINT('Ctrl Pts',(-37.3003733151561,-8.45550849433959,
15.));
#24795=CARTESIAN_POINT('Ctrl Pts',(-37.3879218093514,-8.49372546467075,
15.));
#24796=CARTESIAN_POINT('Ctrl Pts',(-37.4752030152968,-8.53279758643783,
15.));
#24797=CARTESIAN_POINT('Ctrl Pts',(-37.5621256752108,-8.57299698459465,
15.));
#24798=CARTESIAN_POINT('Ctrl Pts',(-37.6486274754754,-8.61450621749154,
15.));
#24799=CARTESIAN_POINT('Ctrl Pts',(-37.7347032383719,-8.65732553894524,
15.));
#24800=CARTESIAN_POINT('Ctrl Pts',(-37.8203816669031,-8.70134776631143,
15.));
#24801=CARTESIAN_POINT('Ctrl Pts',(-37.9057107230066,-8.74640499479002,
15.));
#24802=CARTESIAN_POINT('Ctrl Pts',(-37.9907407304174,-8.79232279131091,
15.));
#24803=CARTESIAN_POINT('Ctrl Pts',(-38.0755058326913,-8.83897959763348,
15.));
#24804=CARTESIAN_POINT('Ctrl Pts',(-38.1600150482528,-8.88633535238434,
15.));
#24805=CARTESIAN_POINT('Ctrl Pts',(-38.2442625706309,-8.93439830996338,
15.));
#24806=CARTESIAN_POINT('Ctrl Pts',(-38.3282340281403,-8.98320483785759,
15.));
#24807=CARTESIAN_POINT('Ctrl Pts',(-38.4119138099805,-9.0327957936019,15.));
#24808=CARTESIAN_POINT('Ctrl Pts',(-38.4952932486131,-9.08319014288085,
15.));
#24809=CARTESIAN_POINT('Ctrl Pts',(-38.5783736628826,-9.13437512010585,
15.));
#24810=CARTESIAN_POINT('Ctrl Pts',(-38.6611620045193,-9.18632019394329,
15.));
#24811=CARTESIAN_POINT('Ctrl Pts',(-38.7436682576832,-9.23898539199331,
15.));
#24812=CARTESIAN_POINT('Ctrl Pts',(-38.8259023794241,-9.29233110570902,
15.));
#24813=CARTESIAN_POINT('Ctrl Pts',(-38.9078708427078,-9.34632917154636,
15.));
#24814=CARTESIAN_POINT('Ctrl Pts',(-38.9895756526779,-9.40096600877643,
15.));
#24815=CARTESIAN_POINT('Ctrl Pts',(-39.0710161994951,-9.45623664577431,
15.));
#24816=CARTESIAN_POINT('Ctrl Pts',(-39.1521903958955,-9.5121410453562,15.));
#24817=CARTESIAN_POINT('Ctrl Pts',(-39.2330959982788,-9.56867984233622,
15.));
#24818=CARTESIAN_POINT('Ctrl Pts',(-39.3137321153686,-9.62584947846543,
15.));
#24819=CARTESIAN_POINT('Ctrl Pts',(-39.3940995760289,-9.68364100883826,
15.));
#24820=CARTESIAN_POINT('Ctrl Pts',(-39.4742001555227,-9.74204258152662,
15.));
#24821=CARTESIAN_POINT('Ctrl Pts',(-39.5540361022309,-9.80104095251613,
15.));
#24822=CARTESIAN_POINT('Ctrl Pts',(-39.6336095893767,-9.86062324242559,
15.));
#24823=CARTESIAN_POINT('Ctrl Pts',(-39.712922089547,-9.92077894513191,15.));
#24824=CARTESIAN_POINT('Ctrl Pts',(-39.7919742367922,-9.98150036150822,
15.));
#24825=CARTESIAN_POINT('Ctrl Pts',(-39.8707661565233,-10.0427815229883,
15.));
#24826=CARTESIAN_POINT('Ctrl Pts',(-39.9492976736738,-10.1046175096878,
15.));
#24827=CARTESIAN_POINT('Ctrl Pts',(-40.0275685525923,-10.1670036683795,
15.));
#24828=CARTESIAN_POINT('Ctrl Pts',(-40.1055787732578,-10.2299347125857,
15.));
#24829=CARTESIAN_POINT('Ctrl Pts',(-40.1833286010098,-10.2934044990237,
15.));
#24830=CARTESIAN_POINT('Ctrl Pts',(-40.2608184485326,-10.3574064830678,
15.));
#24831=CARTESIAN_POINT('Ctrl Pts',(-40.3380487942952,-10.421933993295,15.));
#24832=CARTESIAN_POINT('Ctrl Pts',(-40.4150200869536,-10.48698054978,15.));
#24833=CARTESIAN_POINT('Ctrl Pts',(-40.4917326404439,-10.5525402237951,
15.));
#24834=CARTESIAN_POINT('Ctrl Pts',(-40.5681866012103,-10.618607730849,15.));
#24835=CARTESIAN_POINT('Ctrl Pts',(-40.6443819999244,-10.6851782157325,
15.));
#24836=CARTESIAN_POINT('Ctrl Pts',(-40.7203187831783,-10.7522471109694,
15.));
#24837=CARTESIAN_POINT('Ctrl Pts',(-40.7959968527561,-10.8198099757795,
15.));
#24838=CARTESIAN_POINT('Ctrl Pts',(-40.8714161092412,-10.8878623066646,
15.));
#24839=CARTESIAN_POINT('Ctrl Pts',(-40.9465764747798,-10.956399476781,15.));
#24840=CARTESIAN_POINT('Ctrl Pts',(-41.0214778832142,-11.0254168609972,
15.));
#24841=CARTESIAN_POINT('Ctrl Pts',(-41.0961202807715,-11.0949099155251,
15.));
#24842=CARTESIAN_POINT('Ctrl Pts',(-41.1705036228854,-11.1648742640378,
15.));
#24843=CARTESIAN_POINT('Ctrl Pts',(-41.2446278781981,-11.2353057980338,
15.));
#24844=CARTESIAN_POINT('Ctrl Pts',(-41.3184930194148,-11.3062006993745,
15.));
#24845=CARTESIAN_POINT('Ctrl Pts',(-41.3920989905986,-11.3775553120176,
15.));
#24846=CARTESIAN_POINT('Ctrl Pts',(-41.4654456796071,-11.4493660393849,
15.));
#24847=CARTESIAN_POINT('Ctrl Pts',(-41.5385328935506,-11.5216292382388,
15.));
#24848=CARTESIAN_POINT('Ctrl Pts',(-41.6113603270596,-11.5943410868252,
15.));
#24849=CARTESIAN_POINT('Ctrl Pts',(-41.6839275596248,-11.6674975352851,
15.));
#24850=CARTESIAN_POINT('Ctrl Pts',(-41.7562341395977,-11.7410945211992,
15.));
#24851=CARTESIAN_POINT('Ctrl Pts',(-41.8282796562569,-11.81512813804,15.));
#24852=CARTESIAN_POINT('Ctrl Pts',(-41.9000638152266,-11.8895948153349,
15.));
#24853=CARTESIAN_POINT('Ctrl Pts',(-41.9715865222182,-11.9644914999263,
15.));
#24854=CARTESIAN_POINT('Ctrl Pts',(-42.0571002269437,-12.054880669507,15.));
#24855=CARTESIAN_POINT('Ctrl Pts',(-42.1280354231517,-12.1307372881904,
15.));
#24856=CARTESIAN_POINT('Ctrl Pts',(-42.18457517013,-12.1917619768791,15.));
#24857=CARTESIAN_POINT('Ctrl Pts',(-42.2268628664988,-12.2377212115623,
15.));
#24858=CARTESIAN_POINT('Ctrl Pts',(-42.2550026135057,-12.2684454652018,
15.));
#24859=CARTESIAN_POINT('Ctrl Pts',(-43.9780537249529,-1.38952890043916,
0.));
#24860=CARTESIAN_POINT('Ctrl Pts',(-43.9780537249529,-1.38952890043916,
18.));
#24861=CARTESIAN_POINT('Ctrl Pts',(-43.9599253218252,-1.39979132121931,
0.));
#24862=CARTESIAN_POINT('Ctrl Pts',(-43.9599253218252,-1.39979132121931,
18.));
#24863=CARTESIAN_POINT('Ctrl Pts',(-43.9236568607623,-1.42026781296156,
0.));
#24864=CARTESIAN_POINT('Ctrl Pts',(-43.9236568607623,-1.42026781296156,
18.));
#24865=CARTESIAN_POINT('Ctrl Pts',(-43.8692192047561,-1.45083750111682,
0.));
#24866=CARTESIAN_POINT('Ctrl Pts',(-43.8692192047561,-1.45083750111682,
18.));
#24867=CARTESIAN_POINT('Ctrl Pts',(-43.7965657112708,-1.49130689006066,
0.));
#24868=CARTESIAN_POINT('Ctrl Pts',(-43.7965657112708,-1.49130689006066,
18.));
#24869=CARTESIAN_POINT('Ctrl Pts',(-43.7056321934163,-1.54140922714764,
0.));
#24870=CARTESIAN_POINT('Ctrl Pts',(-43.7056321934163,-1.54140922714764,
18.));
#24871=CARTESIAN_POINT('Ctrl Pts',(-43.6145820637333,-1.59102591108103,
0.));
#24872=CARTESIAN_POINT('Ctrl Pts',(-43.6145820637333,-1.59102591108103,
18.));
#24873=CARTESIAN_POINT('Ctrl Pts',(-43.5234155788248,-1.64015515906648,
0.));
#24874=CARTESIAN_POINT('Ctrl Pts',(-43.5234155788248,-1.64015515906648,
18.));
#24875=CARTESIAN_POINT('Ctrl Pts',(-43.4321333178711,-1.68879465270608,
0.));
#24876=CARTESIAN_POINT('Ctrl Pts',(-43.4321333178711,-1.68879465270608,
18.));
#24877=CARTESIAN_POINT('Ctrl Pts',(-43.3407363140236,-1.73694151741123,
0.));
#24878=CARTESIAN_POINT('Ctrl Pts',(-43.3407363140236,-1.73694151741123,
18.));
#24879=CARTESIAN_POINT('Ctrl Pts',(-43.2492259505872,-1.78459244842769,
0.));
#24880=CARTESIAN_POINT('Ctrl Pts',(-43.2492259505872,-1.78459244842769,
18.));
#24881=CARTESIAN_POINT('Ctrl Pts',(-43.1576038253643,-1.83174385734711,
0.));
#24882=CARTESIAN_POINT('Ctrl Pts',(-43.1576038253643,-1.83174385734711,
18.));
#24883=CARTESIAN_POINT('Ctrl Pts',(-43.065871623255,-1.87839202014609,0.));
#24884=CARTESIAN_POINT('Ctrl Pts',(-43.065871623255,-1.87839202014609,18.));
#24885=CARTESIAN_POINT('Ctrl Pts',(-42.9740309956624,-1.92453321512435,
0.));
#24886=CARTESIAN_POINT('Ctrl Pts',(-42.9740309956624,-1.92453321512435,
18.));
#24887=CARTESIAN_POINT('Ctrl Pts',(-42.8820834139973,-1.97016390194216,
0.));
#24888=CARTESIAN_POINT('Ctrl Pts',(-42.8820834139973,-1.97016390194216,
18.));
#24889=CARTESIAN_POINT('Ctrl Pts',(-42.7900301875309,-2.01528067528089,
0.));
#24890=CARTESIAN_POINT('Ctrl Pts',(-42.7900301875309,-2.01528067528089,
18.));
#24891=CARTESIAN_POINT('Ctrl Pts',(-42.6978725343209,-2.05988014924519,
0.));
#24892=CARTESIAN_POINT('Ctrl Pts',(-42.6978725343209,-2.05988014924519,
18.));
#24893=CARTESIAN_POINT('Ctrl Pts',(-42.6056116373456,-2.1039588640177,0.));
#24894=CARTESIAN_POINT('Ctrl Pts',(-42.6056116373456,-2.1039588640177,18.));
#24895=CARTESIAN_POINT('Ctrl Pts',(-42.5132487024335,-2.14751319676745,
0.));
#24896=CARTESIAN_POINT('Ctrl Pts',(-42.5132487024335,-2.14751319676745,
18.));
#24897=CARTESIAN_POINT('Ctrl Pts',(-42.4207850290047,-2.19053924976737,
0.));
#24898=CARTESIAN_POINT('Ctrl Pts',(-42.4207850290047,-2.19053924976737,
18.));
#24899=CARTESIAN_POINT('Ctrl Pts',(-42.3282220118033,-2.23303287465499,
0.));
#24900=CARTESIAN_POINT('Ctrl Pts',(-42.3282220118033,-2.23303287465499,
18.));
#24901=CARTESIAN_POINT('Ctrl Pts',(-42.2355611060784,-2.27498976664774,
0.));
#24902=CARTESIAN_POINT('Ctrl Pts',(-42.2355611060784,-2.27498976664774,
18.));
#24903=CARTESIAN_POINT('Ctrl Pts',(-42.1428038039937,-2.31640554742808,
0.));
#24904=CARTESIAN_POINT('Ctrl Pts',(-42.1428038039937,-2.31640554742808,
18.));
#24905=CARTESIAN_POINT('Ctrl Pts',(-42.0499516093661,-2.35727584066429,
0.));
#24906=CARTESIAN_POINT('Ctrl Pts',(-42.0499516093661,-2.35727584066429,
18.));
#24907=CARTESIAN_POINT('Ctrl Pts',(-41.9570060084039,-2.39759639399648,
0.));
#24908=CARTESIAN_POINT('Ctrl Pts',(-41.9570060084039,-2.39759639399648,
18.));
#24909=CARTESIAN_POINT('Ctrl Pts',(-41.8639684667923,-2.437363014342,0.));
#24910=CARTESIAN_POINT('Ctrl Pts',(-41.8639684667923,-2.437363014342,18.));
#24911=CARTESIAN_POINT('Ctrl Pts',(-41.7708404467533,-2.47657137427693,
0.));
#24912=CARTESIAN_POINT('Ctrl Pts',(-41.7708404467533,-2.47657137427693,
18.));
#24913=CARTESIAN_POINT('Ctrl Pts',(-41.6776234194583,-2.51521684674477,
0.));
#24914=CARTESIAN_POINT('Ctrl Pts',(-41.6776234194583,-2.51521684674477,
18.));
#24915=CARTESIAN_POINT('Ctrl Pts',(-41.5843188786284,-2.55329436064184,
0.));
#24916=CARTESIAN_POINT('Ctrl Pts',(-41.5843188786284,-2.55329436064184,
18.));
#24917=CARTESIAN_POINT('Ctrl Pts',(-41.4909283577703,-2.59079818040171,
0.));
#24918=CARTESIAN_POINT('Ctrl Pts',(-41.4909283577703,-2.59079818040171,
18.));
#24919=CARTESIAN_POINT('Ctrl Pts',(-41.3974534325937,-2.62772200460656,
0.));
#24920=CARTESIAN_POINT('Ctrl Pts',(-41.3974534325937,-2.62772200460656,
18.));
#24921=CARTESIAN_POINT('Ctrl Pts',(-41.3038957096306,-2.66405934050118,
0.));
#24922=CARTESIAN_POINT('Ctrl Pts',(-41.3038957096306,-2.66405934050118,
18.));
#24923=CARTESIAN_POINT('Ctrl Pts',(-41.2102568187956,-2.69980383625015,
0.));
#24924=CARTESIAN_POINT('Ctrl Pts',(-41.2102568187956,-2.69980383625015,
18.));
#24925=CARTESIAN_POINT('Ctrl Pts',(-41.1165384061145,-2.73494956725005,
0.));
#24926=CARTESIAN_POINT('Ctrl Pts',(-41.1165384061145,-2.73494956725005,
18.));
#24927=CARTESIAN_POINT('Ctrl Pts',(-41.0227421242398,-2.76949151194863,
0.));
#24928=CARTESIAN_POINT('Ctrl Pts',(-41.0227421242398,-2.76949151194863,
18.));
#24929=CARTESIAN_POINT('Ctrl Pts',(-40.9288696352159,-2.80342531768405,
0.));
#24930=CARTESIAN_POINT('Ctrl Pts',(-40.9288696352159,-2.80342531768405,
18.));
#24931=CARTESIAN_POINT('Ctrl Pts',(-40.8349226258683,-2.83674635946679,
0.));
#24932=CARTESIAN_POINT('Ctrl Pts',(-40.8349226258683,-2.83674635946679,
18.));
#24933=CARTESIAN_POINT('Ctrl Pts',(-40.7409028213129,-2.86944892209897,
0.));
#24934=CARTESIAN_POINT('Ctrl Pts',(-40.7409028213129,-2.86944892209897,
18.));
#24935=CARTESIAN_POINT('Ctrl Pts',(-40.6468119976928,-2.90152548734342,
0.));
#24936=CARTESIAN_POINT('Ctrl Pts',(-40.6468119976928,-2.90152548734342,
18.));
#24937=CARTESIAN_POINT('Ctrl Pts',(-40.5526520010651,-2.93296560822893,
0.));
#24938=CARTESIAN_POINT('Ctrl Pts',(-40.5526520010651,-2.93296560822893,
18.));
#24939=CARTESIAN_POINT('Ctrl Pts',(-40.4584247445196,-2.96375636417322,
0.));
#24940=CARTESIAN_POINT('Ctrl Pts',(-40.4584247445196,-2.96375636417322,
18.));
#24941=CARTESIAN_POINT('Ctrl Pts',(-40.3641321823444,-2.99388446458219,
0.));
#24942=CARTESIAN_POINT('Ctrl Pts',(-40.3641321823444,-2.99388446458219,
18.));
#24943=CARTESIAN_POINT('Ctrl Pts',(-40.2697762886113,-3.02333808901595,
0.));
#24944=CARTESIAN_POINT('Ctrl Pts',(-40.2697762886113,-3.02333808901595,
18.));
#24945=CARTESIAN_POINT('Ctrl Pts',(-40.1753590391515,-3.0521084742307,0.));
#24946=CARTESIAN_POINT('Ctrl Pts',(-40.1753590391515,-3.0521084742307,18.));
#24947=CARTESIAN_POINT('Ctrl Pts',(-40.0808823811787,-3.08019251155015,
0.));
#24948=CARTESIAN_POINT('Ctrl Pts',(-40.0808823811787,-3.08019251155015,
18.));
#24949=CARTESIAN_POINT('Ctrl Pts',(-39.9863482523153,-3.10759149802907,
0.));
#24950=CARTESIAN_POINT('Ctrl Pts',(-39.9863482523153,-3.10759149802907,
18.));
#24951=CARTESIAN_POINT('Ctrl Pts',(-39.8917586491576,-3.13430604330355,
0.));
#24952=CARTESIAN_POINT('Ctrl Pts',(-39.8917586491576,-3.13430604330355,
18.));
#24953=CARTESIAN_POINT('Ctrl Pts',(-39.7971156880138,-3.16033160752803,
0.));
#24954=CARTESIAN_POINT('Ctrl Pts',(-39.7971156880138,-3.16033160752803,
18.));
#24955=CARTESIAN_POINT('Ctrl Pts',(-39.7024216585552,-3.18565465503835,
0.));
#24956=CARTESIAN_POINT('Ctrl Pts',(-39.7024216585552,-3.18565465503835,
18.));
#24957=CARTESIAN_POINT('Ctrl Pts',(-39.607679107639,-3.21024640045595,0.));
#24958=CARTESIAN_POINT('Ctrl Pts',(-39.607679107639,-3.21024640045595,18.));
#24959=CARTESIAN_POINT('Ctrl Pts',(-39.5128908052622,-3.23406609691661,
0.));
#24960=CARTESIAN_POINT('Ctrl Pts',(-39.5128908052622,-3.23406609691661,
18.));
#24961=CARTESIAN_POINT('Ctrl Pts',(-39.4180596080755,-3.25707264313388,
0.));
#24962=CARTESIAN_POINT('Ctrl Pts',(-39.4180596080755,-3.25707264313388,
18.));
#24963=CARTESIAN_POINT('Ctrl Pts',(-39.3231883392913,-3.27923485388117,
0.));
#24964=CARTESIAN_POINT('Ctrl Pts',(-39.3231883392913,-3.27923485388117,
18.));
#24965=CARTESIAN_POINT('Ctrl Pts',(-39.2282796893977,-3.30054018081687,
0.));
#24966=CARTESIAN_POINT('Ctrl Pts',(-39.2282796893977,-3.30054018081687,
18.));
#24967=CARTESIAN_POINT('Ctrl Pts',(-39.1333360409949,-3.32100933979557,
0.));
#24968=CARTESIAN_POINT('Ctrl Pts',(-39.1333360409949,-3.32100933979557,
18.));
#24969=CARTESIAN_POINT('Ctrl Pts',(-39.0383596151636,-3.34068601264472,
0.));
#24970=CARTESIAN_POINT('Ctrl Pts',(-39.0383596151636,-3.34068601264472,
18.));
#24971=CARTESIAN_POINT('Ctrl Pts',(-38.9433528420174,-3.3596092279948,0.));
#24972=CARTESIAN_POINT('Ctrl Pts',(-38.9433528420174,-3.3596092279948,18.));
#24973=CARTESIAN_POINT('Ctrl Pts',(-38.8483186930884,-3.37778863054482,
0.));
#24974=CARTESIAN_POINT('Ctrl Pts',(-38.8483186930884,-3.37778863054482,
18.));
#24975=CARTESIAN_POINT('Ctrl Pts',(-38.7532609709905,-3.39518333281818,
0.));
#24976=CARTESIAN_POINT('Ctrl Pts',(-38.7532609709905,-3.39518333281818,
18.));
#24977=CARTESIAN_POINT('Ctrl Pts',(-38.6581847668347,-3.411667175119,0.));
#24978=CARTESIAN_POINT('Ctrl Pts',(-38.6581847668347,-3.411667175119,18.));
#24979=CARTESIAN_POINT('Ctrl Pts',(-38.5630961226878,-3.42705871084996,
0.));
#24980=CARTESIAN_POINT('Ctrl Pts',(-38.5630961226878,-3.42705871084996,
18.));
#24981=CARTESIAN_POINT('Ctrl Pts',(-38.4680013094732,-3.44118343200303,
0.));
#24982=CARTESIAN_POINT('Ctrl Pts',(-38.4680013094732,-3.44118343200303,
18.));
#24983=CARTESIAN_POINT('Ctrl Pts',(-38.3729061502716,-3.45393053211022,
0.));
#24984=CARTESIAN_POINT('Ctrl Pts',(-38.3729061502716,-3.45393053211022,
18.));
#24985=CARTESIAN_POINT('Ctrl Pts',(-38.2778154909527,-3.46530185256872,
0.));
#24986=CARTESIAN_POINT('Ctrl Pts',(-38.2778154909527,-3.46530185256872,
18.));
#24987=CARTESIAN_POINT('Ctrl Pts',(-38.1827321816559,-3.47549027265411,
0.));
#24988=CARTESIAN_POINT('Ctrl Pts',(-38.1827321816559,-3.47549027265411,
18.));
#24989=CARTESIAN_POINT('Ctrl Pts',(-38.0876589224537,-3.48478279878233,
0.));
#24990=CARTESIAN_POINT('Ctrl Pts',(-38.0876589224537,-3.48478279878233,
18.));
#24991=CARTESIAN_POINT('Ctrl Pts',(-37.9926009950482,-3.49340804454645,
0.));
#24992=CARTESIAN_POINT('Ctrl Pts',(-37.9926009950482,-3.49340804454645,
18.));
#24993=CARTESIAN_POINT('Ctrl Pts',(-37.8975688353863,-3.50139628556083,
0.));
#24994=CARTESIAN_POINT('Ctrl Pts',(-37.8975688353863,-3.50139628556083,
18.));
#24995=CARTESIAN_POINT('Ctrl Pts',(-37.8025803811856,-3.50844720825128,
0.));
#24996=CARTESIAN_POINT('Ctrl Pts',(-37.8025803811856,-3.50844720825128,
18.));
#24997=CARTESIAN_POINT('Ctrl Pts',(-37.7076643105286,-3.51375922979957,
0.));
#24998=CARTESIAN_POINT('Ctrl Pts',(-37.7076643105286,-3.51375922979957,
18.));
#24999=CARTESIAN_POINT('Ctrl Pts',(-37.6128545966533,-3.51624243734645,
0.));
#25000=CARTESIAN_POINT('Ctrl Pts',(-37.6128545966533,-3.51624243734645,
18.));
#25001=CARTESIAN_POINT('Ctrl Pts',(-37.5371179004295,-3.51508109065209,
0.));
#25002=CARTESIAN_POINT('Ctrl Pts',(-37.5371179004295,-3.51508109065209,
18.));
#25003=CARTESIAN_POINT('Ctrl Pts',(-37.4803889700239,-3.51204731876361,
0.));
#25004=CARTESIAN_POINT('Ctrl Pts',(-37.4803889700239,-3.51204731876361,
18.));
#25005=CARTESIAN_POINT('Ctrl Pts',(-37.4426037737699,-3.50901346997657,
0.));
#25006=CARTESIAN_POINT('Ctrl Pts',(-37.4426037737699,-3.50901346997657,
18.));
#25007=CARTESIAN_POINT('Ctrl Pts',(-37.4237196983922,-3.50724370857673,
0.));
#25008=CARTESIAN_POINT('Ctrl Pts',(-37.4237196983922,-3.50724370857673,
18.));
#25009=CARTESIAN_POINT('',(-43.9780537249529,-1.38952890043929,0.));
#25010=CARTESIAN_POINT('Ctrl Pts',(-37.4237196983922,-3.50724370857673,
0.));
#25011=CARTESIAN_POINT('Ctrl Pts',(-37.4426037737699,-3.50901346997657,
0.));
#25012=CARTESIAN_POINT('Ctrl Pts',(-37.4803889700239,-3.51204731876361,
0.));
#25013=CARTESIAN_POINT('Ctrl Pts',(-37.5371179004295,-3.51508109065209,
0.));
#25014=CARTESIAN_POINT('Ctrl Pts',(-37.6128545966533,-3.51624243734645,
0.));
#25015=CARTESIAN_POINT('Ctrl Pts',(-37.7076643105286,-3.51375922979957,
0.));
#25016=CARTESIAN_POINT('Ctrl Pts',(-37.8025803811856,-3.50844720825128,
0.));
#25017=CARTESIAN_POINT('Ctrl Pts',(-37.8975688353863,-3.50139628556083,
0.));
#25018=CARTESIAN_POINT('Ctrl Pts',(-37.9926009950482,-3.49340804454645,
0.));
#25019=CARTESIAN_POINT('Ctrl Pts',(-38.0876589224537,-3.48478279878233,
0.));
#25020=CARTESIAN_POINT('Ctrl Pts',(-38.1827321816559,-3.47549027265411,
0.));
#25021=CARTESIAN_POINT('Ctrl Pts',(-38.2778154909527,-3.46530185256872,
0.));
#25022=CARTESIAN_POINT('Ctrl Pts',(-38.3729061502716,-3.45393053211022,
0.));
#25023=CARTESIAN_POINT('Ctrl Pts',(-38.4680013094732,-3.44118343200303,
0.));
#25024=CARTESIAN_POINT('Ctrl Pts',(-38.5630961226878,-3.42705871084996,
0.));
#25025=CARTESIAN_POINT('Ctrl Pts',(-38.6581847668347,-3.411667175119,0.));
#25026=CARTESIAN_POINT('Ctrl Pts',(-38.7532609709905,-3.39518333281818,
0.));
#25027=CARTESIAN_POINT('Ctrl Pts',(-38.8483186930884,-3.37778863054482,
0.));
#25028=CARTESIAN_POINT('Ctrl Pts',(-38.9433528420174,-3.3596092279948,0.));
#25029=CARTESIAN_POINT('Ctrl Pts',(-39.0383596151636,-3.34068601264472,
0.));
#25030=CARTESIAN_POINT('Ctrl Pts',(-39.1333360409949,-3.32100933979557,
0.));
#25031=CARTESIAN_POINT('Ctrl Pts',(-39.2282796893977,-3.30054018081687,
0.));
#25032=CARTESIAN_POINT('Ctrl Pts',(-39.3231883392913,-3.27923485388117,
0.));
#25033=CARTESIAN_POINT('Ctrl Pts',(-39.4180596080755,-3.25707264313388,
0.));
#25034=CARTESIAN_POINT('Ctrl Pts',(-39.5128908052622,-3.23406609691661,
0.));
#25035=CARTESIAN_POINT('Ctrl Pts',(-39.607679107639,-3.21024640045595,0.));
#25036=CARTESIAN_POINT('Ctrl Pts',(-39.7024216585552,-3.18565465503835,
0.));
#25037=CARTESIAN_POINT('Ctrl Pts',(-39.7971156880138,-3.16033160752803,
0.));
#25038=CARTESIAN_POINT('Ctrl Pts',(-39.8917586491576,-3.13430604330355,
0.));
#25039=CARTESIAN_POINT('Ctrl Pts',(-39.9863482523153,-3.10759149802907,
0.));
#25040=CARTESIAN_POINT('Ctrl Pts',(-40.0808823811787,-3.08019251155015,
0.));
#25041=CARTESIAN_POINT('Ctrl Pts',(-40.1753590391515,-3.0521084742307,0.));
#25042=CARTESIAN_POINT('Ctrl Pts',(-40.2697762886113,-3.02333808901595,
0.));
#25043=CARTESIAN_POINT('Ctrl Pts',(-40.3641321823444,-2.99388446458219,
0.));
#25044=CARTESIAN_POINT('Ctrl Pts',(-40.4584247445196,-2.96375636417322,
0.));
#25045=CARTESIAN_POINT('Ctrl Pts',(-40.5526520010651,-2.93296560822893,
0.));
#25046=CARTESIAN_POINT('Ctrl Pts',(-40.6468119976928,-2.90152548734342,
0.));
#25047=CARTESIAN_POINT('Ctrl Pts',(-40.7409028213129,-2.86944892209897,
0.));
#25048=CARTESIAN_POINT('Ctrl Pts',(-40.8349226258683,-2.83674635946679,
0.));
#25049=CARTESIAN_POINT('Ctrl Pts',(-40.9288696352159,-2.80342531768405,
0.));
#25050=CARTESIAN_POINT('Ctrl Pts',(-41.0227421242398,-2.76949151194863,
0.));
#25051=CARTESIAN_POINT('Ctrl Pts',(-41.1165384061145,-2.73494956725005,
0.));
#25052=CARTESIAN_POINT('Ctrl Pts',(-41.2102568187956,-2.69980383625015,
0.));
#25053=CARTESIAN_POINT('Ctrl Pts',(-41.3038957096306,-2.66405934050118,
0.));
#25054=CARTESIAN_POINT('Ctrl Pts',(-41.3974534325937,-2.62772200460656,
0.));
#25055=CARTESIAN_POINT('Ctrl Pts',(-41.4909283577703,-2.59079818040171,
0.));
#25056=CARTESIAN_POINT('Ctrl Pts',(-41.5843188786284,-2.55329436064184,
0.));
#25057=CARTESIAN_POINT('Ctrl Pts',(-41.6776234194583,-2.51521684674477,
0.));
#25058=CARTESIAN_POINT('Ctrl Pts',(-41.7708404467533,-2.47657137427693,
0.));
#25059=CARTESIAN_POINT('Ctrl Pts',(-41.8639684667923,-2.437363014342,0.));
#25060=CARTESIAN_POINT('Ctrl Pts',(-41.9570060084039,-2.39759639399648,
0.));
#25061=CARTESIAN_POINT('Ctrl Pts',(-42.0499516093661,-2.35727584066429,
0.));
#25062=CARTESIAN_POINT('Ctrl Pts',(-42.1428038039937,-2.31640554742808,
0.));
#25063=CARTESIAN_POINT('Ctrl Pts',(-42.2355611060784,-2.27498976664774,
0.));
#25064=CARTESIAN_POINT('Ctrl Pts',(-42.3282220118033,-2.23303287465499,
0.));
#25065=CARTESIAN_POINT('Ctrl Pts',(-42.4207850290047,-2.19053924976737,
0.));
#25066=CARTESIAN_POINT('Ctrl Pts',(-42.5132487024335,-2.14751319676745,
0.));
#25067=CARTESIAN_POINT('Ctrl Pts',(-42.6056116373456,-2.1039588640177,0.));
#25068=CARTESIAN_POINT('Ctrl Pts',(-42.6978725343209,-2.05988014924519,
0.));
#25069=CARTESIAN_POINT('Ctrl Pts',(-42.7900301875309,-2.01528067528089,
0.));
#25070=CARTESIAN_POINT('Ctrl Pts',(-42.8820834139973,-1.97016390194216,
0.));
#25071=CARTESIAN_POINT('Ctrl Pts',(-42.9740309956624,-1.92453321512435,
0.));
#25072=CARTESIAN_POINT('Ctrl Pts',(-43.065871623255,-1.87839202014609,0.));
#25073=CARTESIAN_POINT('Ctrl Pts',(-43.1576038253643,-1.83174385734711,
0.));
#25074=CARTESIAN_POINT('Ctrl Pts',(-43.2492259505872,-1.78459244842769,
0.));
#25075=CARTESIAN_POINT('Ctrl Pts',(-43.3407363140236,-1.73694151741123,
0.));
#25076=CARTESIAN_POINT('Ctrl Pts',(-43.4321333178711,-1.68879465270608,
0.));
#25077=CARTESIAN_POINT('Ctrl Pts',(-43.5234155788248,-1.64015515906648,
0.));
#25078=CARTESIAN_POINT('Ctrl Pts',(-43.6145820637333,-1.59102591108103,
0.));
#25079=CARTESIAN_POINT('Ctrl Pts',(-43.7238422193529,-1.53148589036096,
0.));
#25080=CARTESIAN_POINT('Ctrl Pts',(-43.8147465842503,-1.48126213998558,
0.));
#25081=CARTESIAN_POINT('Ctrl Pts',(-43.8873767449247,-1.44069595482723,
0.));
#25082=CARTESIAN_POINT('Ctrl Pts',(-43.9417969186811,-1.41005374202872,
0.));
#25083=CARTESIAN_POINT('Ctrl Pts',(-43.9780537249529,-1.38952890043916,
0.));
#25084=CARTESIAN_POINT('',(-43.9780537249529,-1.38952890043929,15.));
#25085=CARTESIAN_POINT('Ctrl Pts',(-43.9780537249529,-1.38952890043916,
15.));
#25086=CARTESIAN_POINT('Ctrl Pts',(-43.9599253218252,-1.39979132121931,
15.));
#25087=CARTESIAN_POINT('Ctrl Pts',(-43.9236568607623,-1.42026781296156,
15.));
#25088=CARTESIAN_POINT('Ctrl Pts',(-43.8692192047561,-1.45083750111682,
15.));
#25089=CARTESIAN_POINT('Ctrl Pts',(-43.7965657112708,-1.49130689006066,
15.));
#25090=CARTESIAN_POINT('Ctrl Pts',(-43.7056321934163,-1.54140922714764,
15.));
#25091=CARTESIAN_POINT('Ctrl Pts',(-43.6145820637333,-1.59102591108103,
15.));
#25092=CARTESIAN_POINT('Ctrl Pts',(-43.5234155788248,-1.64015515906648,
15.));
#25093=CARTESIAN_POINT('Ctrl Pts',(-43.4321333178711,-1.68879465270608,
15.));
#25094=CARTESIAN_POINT('Ctrl Pts',(-43.3407363140236,-1.73694151741123,
15.));
#25095=CARTESIAN_POINT('Ctrl Pts',(-43.2492259505872,-1.78459244842769,
15.));
#25096=CARTESIAN_POINT('Ctrl Pts',(-43.1576038253643,-1.83174385734711,
15.));
#25097=CARTESIAN_POINT('Ctrl Pts',(-43.065871623255,-1.87839202014609,15.));
#25098=CARTESIAN_POINT('Ctrl Pts',(-42.9740309956624,-1.92453321512435,
15.));
#25099=CARTESIAN_POINT('Ctrl Pts',(-42.8820834139973,-1.97016390194216,
15.));
#25100=CARTESIAN_POINT('Ctrl Pts',(-42.7900301875309,-2.01528067528089,
15.));
#25101=CARTESIAN_POINT('Ctrl Pts',(-42.6978725343209,-2.05988014924519,
15.));
#25102=CARTESIAN_POINT('Ctrl Pts',(-42.6056116373456,-2.1039588640177,15.));
#25103=CARTESIAN_POINT('Ctrl Pts',(-42.5132487024335,-2.14751319676745,
15.));
#25104=CARTESIAN_POINT('Ctrl Pts',(-42.4207850290047,-2.19053924976737,
15.));
#25105=CARTESIAN_POINT('Ctrl Pts',(-42.3282220118033,-2.23303287465499,
15.));
#25106=CARTESIAN_POINT('Ctrl Pts',(-42.2355611060784,-2.27498976664774,
15.));
#25107=CARTESIAN_POINT('Ctrl Pts',(-42.1428038039937,-2.31640554742808,
15.));
#25108=CARTESIAN_POINT('Ctrl Pts',(-42.0499516093661,-2.35727584066429,
15.));
#25109=CARTESIAN_POINT('Ctrl Pts',(-41.9570060084039,-2.39759639399648,
15.));
#25110=CARTESIAN_POINT('Ctrl Pts',(-41.8639684667923,-2.437363014342,15.));
#25111=CARTESIAN_POINT('Ctrl Pts',(-41.7708404467533,-2.47657137427693,
15.));
#25112=CARTESIAN_POINT('Ctrl Pts',(-41.6776234194583,-2.51521684674477,
15.));
#25113=CARTESIAN_POINT('Ctrl Pts',(-41.5843188786284,-2.55329436064184,
15.));
#25114=CARTESIAN_POINT('Ctrl Pts',(-41.4909283577703,-2.59079818040171,
15.));
#25115=CARTESIAN_POINT('Ctrl Pts',(-41.3974534325937,-2.62772200460656,
15.));
#25116=CARTESIAN_POINT('Ctrl Pts',(-41.3038957096306,-2.66405934050118,
15.));
#25117=CARTESIAN_POINT('Ctrl Pts',(-41.2102568187956,-2.69980383625015,
15.));
#25118=CARTESIAN_POINT('Ctrl Pts',(-41.1165384061145,-2.73494956725005,
15.));
#25119=CARTESIAN_POINT('Ctrl Pts',(-41.0227421242398,-2.76949151194863,
15.));
#25120=CARTESIAN_POINT('Ctrl Pts',(-40.9288696352159,-2.80342531768405,
15.));
#25121=CARTESIAN_POINT('Ctrl Pts',(-40.8349226258683,-2.83674635946679,
15.));
#25122=CARTESIAN_POINT('Ctrl Pts',(-40.7409028213129,-2.86944892209897,
15.));
#25123=CARTESIAN_POINT('Ctrl Pts',(-40.6468119976928,-2.90152548734342,
15.));
#25124=CARTESIAN_POINT('Ctrl Pts',(-40.5526520010651,-2.93296560822893,
15.));
#25125=CARTESIAN_POINT('Ctrl Pts',(-40.4584247445196,-2.96375636417322,
15.));
#25126=CARTESIAN_POINT('Ctrl Pts',(-40.3641321823444,-2.99388446458219,
15.));
#25127=CARTESIAN_POINT('Ctrl Pts',(-40.2697762886113,-3.02333808901595,
15.));
#25128=CARTESIAN_POINT('Ctrl Pts',(-40.1753590391515,-3.0521084742307,15.));
#25129=CARTESIAN_POINT('Ctrl Pts',(-40.0808823811787,-3.08019251155015,
15.));
#25130=CARTESIAN_POINT('Ctrl Pts',(-39.9863482523153,-3.10759149802907,
15.));
#25131=CARTESIAN_POINT('Ctrl Pts',(-39.8917586491576,-3.13430604330355,
15.));
#25132=CARTESIAN_POINT('Ctrl Pts',(-39.7971156880138,-3.16033160752803,
15.));
#25133=CARTESIAN_POINT('Ctrl Pts',(-39.7024216585552,-3.18565465503835,
15.));
#25134=CARTESIAN_POINT('Ctrl Pts',(-39.607679107639,-3.21024640045595,15.));
#25135=CARTESIAN_POINT('Ctrl Pts',(-39.5128908052622,-3.23406609691661,
15.));
#25136=CARTESIAN_POINT('Ctrl Pts',(-39.4180596080755,-3.25707264313388,
15.));
#25137=CARTESIAN_POINT('Ctrl Pts',(-39.3231883392913,-3.27923485388117,
15.));
#25138=CARTESIAN_POINT('Ctrl Pts',(-39.2282796893977,-3.30054018081687,
15.));
#25139=CARTESIAN_POINT('Ctrl Pts',(-39.1333360409949,-3.32100933979557,
15.));
#25140=CARTESIAN_POINT('Ctrl Pts',(-39.0383596151636,-3.34068601264472,
15.));
#25141=CARTESIAN_POINT('Ctrl Pts',(-38.9433528420174,-3.3596092279948,15.));
#25142=CARTESIAN_POINT('Ctrl Pts',(-38.8483186930884,-3.37778863054482,
15.));
#25143=CARTESIAN_POINT('Ctrl Pts',(-38.7532609709905,-3.39518333281818,
15.));
#25144=CARTESIAN_POINT('Ctrl Pts',(-38.6581847668347,-3.411667175119,15.));
#25145=CARTESIAN_POINT('Ctrl Pts',(-38.5630961226878,-3.42705871084996,
15.));
#25146=CARTESIAN_POINT('Ctrl Pts',(-38.4680013094732,-3.44118343200303,
15.));
#25147=CARTESIAN_POINT('Ctrl Pts',(-38.3729061502716,-3.45393053211022,
15.));
#25148=CARTESIAN_POINT('Ctrl Pts',(-38.2778154909527,-3.46530185256872,
15.));
#25149=CARTESIAN_POINT('Ctrl Pts',(-38.1827321816559,-3.47549027265411,
15.));
#25150=CARTESIAN_POINT('Ctrl Pts',(-38.0876589224537,-3.48478279878233,
15.));
#25151=CARTESIAN_POINT('Ctrl Pts',(-37.9926009950482,-3.49340804454645,
15.));
#25152=CARTESIAN_POINT('Ctrl Pts',(-37.8975688353863,-3.50139628556083,
15.));
#25153=CARTESIAN_POINT('Ctrl Pts',(-37.8025803811856,-3.50844720825128,
15.));
#25154=CARTESIAN_POINT('Ctrl Pts',(-37.7076643105286,-3.51375922979957,
15.));
#25155=CARTESIAN_POINT('Ctrl Pts',(-37.6128545966533,-3.51624243734645,
15.));
#25156=CARTESIAN_POINT('Ctrl Pts',(-37.5371179004295,-3.51508109065209,
15.));
#25157=CARTESIAN_POINT('Ctrl Pts',(-37.4803889700239,-3.51204731876361,
15.));
#25158=CARTESIAN_POINT('Ctrl Pts',(-37.4426037737699,-3.50901346997657,
15.));
#25159=CARTESIAN_POINT('Ctrl Pts',(-37.4237196983922,-3.50724370857673,
15.));
#25160=CARTESIAN_POINT('',(-43.9780537249529,-1.38952890043929,0.));
#25161=CARTESIAN_POINT('Origin',(-1.13331566353736E-11,5.04870979341448E-28,
0.));
#25162=CARTESIAN_POINT('',(-43.9780537249529,1.38952890043917,0.));
#25163=CARTESIAN_POINT('Origin',(-1.13331566353736E-11,5.04870979341448E-28,
0.));
#25164=CARTESIAN_POINT('',(-43.9780537249529,1.38952890043917,15.));
#25165=CARTESIAN_POINT('Origin',(-1.13331566353736E-11,5.04870979341448E-28,
15.));
#25166=CARTESIAN_POINT('',(-43.9780537249529,1.38952890043917,0.));
#25167=CARTESIAN_POINT('Ctrl Pts',(-37.4237196983923,3.50724370857673,0.));
#25168=CARTESIAN_POINT('Ctrl Pts',(-37.4237196983923,3.50724370857673,18.));
#25169=CARTESIAN_POINT('Ctrl Pts',(-37.4426037737699,3.50901346997657,0.));
#25170=CARTESIAN_POINT('Ctrl Pts',(-37.4426037737699,3.50901346997657,18.));
#25171=CARTESIAN_POINT('Ctrl Pts',(-37.4803889700239,3.51204731876362,0.));
#25172=CARTESIAN_POINT('Ctrl Pts',(-37.4803889700239,3.51204731876362,18.));
#25173=CARTESIAN_POINT('Ctrl Pts',(-37.5371179004295,3.5150810906521,0.));
#25174=CARTESIAN_POINT('Ctrl Pts',(-37.5371179004295,3.5150810906521,18.));
#25175=CARTESIAN_POINT('Ctrl Pts',(-37.6128545966533,3.51624243734645,0.));
#25176=CARTESIAN_POINT('Ctrl Pts',(-37.6128545966533,3.51624243734645,18.));
#25177=CARTESIAN_POINT('Ctrl Pts',(-37.7076643105286,3.51375922979958,0.));
#25178=CARTESIAN_POINT('Ctrl Pts',(-37.7076643105286,3.51375922979958,18.));
#25179=CARTESIAN_POINT('Ctrl Pts',(-37.8025803811856,3.50844720825129,0.));
#25180=CARTESIAN_POINT('Ctrl Pts',(-37.8025803811856,3.50844720825129,18.));
#25181=CARTESIAN_POINT('Ctrl Pts',(-37.8975688353863,3.50139628556084,0.));
#25182=CARTESIAN_POINT('Ctrl Pts',(-37.8975688353863,3.50139628556084,18.));
#25183=CARTESIAN_POINT('Ctrl Pts',(-37.9926009950482,3.49340804454646,0.));
#25184=CARTESIAN_POINT('Ctrl Pts',(-37.9926009950482,3.49340804454646,18.));
#25185=CARTESIAN_POINT('Ctrl Pts',(-38.0876589224537,3.48478279878234,0.));
#25186=CARTESIAN_POINT('Ctrl Pts',(-38.0876589224537,3.48478279878234,18.));
#25187=CARTESIAN_POINT('Ctrl Pts',(-38.1827321816559,3.47549027265412,0.));
#25188=CARTESIAN_POINT('Ctrl Pts',(-38.1827321816559,3.47549027265412,18.));
#25189=CARTESIAN_POINT('Ctrl Pts',(-38.2778154909527,3.46530185256873,0.));
#25190=CARTESIAN_POINT('Ctrl Pts',(-38.2778154909527,3.46530185256873,18.));
#25191=CARTESIAN_POINT('Ctrl Pts',(-38.3729061502716,3.45393053211023,0.));
#25192=CARTESIAN_POINT('Ctrl Pts',(-38.3729061502716,3.45393053211023,18.));
#25193=CARTESIAN_POINT('Ctrl Pts',(-38.4680013094732,3.44118343200304,0.));
#25194=CARTESIAN_POINT('Ctrl Pts',(-38.4680013094732,3.44118343200304,18.));
#25195=CARTESIAN_POINT('Ctrl Pts',(-38.5630961226878,3.42705871084997,0.));
#25196=CARTESIAN_POINT('Ctrl Pts',(-38.5630961226878,3.42705871084997,18.));
#25197=CARTESIAN_POINT('Ctrl Pts',(-38.6581847668347,3.41166717511901,0.));
#25198=CARTESIAN_POINT('Ctrl Pts',(-38.6581847668347,3.41166717511901,18.));
#25199=CARTESIAN_POINT('Ctrl Pts',(-38.7532609709905,3.39518333281819,0.));
#25200=CARTESIAN_POINT('Ctrl Pts',(-38.7532609709905,3.39518333281819,18.));
#25201=CARTESIAN_POINT('Ctrl Pts',(-38.8483186930884,3.37778863054482,0.));
#25202=CARTESIAN_POINT('Ctrl Pts',(-38.8483186930884,3.37778863054482,18.));
#25203=CARTESIAN_POINT('Ctrl Pts',(-38.9433528420174,3.35960922799481,0.));
#25204=CARTESIAN_POINT('Ctrl Pts',(-38.9433528420174,3.35960922799481,18.));
#25205=CARTESIAN_POINT('Ctrl Pts',(-39.0383596151636,3.34068601264473,0.));
#25206=CARTESIAN_POINT('Ctrl Pts',(-39.0383596151636,3.34068601264473,18.));
#25207=CARTESIAN_POINT('Ctrl Pts',(-39.1333360409949,3.32100933979558,0.));
#25208=CARTESIAN_POINT('Ctrl Pts',(-39.1333360409949,3.32100933979558,18.));
#25209=CARTESIAN_POINT('Ctrl Pts',(-39.2282796893977,3.30054018081688,0.));
#25210=CARTESIAN_POINT('Ctrl Pts',(-39.2282796893977,3.30054018081688,18.));
#25211=CARTESIAN_POINT('Ctrl Pts',(-39.3231883392913,3.27923485388118,0.));
#25212=CARTESIAN_POINT('Ctrl Pts',(-39.3231883392913,3.27923485388118,18.));
#25213=CARTESIAN_POINT('Ctrl Pts',(-39.4180596080755,3.25707264313388,0.));
#25214=CARTESIAN_POINT('Ctrl Pts',(-39.4180596080755,3.25707264313388,18.));
#25215=CARTESIAN_POINT('Ctrl Pts',(-39.5128908052622,3.23406609691661,0.));
#25216=CARTESIAN_POINT('Ctrl Pts',(-39.5128908052622,3.23406609691661,18.));
#25217=CARTESIAN_POINT('Ctrl Pts',(-39.607679107639,3.21024640045596,0.));
#25218=CARTESIAN_POINT('Ctrl Pts',(-39.607679107639,3.21024640045596,18.));
#25219=CARTESIAN_POINT('Ctrl Pts',(-39.7024216585552,3.18565465503836,0.));
#25220=CARTESIAN_POINT('Ctrl Pts',(-39.7024216585552,3.18565465503836,18.));
#25221=CARTESIAN_POINT('Ctrl Pts',(-39.7971156880138,3.16033160752804,0.));
#25222=CARTESIAN_POINT('Ctrl Pts',(-39.7971156880138,3.16033160752804,18.));
#25223=CARTESIAN_POINT('Ctrl Pts',(-39.8917586491576,3.13430604330356,0.));
#25224=CARTESIAN_POINT('Ctrl Pts',(-39.8917586491576,3.13430604330356,18.));
#25225=CARTESIAN_POINT('Ctrl Pts',(-39.9863482523153,3.10759149802908,0.));
#25226=CARTESIAN_POINT('Ctrl Pts',(-39.9863482523153,3.10759149802908,18.));
#25227=CARTESIAN_POINT('Ctrl Pts',(-40.0808823811787,3.08019251155016,0.));
#25228=CARTESIAN_POINT('Ctrl Pts',(-40.0808823811787,3.08019251155016,18.));
#25229=CARTESIAN_POINT('Ctrl Pts',(-40.1753590391515,3.05210847423071,0.));
#25230=CARTESIAN_POINT('Ctrl Pts',(-40.1753590391515,3.05210847423071,18.));
#25231=CARTESIAN_POINT('Ctrl Pts',(-40.2697762886113,3.02333808901596,0.));
#25232=CARTESIAN_POINT('Ctrl Pts',(-40.2697762886113,3.02333808901596,18.));
#25233=CARTESIAN_POINT('Ctrl Pts',(-40.3641321823444,2.9938844645822,0.));
#25234=CARTESIAN_POINT('Ctrl Pts',(-40.3641321823444,2.9938844645822,18.));
#25235=CARTESIAN_POINT('Ctrl Pts',(-40.4584247445196,2.96375636417323,0.));
#25236=CARTESIAN_POINT('Ctrl Pts',(-40.4584247445196,2.96375636417323,18.));
#25237=CARTESIAN_POINT('Ctrl Pts',(-40.5526520010651,2.93296560822894,0.));
#25238=CARTESIAN_POINT('Ctrl Pts',(-40.5526520010651,2.93296560822894,18.));
#25239=CARTESIAN_POINT('Ctrl Pts',(-40.6468119976928,2.90152548734343,0.));
#25240=CARTESIAN_POINT('Ctrl Pts',(-40.6468119976928,2.90152548734343,18.));
#25241=CARTESIAN_POINT('Ctrl Pts',(-40.7409028213129,2.86944892209898,0.));
#25242=CARTESIAN_POINT('Ctrl Pts',(-40.7409028213129,2.86944892209898,18.));
#25243=CARTESIAN_POINT('Ctrl Pts',(-40.8349226258683,2.8367463594668,0.));
#25244=CARTESIAN_POINT('Ctrl Pts',(-40.8349226258683,2.8367463594668,18.));
#25245=CARTESIAN_POINT('Ctrl Pts',(-40.9288696352159,2.80342531768405,0.));
#25246=CARTESIAN_POINT('Ctrl Pts',(-40.9288696352159,2.80342531768405,18.));
#25247=CARTESIAN_POINT('Ctrl Pts',(-41.0227421242398,2.76949151194864,0.));
#25248=CARTESIAN_POINT('Ctrl Pts',(-41.0227421242398,2.76949151194864,18.));
#25249=CARTESIAN_POINT('Ctrl Pts',(-41.1165384061145,2.73494956725006,0.));
#25250=CARTESIAN_POINT('Ctrl Pts',(-41.1165384061145,2.73494956725006,18.));
#25251=CARTESIAN_POINT('Ctrl Pts',(-41.2102568187956,2.69980383625016,0.));
#25252=CARTESIAN_POINT('Ctrl Pts',(-41.2102568187956,2.69980383625016,18.));
#25253=CARTESIAN_POINT('Ctrl Pts',(-41.3038957096306,2.66405934050119,0.));
#25254=CARTESIAN_POINT('Ctrl Pts',(-41.3038957096306,2.66405934050119,18.));
#25255=CARTESIAN_POINT('Ctrl Pts',(-41.3974534325937,2.62772200460657,0.));
#25256=CARTESIAN_POINT('Ctrl Pts',(-41.3974534325937,2.62772200460657,18.));
#25257=CARTESIAN_POINT('Ctrl Pts',(-41.4909283577703,2.59079818040173,0.));
#25258=CARTESIAN_POINT('Ctrl Pts',(-41.4909283577703,2.59079818040173,18.));
#25259=CARTESIAN_POINT('Ctrl Pts',(-41.5843188786284,2.55329436064184,0.));
#25260=CARTESIAN_POINT('Ctrl Pts',(-41.5843188786284,2.55329436064184,18.));
#25261=CARTESIAN_POINT('Ctrl Pts',(-41.6776234194583,2.51521684674477,0.));
#25262=CARTESIAN_POINT('Ctrl Pts',(-41.6776234194583,2.51521684674477,18.));
#25263=CARTESIAN_POINT('Ctrl Pts',(-41.7708404467533,2.47657137427693,0.));
#25264=CARTESIAN_POINT('Ctrl Pts',(-41.7708404467533,2.47657137427693,18.));
#25265=CARTESIAN_POINT('Ctrl Pts',(-41.8639684667923,2.43736301434201,0.));
#25266=CARTESIAN_POINT('Ctrl Pts',(-41.8639684667923,2.43736301434201,18.));
#25267=CARTESIAN_POINT('Ctrl Pts',(-41.9570060084039,2.39759639399648,0.));
#25268=CARTESIAN_POINT('Ctrl Pts',(-41.9570060084039,2.39759639399648,18.));
#25269=CARTESIAN_POINT('Ctrl Pts',(-42.0499516093661,2.3572758406643,0.));
#25270=CARTESIAN_POINT('Ctrl Pts',(-42.0499516093661,2.3572758406643,18.));
#25271=CARTESIAN_POINT('Ctrl Pts',(-42.1428038039937,2.3164055474281,0.));
#25272=CARTESIAN_POINT('Ctrl Pts',(-42.1428038039937,2.3164055474281,18.));
#25273=CARTESIAN_POINT('Ctrl Pts',(-42.2355611060784,2.27498976664775,0.));
#25274=CARTESIAN_POINT('Ctrl Pts',(-42.2355611060784,2.27498976664775,18.));
#25275=CARTESIAN_POINT('Ctrl Pts',(-42.3282220118033,2.233032874655,0.));
#25276=CARTESIAN_POINT('Ctrl Pts',(-42.3282220118033,2.233032874655,18.));
#25277=CARTESIAN_POINT('Ctrl Pts',(-42.4207850290047,2.19053924976738,0.));
#25278=CARTESIAN_POINT('Ctrl Pts',(-42.4207850290047,2.19053924976738,18.));
#25279=CARTESIAN_POINT('Ctrl Pts',(-42.5132487024335,2.14751319676746,0.));
#25280=CARTESIAN_POINT('Ctrl Pts',(-42.5132487024335,2.14751319676746,18.));
#25281=CARTESIAN_POINT('Ctrl Pts',(-42.6056116373456,2.10395886401771,0.));
#25282=CARTESIAN_POINT('Ctrl Pts',(-42.6056116373456,2.10395886401771,18.));
#25283=CARTESIAN_POINT('Ctrl Pts',(-42.6978725343209,2.0598801492452,0.));
#25284=CARTESIAN_POINT('Ctrl Pts',(-42.6978725343209,2.0598801492452,18.));
#25285=CARTESIAN_POINT('Ctrl Pts',(-42.7900301875309,2.0152806752809,0.));
#25286=CARTESIAN_POINT('Ctrl Pts',(-42.7900301875309,2.0152806752809,18.));
#25287=CARTESIAN_POINT('Ctrl Pts',(-42.8820834139973,1.97016390194217,0.));
#25288=CARTESIAN_POINT('Ctrl Pts',(-42.8820834139973,1.97016390194217,18.));
#25289=CARTESIAN_POINT('Ctrl Pts',(-42.9740309956624,1.92453321512436,0.));
#25290=CARTESIAN_POINT('Ctrl Pts',(-42.9740309956624,1.92453321512436,18.));
#25291=CARTESIAN_POINT('Ctrl Pts',(-43.065871623255,1.8783920201461,0.));
#25292=CARTESIAN_POINT('Ctrl Pts',(-43.065871623255,1.8783920201461,18.));
#25293=CARTESIAN_POINT('Ctrl Pts',(-43.1576038253643,1.83174385734712,0.));
#25294=CARTESIAN_POINT('Ctrl Pts',(-43.1576038253643,1.83174385734712,18.));
#25295=CARTESIAN_POINT('Ctrl Pts',(-43.2492259505872,1.7845924484277,0.));
#25296=CARTESIAN_POINT('Ctrl Pts',(-43.2492259505872,1.7845924484277,18.));
#25297=CARTESIAN_POINT('Ctrl Pts',(-43.3407363140236,1.73694151741124,0.));
#25298=CARTESIAN_POINT('Ctrl Pts',(-43.3407363140236,1.73694151741124,18.));
#25299=CARTESIAN_POINT('Ctrl Pts',(-43.4321333178711,1.68879465270609,0.));
#25300=CARTESIAN_POINT('Ctrl Pts',(-43.4321333178711,1.68879465270609,18.));
#25301=CARTESIAN_POINT('Ctrl Pts',(-43.5234155788248,1.64015515906649,0.));
#25302=CARTESIAN_POINT('Ctrl Pts',(-43.5234155788248,1.64015515906649,18.));
#25303=CARTESIAN_POINT('Ctrl Pts',(-43.6145820637333,1.59102591108104,0.));
#25304=CARTESIAN_POINT('Ctrl Pts',(-43.6145820637333,1.59102591108104,18.));
#25305=CARTESIAN_POINT('Ctrl Pts',(-43.7056321934163,1.54140922714765,0.));
#25306=CARTESIAN_POINT('Ctrl Pts',(-43.7056321934163,1.54140922714765,18.));
#25307=CARTESIAN_POINT('Ctrl Pts',(-43.7965657112708,1.49130689006067,0.));
#25308=CARTESIAN_POINT('Ctrl Pts',(-43.7965657112708,1.49130689006067,18.));
#25309=CARTESIAN_POINT('Ctrl Pts',(-43.8692192047561,1.45083750111683,0.));
#25310=CARTESIAN_POINT('Ctrl Pts',(-43.8692192047561,1.45083750111683,18.));
#25311=CARTESIAN_POINT('Ctrl Pts',(-43.9236568607623,1.42026781296157,0.));
#25312=CARTESIAN_POINT('Ctrl Pts',(-43.9236568607623,1.42026781296157,18.));
#25313=CARTESIAN_POINT('Ctrl Pts',(-43.9599253218252,1.39979132121932,0.));
#25314=CARTESIAN_POINT('Ctrl Pts',(-43.9599253218252,1.39979132121932,18.));
#25315=CARTESIAN_POINT('Ctrl Pts',(-43.9780537249529,1.38952890043917,0.));
#25316=CARTESIAN_POINT('Ctrl Pts',(-43.9780537249529,1.38952890043917,18.));
#25317=CARTESIAN_POINT('Ctrl Pts',(-37.4237196983923,3.50724370857673,0.));
#25318=CARTESIAN_POINT('Ctrl Pts',(-37.4426037737699,3.50901346997657,0.));
#25319=CARTESIAN_POINT('Ctrl Pts',(-37.4803889700239,3.51204731876362,0.));
#25320=CARTESIAN_POINT('Ctrl Pts',(-37.5371179004295,3.5150810906521,0.));
#25321=CARTESIAN_POINT('Ctrl Pts',(-37.6128545966533,3.51624243734645,0.));
#25322=CARTESIAN_POINT('Ctrl Pts',(-37.7076643105286,3.51375922979958,0.));
#25323=CARTESIAN_POINT('Ctrl Pts',(-37.8025803811856,3.50844720825129,0.));
#25324=CARTESIAN_POINT('Ctrl Pts',(-37.8975688353863,3.50139628556084,0.));
#25325=CARTESIAN_POINT('Ctrl Pts',(-37.9926009950482,3.49340804454646,0.));
#25326=CARTESIAN_POINT('Ctrl Pts',(-38.0876589224537,3.48478279878234,0.));
#25327=CARTESIAN_POINT('Ctrl Pts',(-38.1827321816559,3.47549027265412,0.));
#25328=CARTESIAN_POINT('Ctrl Pts',(-38.2778154909527,3.46530185256873,0.));
#25329=CARTESIAN_POINT('Ctrl Pts',(-38.3729061502716,3.45393053211023,0.));
#25330=CARTESIAN_POINT('Ctrl Pts',(-38.4680013094732,3.44118343200304,0.));
#25331=CARTESIAN_POINT('Ctrl Pts',(-38.5630961226878,3.42705871084997,0.));
#25332=CARTESIAN_POINT('Ctrl Pts',(-38.6581847668347,3.41166717511901,0.));
#25333=CARTESIAN_POINT('Ctrl Pts',(-38.7532609709905,3.39518333281819,0.));
#25334=CARTESIAN_POINT('Ctrl Pts',(-38.8483186930884,3.37778863054482,0.));
#25335=CARTESIAN_POINT('Ctrl Pts',(-38.9433528420174,3.35960922799481,0.));
#25336=CARTESIAN_POINT('Ctrl Pts',(-39.0383596151636,3.34068601264473,0.));
#25337=CARTESIAN_POINT('Ctrl Pts',(-39.1333360409949,3.32100933979558,0.));
#25338=CARTESIAN_POINT('Ctrl Pts',(-39.2282796893977,3.30054018081688,0.));
#25339=CARTESIAN_POINT('Ctrl Pts',(-39.3231883392913,3.27923485388118,0.));
#25340=CARTESIAN_POINT('Ctrl Pts',(-39.4180596080755,3.25707264313388,0.));
#25341=CARTESIAN_POINT('Ctrl Pts',(-39.5128908052622,3.23406609691661,0.));
#25342=CARTESIAN_POINT('Ctrl Pts',(-39.607679107639,3.21024640045596,0.));
#25343=CARTESIAN_POINT('Ctrl Pts',(-39.7024216585552,3.18565465503836,0.));
#25344=CARTESIAN_POINT('Ctrl Pts',(-39.7971156880138,3.16033160752804,0.));
#25345=CARTESIAN_POINT('Ctrl Pts',(-39.8917586491576,3.13430604330356,0.));
#25346=CARTESIAN_POINT('Ctrl Pts',(-39.9863482523153,3.10759149802908,0.));
#25347=CARTESIAN_POINT('Ctrl Pts',(-40.0808823811787,3.08019251155016,0.));
#25348=CARTESIAN_POINT('Ctrl Pts',(-40.1753590391515,3.05210847423071,0.));
#25349=CARTESIAN_POINT('Ctrl Pts',(-40.2697762886113,3.02333808901596,0.));
#25350=CARTESIAN_POINT('Ctrl Pts',(-40.3641321823444,2.9938844645822,0.));
#25351=CARTESIAN_POINT('Ctrl Pts',(-40.4584247445196,2.96375636417323,0.));
#25352=CARTESIAN_POINT('Ctrl Pts',(-40.5526520010651,2.93296560822894,0.));
#25353=CARTESIAN_POINT('Ctrl Pts',(-40.6468119976928,2.90152548734343,0.));
#25354=CARTESIAN_POINT('Ctrl Pts',(-40.7409028213129,2.86944892209898,0.));
#25355=CARTESIAN_POINT('Ctrl Pts',(-40.8349226258683,2.8367463594668,0.));
#25356=CARTESIAN_POINT('Ctrl Pts',(-40.9288696352159,2.80342531768405,0.));
#25357=CARTESIAN_POINT('Ctrl Pts',(-41.0227421242398,2.76949151194864,0.));
#25358=CARTESIAN_POINT('Ctrl Pts',(-41.1165384061145,2.73494956725006,0.));
#25359=CARTESIAN_POINT('Ctrl Pts',(-41.2102568187956,2.69980383625016,0.));
#25360=CARTESIAN_POINT('Ctrl Pts',(-41.3038957096306,2.66405934050119,0.));
#25361=CARTESIAN_POINT('Ctrl Pts',(-41.3974534325937,2.62772200460657,0.));
#25362=CARTESIAN_POINT('Ctrl Pts',(-41.4909283577703,2.59079818040173,0.));
#25363=CARTESIAN_POINT('Ctrl Pts',(-41.5843188786284,2.55329436064184,0.));
#25364=CARTESIAN_POINT('Ctrl Pts',(-41.6776234194583,2.51521684674477,0.));
#25365=CARTESIAN_POINT('Ctrl Pts',(-41.7708404467533,2.47657137427693,0.));
#25366=CARTESIAN_POINT('Ctrl Pts',(-41.8639684667923,2.43736301434201,0.));
#25367=CARTESIAN_POINT('Ctrl Pts',(-41.9570060084039,2.39759639399648,0.));
#25368=CARTESIAN_POINT('Ctrl Pts',(-42.0499516093661,2.3572758406643,0.));
#25369=CARTESIAN_POINT('Ctrl Pts',(-42.1428038039937,2.3164055474281,0.));
#25370=CARTESIAN_POINT('Ctrl Pts',(-42.2355611060784,2.27498976664775,0.));
#25371=CARTESIAN_POINT('Ctrl Pts',(-42.3282220118033,2.233032874655,0.));
#25372=CARTESIAN_POINT('Ctrl Pts',(-42.4207850290047,2.19053924976738,0.));
#25373=CARTESIAN_POINT('Ctrl Pts',(-42.5132487024335,2.14751319676746,0.));
#25374=CARTESIAN_POINT('Ctrl Pts',(-42.6056116373456,2.10395886401771,0.));
#25375=CARTESIAN_POINT('Ctrl Pts',(-42.6978725343209,2.0598801492452,0.));
#25376=CARTESIAN_POINT('Ctrl Pts',(-42.7900301875309,2.0152806752809,0.));
#25377=CARTESIAN_POINT('Ctrl Pts',(-42.8820834139973,1.97016390194217,0.));
#25378=CARTESIAN_POINT('Ctrl Pts',(-42.9740309956624,1.92453321512436,0.));
#25379=CARTESIAN_POINT('Ctrl Pts',(-43.065871623255,1.8783920201461,0.));
#25380=CARTESIAN_POINT('Ctrl Pts',(-43.1576038253643,1.83174385734712,0.));
#25381=CARTESIAN_POINT('Ctrl Pts',(-43.2492259505872,1.7845924484277,0.));
#25382=CARTESIAN_POINT('Ctrl Pts',(-43.3407363140236,1.73694151741124,0.));
#25383=CARTESIAN_POINT('Ctrl Pts',(-43.4321333178711,1.68879465270609,0.));
#25384=CARTESIAN_POINT('Ctrl Pts',(-43.5234155788248,1.64015515906649,0.));
#25385=CARTESIAN_POINT('Ctrl Pts',(-43.6145820637333,1.59102591108104,0.));
#25386=CARTESIAN_POINT('Ctrl Pts',(-43.7238422193529,1.53148589036097,0.));
#25387=CARTESIAN_POINT('Ctrl Pts',(-43.8147465842503,1.48126213998559,0.));
#25388=CARTESIAN_POINT('Ctrl Pts',(-43.8873767449247,1.44069595482724,0.));
#25389=CARTESIAN_POINT('Ctrl Pts',(-43.9417969186811,1.41005374202873,0.));
#25390=CARTESIAN_POINT('Ctrl Pts',(-43.9780537249529,1.38952890043917,0.));
#25391=CARTESIAN_POINT('Ctrl Pts',(-37.4237196983923,3.50724370857673,15.));
#25392=CARTESIAN_POINT('Ctrl Pts',(-37.4426037737699,3.50901346997657,15.));
#25393=CARTESIAN_POINT('Ctrl Pts',(-37.4803889700239,3.51204731876362,15.));
#25394=CARTESIAN_POINT('Ctrl Pts',(-37.5371179004295,3.5150810906521,15.));
#25395=CARTESIAN_POINT('Ctrl Pts',(-37.6128545966533,3.51624243734645,15.));
#25396=CARTESIAN_POINT('Ctrl Pts',(-37.7076643105286,3.51375922979958,15.));
#25397=CARTESIAN_POINT('Ctrl Pts',(-37.8025803811856,3.50844720825129,15.));
#25398=CARTESIAN_POINT('Ctrl Pts',(-37.8975688353863,3.50139628556084,15.));
#25399=CARTESIAN_POINT('Ctrl Pts',(-37.9926009950482,3.49340804454646,15.));
#25400=CARTESIAN_POINT('Ctrl Pts',(-38.0876589224537,3.48478279878234,15.));
#25401=CARTESIAN_POINT('Ctrl Pts',(-38.1827321816559,3.47549027265412,15.));
#25402=CARTESIAN_POINT('Ctrl Pts',(-38.2778154909527,3.46530185256873,15.));
#25403=CARTESIAN_POINT('Ctrl Pts',(-38.3729061502716,3.45393053211023,15.));
#25404=CARTESIAN_POINT('Ctrl Pts',(-38.4680013094732,3.44118343200304,15.));
#25405=CARTESIAN_POINT('Ctrl Pts',(-38.5630961226878,3.42705871084997,15.));
#25406=CARTESIAN_POINT('Ctrl Pts',(-38.6581847668347,3.41166717511901,15.));
#25407=CARTESIAN_POINT('Ctrl Pts',(-38.7532609709905,3.39518333281819,15.));
#25408=CARTESIAN_POINT('Ctrl Pts',(-38.8483186930884,3.37778863054482,15.));
#25409=CARTESIAN_POINT('Ctrl Pts',(-38.9433528420174,3.35960922799481,15.));
#25410=CARTESIAN_POINT('Ctrl Pts',(-39.0383596151636,3.34068601264473,15.));
#25411=CARTESIAN_POINT('Ctrl Pts',(-39.1333360409949,3.32100933979558,15.));
#25412=CARTESIAN_POINT('Ctrl Pts',(-39.2282796893977,3.30054018081688,15.));
#25413=CARTESIAN_POINT('Ctrl Pts',(-39.3231883392913,3.27923485388118,15.));
#25414=CARTESIAN_POINT('Ctrl Pts',(-39.4180596080755,3.25707264313388,15.));
#25415=CARTESIAN_POINT('Ctrl Pts',(-39.5128908052622,3.23406609691661,15.));
#25416=CARTESIAN_POINT('Ctrl Pts',(-39.607679107639,3.21024640045596,15.));
#25417=CARTESIAN_POINT('Ctrl Pts',(-39.7024216585552,3.18565465503836,15.));
#25418=CARTESIAN_POINT('Ctrl Pts',(-39.7971156880138,3.16033160752804,15.));
#25419=CARTESIAN_POINT('Ctrl Pts',(-39.8917586491576,3.13430604330356,15.));
#25420=CARTESIAN_POINT('Ctrl Pts',(-39.9863482523153,3.10759149802908,15.));
#25421=CARTESIAN_POINT('Ctrl Pts',(-40.0808823811787,3.08019251155016,15.));
#25422=CARTESIAN_POINT('Ctrl Pts',(-40.1753590391515,3.05210847423071,15.));
#25423=CARTESIAN_POINT('Ctrl Pts',(-40.2697762886113,3.02333808901596,15.));
#25424=CARTESIAN_POINT('Ctrl Pts',(-40.3641321823444,2.9938844645822,15.));
#25425=CARTESIAN_POINT('Ctrl Pts',(-40.4584247445196,2.96375636417323,15.));
#25426=CARTESIAN_POINT('Ctrl Pts',(-40.5526520010651,2.93296560822894,15.));
#25427=CARTESIAN_POINT('Ctrl Pts',(-40.6468119976928,2.90152548734343,15.));
#25428=CARTESIAN_POINT('Ctrl Pts',(-40.7409028213129,2.86944892209898,15.));
#25429=CARTESIAN_POINT('Ctrl Pts',(-40.8349226258683,2.8367463594668,15.));
#25430=CARTESIAN_POINT('Ctrl Pts',(-40.9288696352159,2.80342531768405,15.));
#25431=CARTESIAN_POINT('Ctrl Pts',(-41.0227421242398,2.76949151194864,15.));
#25432=CARTESIAN_POINT('Ctrl Pts',(-41.1165384061145,2.73494956725006,15.));
#25433=CARTESIAN_POINT('Ctrl Pts',(-41.2102568187956,2.69980383625016,15.));
#25434=CARTESIAN_POINT('Ctrl Pts',(-41.3038957096306,2.66405934050119,15.));
#25435=CARTESIAN_POINT('Ctrl Pts',(-41.3974534325937,2.62772200460657,15.));
#25436=CARTESIAN_POINT('Ctrl Pts',(-41.4909283577703,2.59079818040173,15.));
#25437=CARTESIAN_POINT('Ctrl Pts',(-41.5843188786284,2.55329436064184,15.));
#25438=CARTESIAN_POINT('Ctrl Pts',(-41.6776234194583,2.51521684674477,15.));
#25439=CARTESIAN_POINT('Ctrl Pts',(-41.7708404467533,2.47657137427693,15.));
#25440=CARTESIAN_POINT('Ctrl Pts',(-41.8639684667923,2.43736301434201,15.));
#25441=CARTESIAN_POINT('Ctrl Pts',(-41.9570060084039,2.39759639399648,15.));
#25442=CARTESIAN_POINT('Ctrl Pts',(-42.0499516093661,2.3572758406643,15.));
#25443=CARTESIAN_POINT('Ctrl Pts',(-42.1428038039937,2.3164055474281,15.));
#25444=CARTESIAN_POINT('Ctrl Pts',(-42.2355611060784,2.27498976664775,15.));
#25445=CARTESIAN_POINT('Ctrl Pts',(-42.3282220118033,2.233032874655,15.));
#25446=CARTESIAN_POINT('Ctrl Pts',(-42.4207850290047,2.19053924976738,15.));
#25447=CARTESIAN_POINT('Ctrl Pts',(-42.5132487024335,2.14751319676746,15.));
#25448=CARTESIAN_POINT('Ctrl Pts',(-42.6056116373456,2.10395886401771,15.));
#25449=CARTESIAN_POINT('Ctrl Pts',(-42.6978725343209,2.0598801492452,15.));
#25450=CARTESIAN_POINT('Ctrl Pts',(-42.7900301875309,2.0152806752809,15.));
#25451=CARTESIAN_POINT('Ctrl Pts',(-42.8820834139973,1.97016390194217,15.));
#25452=CARTESIAN_POINT('Ctrl Pts',(-42.9740309956624,1.92453321512436,15.));
#25453=CARTESIAN_POINT('Ctrl Pts',(-43.065871623255,1.8783920201461,15.));
#25454=CARTESIAN_POINT('Ctrl Pts',(-43.1576038253643,1.83174385734712,15.));
#25455=CARTESIAN_POINT('Ctrl Pts',(-43.2492259505872,1.7845924484277,15.));
#25456=CARTESIAN_POINT('Ctrl Pts',(-43.3407363140236,1.73694151741124,15.));
#25457=CARTESIAN_POINT('Ctrl Pts',(-43.4321333178711,1.68879465270609,15.));
#25458=CARTESIAN_POINT('Ctrl Pts',(-43.5234155788248,1.64015515906649,15.));
#25459=CARTESIAN_POINT('Ctrl Pts',(-43.6145820637333,1.59102591108104,15.));
#25460=CARTESIAN_POINT('Ctrl Pts',(-43.7238422193529,1.53148589036097,15.));
#25461=CARTESIAN_POINT('Ctrl Pts',(-43.8147465842503,1.48126213998559,15.));
#25462=CARTESIAN_POINT('Ctrl Pts',(-43.8873767449247,1.44069595482724,15.));
#25463=CARTESIAN_POINT('Ctrl Pts',(-43.9417969186811,1.41005374202873,15.));
#25464=CARTESIAN_POINT('Ctrl Pts',(-43.9780537249529,1.38952890043917,15.));
#25465=CARTESIAN_POINT('Ctrl Pts',(-42.2550026135057,12.2684454652018,0.));
#25466=CARTESIAN_POINT('Ctrl Pts',(-42.2550026135057,12.2684454652018,18.));
#25467=CARTESIAN_POINT('Ctrl Pts',(-42.2409327400055,12.2530833383985,0.));
#25468=CARTESIAN_POINT('Ctrl Pts',(-42.2409327400055,12.2530833383985,18.));
#25469=CARTESIAN_POINT('Ctrl Pts',(-42.2127669677092,12.222401466668,0.));
#25470=CARTESIAN_POINT('Ctrl Pts',(-42.2127669677092,12.222401466668,18.));
#25471=CARTESIAN_POINT('Ctrl Pts',(-42.1704402333854,12.1765058047069,0.));
#25472=CARTESIAN_POINT('Ctrl Pts',(-42.1704402333854,12.1765058047069,18.));
#25473=CARTESIAN_POINT('Ctrl Pts',(-42.1138483839101,12.1155659644537,0.));
#25474=CARTESIAN_POINT('Ctrl Pts',(-42.1138483839101,12.1155659644537,18.));
#25475=CARTESIAN_POINT('Ctrl Pts',(-42.0428479428228,12.0398158079102,0.));
#25476=CARTESIAN_POINT('Ctrl Pts',(-42.0428479428228,12.0398158079102,18.));
#25477=CARTESIAN_POINT('Ctrl Pts',(-41.9715865222182,11.9644914999263,0.));
#25478=CARTESIAN_POINT('Ctrl Pts',(-41.9715865222182,11.9644914999263,18.));
#25479=CARTESIAN_POINT('Ctrl Pts',(-41.9000638152266,11.8895948153349,0.));
#25480=CARTESIAN_POINT('Ctrl Pts',(-41.9000638152266,11.8895948153349,18.));
#25481=CARTESIAN_POINT('Ctrl Pts',(-41.8282796562569,11.81512813804,0.));
#25482=CARTESIAN_POINT('Ctrl Pts',(-41.8282796562569,11.81512813804,18.));
#25483=CARTESIAN_POINT('Ctrl Pts',(-41.7562341395977,11.7410945211992,0.));
#25484=CARTESIAN_POINT('Ctrl Pts',(-41.7562341395977,11.7410945211992,18.));
#25485=CARTESIAN_POINT('Ctrl Pts',(-41.6839275596248,11.6674975352852,0.));
#25486=CARTESIAN_POINT('Ctrl Pts',(-41.6839275596248,11.6674975352852,18.));
#25487=CARTESIAN_POINT('Ctrl Pts',(-41.6113603270596,11.5943410868252,0.));
#25488=CARTESIAN_POINT('Ctrl Pts',(-41.6113603270596,11.5943410868252,18.));
#25489=CARTESIAN_POINT('Ctrl Pts',(-41.5385328935506,11.5216292382388,0.));
#25490=CARTESIAN_POINT('Ctrl Pts',(-41.5385328935506,11.5216292382388,18.));
#25491=CARTESIAN_POINT('Ctrl Pts',(-41.4654456796071,11.4493660393849,0.));
#25492=CARTESIAN_POINT('Ctrl Pts',(-41.4654456796071,11.4493660393849,18.));
#25493=CARTESIAN_POINT('Ctrl Pts',(-41.3920989905986,11.3775553120176,0.));
#25494=CARTESIAN_POINT('Ctrl Pts',(-41.3920989905986,11.3775553120176,18.));
#25495=CARTESIAN_POINT('Ctrl Pts',(-41.3184930194148,11.3062006993745,0.));
#25496=CARTESIAN_POINT('Ctrl Pts',(-41.3184930194148,11.3062006993745,18.));
#25497=CARTESIAN_POINT('Ctrl Pts',(-41.2446278781981,11.2353057980338,0.));
#25498=CARTESIAN_POINT('Ctrl Pts',(-41.2446278781981,11.2353057980338,18.));
#25499=CARTESIAN_POINT('Ctrl Pts',(-41.1705036228854,11.1648742640378,0.));
#25500=CARTESIAN_POINT('Ctrl Pts',(-41.1705036228854,11.1648742640378,18.));
#25501=CARTESIAN_POINT('Ctrl Pts',(-41.0961202807715,11.0949099155251,0.));
#25502=CARTESIAN_POINT('Ctrl Pts',(-41.0961202807715,11.0949099155251,18.));
#25503=CARTESIAN_POINT('Ctrl Pts',(-41.0214778832142,11.0254168609972,0.));
#25504=CARTESIAN_POINT('Ctrl Pts',(-41.0214778832142,11.0254168609972,18.));
#25505=CARTESIAN_POINT('Ctrl Pts',(-40.9465764747798,10.956399476781,0.));
#25506=CARTESIAN_POINT('Ctrl Pts',(-40.9465764747798,10.956399476781,18.));
#25507=CARTESIAN_POINT('Ctrl Pts',(-40.8714161092412,10.8878623066646,0.));
#25508=CARTESIAN_POINT('Ctrl Pts',(-40.8714161092412,10.8878623066646,18.));
#25509=CARTESIAN_POINT('Ctrl Pts',(-40.7959968527561,10.8198099757795,0.));
#25510=CARTESIAN_POINT('Ctrl Pts',(-40.7959968527561,10.8198099757795,18.));
#25511=CARTESIAN_POINT('Ctrl Pts',(-40.7203187831783,10.7522471109694,0.));
#25512=CARTESIAN_POINT('Ctrl Pts',(-40.7203187831783,10.7522471109694,18.));
#25513=CARTESIAN_POINT('Ctrl Pts',(-40.6443819999244,10.6851782157325,0.));
#25514=CARTESIAN_POINT('Ctrl Pts',(-40.6443819999244,10.6851782157325,18.));
#25515=CARTESIAN_POINT('Ctrl Pts',(-40.5681866012103,10.618607730849,0.));
#25516=CARTESIAN_POINT('Ctrl Pts',(-40.5681866012103,10.618607730849,18.));
#25517=CARTESIAN_POINT('Ctrl Pts',(-40.4917326404439,10.5525402237951,0.));
#25518=CARTESIAN_POINT('Ctrl Pts',(-40.4917326404439,10.5525402237951,18.));
#25519=CARTESIAN_POINT('Ctrl Pts',(-40.4150200869536,10.48698054978,0.));
#25520=CARTESIAN_POINT('Ctrl Pts',(-40.4150200869536,10.48698054978,18.));
#25521=CARTESIAN_POINT('Ctrl Pts',(-40.3380487942952,10.4219339932951,0.));
#25522=CARTESIAN_POINT('Ctrl Pts',(-40.3380487942952,10.4219339932951,18.));
#25523=CARTESIAN_POINT('Ctrl Pts',(-40.2608184485326,10.3574064830678,0.));
#25524=CARTESIAN_POINT('Ctrl Pts',(-40.2608184485326,10.3574064830678,18.));
#25525=CARTESIAN_POINT('Ctrl Pts',(-40.1833286010098,10.2934044990237,0.));
#25526=CARTESIAN_POINT('Ctrl Pts',(-40.1833286010098,10.2934044990237,18.));
#25527=CARTESIAN_POINT('Ctrl Pts',(-40.1055787732578,10.2299347125857,0.));
#25528=CARTESIAN_POINT('Ctrl Pts',(-40.1055787732578,10.2299347125857,18.));
#25529=CARTESIAN_POINT('Ctrl Pts',(-40.0275685525923,10.1670036683795,0.));
#25530=CARTESIAN_POINT('Ctrl Pts',(-40.0275685525923,10.1670036683795,18.));
#25531=CARTESIAN_POINT('Ctrl Pts',(-39.9492976736738,10.1046175096878,0.));
#25532=CARTESIAN_POINT('Ctrl Pts',(-39.9492976736738,10.1046175096878,18.));
#25533=CARTESIAN_POINT('Ctrl Pts',(-39.8707661565233,10.0427815229883,0.));
#25534=CARTESIAN_POINT('Ctrl Pts',(-39.8707661565233,10.0427815229883,18.));
#25535=CARTESIAN_POINT('Ctrl Pts',(-39.7919742367922,9.98150036150823,0.));
#25536=CARTESIAN_POINT('Ctrl Pts',(-39.7919742367922,9.98150036150823,18.));
#25537=CARTESIAN_POINT('Ctrl Pts',(-39.712922089547,9.92077894513192,0.));
#25538=CARTESIAN_POINT('Ctrl Pts',(-39.712922089547,9.92077894513192,18.));
#25539=CARTESIAN_POINT('Ctrl Pts',(-39.6336095893767,9.8606232424256,0.));
#25540=CARTESIAN_POINT('Ctrl Pts',(-39.6336095893767,9.8606232424256,18.));
#25541=CARTESIAN_POINT('Ctrl Pts',(-39.5540361022309,9.80104095251614,0.));
#25542=CARTESIAN_POINT('Ctrl Pts',(-39.5540361022309,9.80104095251614,18.));
#25543=CARTESIAN_POINT('Ctrl Pts',(-39.4742001555227,9.74204258152664,0.));
#25544=CARTESIAN_POINT('Ctrl Pts',(-39.4742001555227,9.74204258152664,18.));
#25545=CARTESIAN_POINT('Ctrl Pts',(-39.3940995760289,9.68364100883827,0.));
#25546=CARTESIAN_POINT('Ctrl Pts',(-39.3940995760289,9.68364100883827,18.));
#25547=CARTESIAN_POINT('Ctrl Pts',(-39.3137321153686,9.62584947846543,0.));
#25548=CARTESIAN_POINT('Ctrl Pts',(-39.3137321153686,9.62584947846543,18.));
#25549=CARTESIAN_POINT('Ctrl Pts',(-39.2330959982788,9.56867984233623,0.));
#25550=CARTESIAN_POINT('Ctrl Pts',(-39.2330959982788,9.56867984233623,18.));
#25551=CARTESIAN_POINT('Ctrl Pts',(-39.1521903958955,9.51214104535621,0.));
#25552=CARTESIAN_POINT('Ctrl Pts',(-39.1521903958955,9.51214104535621,18.));
#25553=CARTESIAN_POINT('Ctrl Pts',(-39.071016199495,9.45623664577432,0.));
#25554=CARTESIAN_POINT('Ctrl Pts',(-39.071016199495,9.45623664577432,18.));
#25555=CARTESIAN_POINT('Ctrl Pts',(-38.9895756526779,9.40096600877644,0.));
#25556=CARTESIAN_POINT('Ctrl Pts',(-38.9895756526779,9.40096600877644,18.));
#25557=CARTESIAN_POINT('Ctrl Pts',(-38.9078708427078,9.34632917154637,0.));
#25558=CARTESIAN_POINT('Ctrl Pts',(-38.9078708427078,9.34632917154637,18.));
#25559=CARTESIAN_POINT('Ctrl Pts',(-38.8259023794241,9.29233110570903,0.));
#25560=CARTESIAN_POINT('Ctrl Pts',(-38.8259023794241,9.29233110570903,18.));
#25561=CARTESIAN_POINT('Ctrl Pts',(-38.7436682576832,9.23898539199332,0.));
#25562=CARTESIAN_POINT('Ctrl Pts',(-38.7436682576832,9.23898539199332,18.));
#25563=CARTESIAN_POINT('Ctrl Pts',(-38.6611620045193,9.1863201939433,0.));
#25564=CARTESIAN_POINT('Ctrl Pts',(-38.6611620045193,9.1863201939433,18.));
#25565=CARTESIAN_POINT('Ctrl Pts',(-38.5783736628826,9.13437512010586,0.));
#25566=CARTESIAN_POINT('Ctrl Pts',(-38.5783736628826,9.13437512010586,18.));
#25567=CARTESIAN_POINT('Ctrl Pts',(-38.4952932486131,9.08319014288086,0.));
#25568=CARTESIAN_POINT('Ctrl Pts',(-38.4952932486131,9.08319014288086,18.));
#25569=CARTESIAN_POINT('Ctrl Pts',(-38.4119138099805,9.03279579360191,0.));
#25570=CARTESIAN_POINT('Ctrl Pts',(-38.4119138099805,9.03279579360191,18.));
#25571=CARTESIAN_POINT('Ctrl Pts',(-38.3282340281403,8.9832048378576,0.));
#25572=CARTESIAN_POINT('Ctrl Pts',(-38.3282340281403,8.9832048378576,18.));
#25573=CARTESIAN_POINT('Ctrl Pts',(-38.2442625706309,8.93439830996339,0.));
#25574=CARTESIAN_POINT('Ctrl Pts',(-38.2442625706309,8.93439830996339,18.));
#25575=CARTESIAN_POINT('Ctrl Pts',(-38.1600150482528,8.88633535238434,0.));
#25576=CARTESIAN_POINT('Ctrl Pts',(-38.1600150482528,8.88633535238434,18.));
#25577=CARTESIAN_POINT('Ctrl Pts',(-38.0755058326913,8.83897959763349,0.));
#25578=CARTESIAN_POINT('Ctrl Pts',(-38.0755058326913,8.83897959763349,18.));
#25579=CARTESIAN_POINT('Ctrl Pts',(-37.9907407304174,8.79232279131092,0.));
#25580=CARTESIAN_POINT('Ctrl Pts',(-37.9907407304174,8.79232279131092,18.));
#25581=CARTESIAN_POINT('Ctrl Pts',(-37.9057107230066,8.74640499479002,0.));
#25582=CARTESIAN_POINT('Ctrl Pts',(-37.9057107230066,8.74640499479002,18.));
#25583=CARTESIAN_POINT('Ctrl Pts',(-37.8203816669031,8.70134776631143,0.));
#25584=CARTESIAN_POINT('Ctrl Pts',(-37.8203816669031,8.70134776631143,18.));
#25585=CARTESIAN_POINT('Ctrl Pts',(-37.7347032383719,8.65732553894525,0.));
#25586=CARTESIAN_POINT('Ctrl Pts',(-37.7347032383719,8.65732553894525,18.));
#25587=CARTESIAN_POINT('Ctrl Pts',(-37.6486274754754,8.61450621749155,0.));
#25588=CARTESIAN_POINT('Ctrl Pts',(-37.6486274754754,8.61450621749155,18.));
#25589=CARTESIAN_POINT('Ctrl Pts',(-37.5621256752108,8.57299698459466,0.));
#25590=CARTESIAN_POINT('Ctrl Pts',(-37.5621256752108,8.57299698459466,18.));
#25591=CARTESIAN_POINT('Ctrl Pts',(-37.4752030152968,8.53279758643785,0.));
#25592=CARTESIAN_POINT('Ctrl Pts',(-37.4752030152968,8.53279758643785,18.));
#25593=CARTESIAN_POINT('Ctrl Pts',(-37.3879218093514,8.49372546467076,0.));
#25594=CARTESIAN_POINT('Ctrl Pts',(-37.3879218093514,8.49372546467076,18.));
#25595=CARTESIAN_POINT('Ctrl Pts',(-37.3003733151561,8.4555084943396,0.));
#25596=CARTESIAN_POINT('Ctrl Pts',(-37.3003733151561,8.4555084943396,18.));
#25597=CARTESIAN_POINT('Ctrl Pts',(-37.2126332013933,8.41793088313261,0.));
#25598=CARTESIAN_POINT('Ctrl Pts',(-37.2126332013933,8.41793088313261,18.));
#25599=CARTESIAN_POINT('Ctrl Pts',(-37.1247207489179,8.38096706211448,0.));
#25600=CARTESIAN_POINT('Ctrl Pts',(-37.1247207489179,8.38096706211448,18.));
#25601=CARTESIAN_POINT('Ctrl Pts',(-37.0365602155148,8.3449081895264,0.));
#25602=CARTESIAN_POINT('Ctrl Pts',(-37.0365602155148,8.3449081895264,18.));
#25603=CARTESIAN_POINT('Ctrl Pts',(-36.9479311729484,8.31052547794592,0.));
#25604=CARTESIAN_POINT('Ctrl Pts',(-36.9479311729484,8.31052547794592,18.));
#25605=CARTESIAN_POINT('Ctrl Pts',(-36.8585291300917,8.27886599440785,0.));
#25606=CARTESIAN_POINT('Ctrl Pts',(-36.8585291300917,8.27886599440785,18.));
#25607=CARTESIAN_POINT('Ctrl Pts',(-36.7861403757604,8.25656657451821,0.));
#25608=CARTESIAN_POINT('Ctrl Pts',(-36.7861403757604,8.25656657451821,18.));
#25609=CARTESIAN_POINT('Ctrl Pts',(-36.7312504697652,8.24192165947368,0.));
#25610=CARTESIAN_POINT('Ctrl Pts',(-36.7312504697652,8.24192165947368,18.));
#25611=CARTESIAN_POINT('Ctrl Pts',(-36.6943771018148,8.23313075335377,0.));
#25612=CARTESIAN_POINT('Ctrl Pts',(-36.6943771018148,8.23313075335377,18.));
#25613=CARTESIAN_POINT('Ctrl Pts',(-36.6758703925241,8.22897839625061,0.));
#25614=CARTESIAN_POINT('Ctrl Pts',(-36.6758703925241,8.22897839625061,18.));
#25615=CARTESIAN_POINT('',(-42.2550026135057,12.2684454652017,0.));
#25616=CARTESIAN_POINT('Ctrl Pts',(-36.6758703925241,8.22897839625061,0.));
#25617=CARTESIAN_POINT('Ctrl Pts',(-36.6943771018148,8.23313075335377,0.));
#25618=CARTESIAN_POINT('Ctrl Pts',(-36.7312504697652,8.24192165947368,0.));
#25619=CARTESIAN_POINT('Ctrl Pts',(-36.7861403757604,8.25656657451821,0.));
#25620=CARTESIAN_POINT('Ctrl Pts',(-36.8585291300917,8.27886599440785,0.));
#25621=CARTESIAN_POINT('Ctrl Pts',(-36.9479311729484,8.31052547794592,0.));
#25622=CARTESIAN_POINT('Ctrl Pts',(-37.0365602155148,8.3449081895264,0.));
#25623=CARTESIAN_POINT('Ctrl Pts',(-37.1247207489179,8.38096706211448,0.));
#25624=CARTESIAN_POINT('Ctrl Pts',(-37.2126332013933,8.41793088313261,0.));
#25625=CARTESIAN_POINT('Ctrl Pts',(-37.3003733151561,8.4555084943396,0.));
#25626=CARTESIAN_POINT('Ctrl Pts',(-37.3879218093514,8.49372546467076,0.));
#25627=CARTESIAN_POINT('Ctrl Pts',(-37.4752030152968,8.53279758643785,0.));
#25628=CARTESIAN_POINT('Ctrl Pts',(-37.5621256752108,8.57299698459466,0.));
#25629=CARTESIAN_POINT('Ctrl Pts',(-37.6486274754754,8.61450621749155,0.));
#25630=CARTESIAN_POINT('Ctrl Pts',(-37.7347032383719,8.65732553894525,0.));
#25631=CARTESIAN_POINT('Ctrl Pts',(-37.8203816669031,8.70134776631143,0.));
#25632=CARTESIAN_POINT('Ctrl Pts',(-37.9057107230066,8.74640499479002,0.));
#25633=CARTESIAN_POINT('Ctrl Pts',(-37.9907407304174,8.79232279131092,0.));
#25634=CARTESIAN_POINT('Ctrl Pts',(-38.0755058326913,8.83897959763349,0.));
#25635=CARTESIAN_POINT('Ctrl Pts',(-38.1600150482528,8.88633535238434,0.));
#25636=CARTESIAN_POINT('Ctrl Pts',(-38.2442625706309,8.93439830996339,0.));
#25637=CARTESIAN_POINT('Ctrl Pts',(-38.3282340281403,8.9832048378576,0.));
#25638=CARTESIAN_POINT('Ctrl Pts',(-38.4119138099805,9.03279579360191,0.));
#25639=CARTESIAN_POINT('Ctrl Pts',(-38.4952932486131,9.08319014288086,0.));
#25640=CARTESIAN_POINT('Ctrl Pts',(-38.5783736628826,9.13437512010586,0.));
#25641=CARTESIAN_POINT('Ctrl Pts',(-38.6611620045193,9.1863201939433,0.));
#25642=CARTESIAN_POINT('Ctrl Pts',(-38.7436682576832,9.23898539199332,0.));
#25643=CARTESIAN_POINT('Ctrl Pts',(-38.8259023794241,9.29233110570903,0.));
#25644=CARTESIAN_POINT('Ctrl Pts',(-38.9078708427078,9.34632917154637,0.));
#25645=CARTESIAN_POINT('Ctrl Pts',(-38.9895756526779,9.40096600877644,0.));
#25646=CARTESIAN_POINT('Ctrl Pts',(-39.071016199495,9.45623664577432,0.));
#25647=CARTESIAN_POINT('Ctrl Pts',(-39.1521903958955,9.51214104535621,0.));
#25648=CARTESIAN_POINT('Ctrl Pts',(-39.2330959982788,9.56867984233623,0.));
#25649=CARTESIAN_POINT('Ctrl Pts',(-39.3137321153686,9.62584947846543,0.));
#25650=CARTESIAN_POINT('Ctrl Pts',(-39.3940995760289,9.68364100883827,0.));
#25651=CARTESIAN_POINT('Ctrl Pts',(-39.4742001555227,9.74204258152664,0.));
#25652=CARTESIAN_POINT('Ctrl Pts',(-39.5540361022309,9.80104095251614,0.));
#25653=CARTESIAN_POINT('Ctrl Pts',(-39.6336095893767,9.8606232424256,0.));
#25654=CARTESIAN_POINT('Ctrl Pts',(-39.712922089547,9.92077894513192,0.));
#25655=CARTESIAN_POINT('Ctrl Pts',(-39.7919742367922,9.98150036150823,0.));
#25656=CARTESIAN_POINT('Ctrl Pts',(-39.8707661565233,10.0427815229883,0.));
#25657=CARTESIAN_POINT('Ctrl Pts',(-39.9492976736738,10.1046175096878,0.));
#25658=CARTESIAN_POINT('Ctrl Pts',(-40.0275685525923,10.1670036683795,0.));
#25659=CARTESIAN_POINT('Ctrl Pts',(-40.1055787732578,10.2299347125857,0.));
#25660=CARTESIAN_POINT('Ctrl Pts',(-40.1833286010098,10.2934044990237,0.));
#25661=CARTESIAN_POINT('Ctrl Pts',(-40.2608184485326,10.3574064830678,0.));
#25662=CARTESIAN_POINT('Ctrl Pts',(-40.3380487942952,10.4219339932951,0.));
#25663=CARTESIAN_POINT('Ctrl Pts',(-40.4150200869536,10.48698054978,0.));
#25664=CARTESIAN_POINT('Ctrl Pts',(-40.4917326404439,10.5525402237951,0.));
#25665=CARTESIAN_POINT('Ctrl Pts',(-40.5681866012103,10.618607730849,0.));
#25666=CARTESIAN_POINT('Ctrl Pts',(-40.6443819999244,10.6851782157325,0.));
#25667=CARTESIAN_POINT('Ctrl Pts',(-40.7203187831783,10.7522471109694,0.));
#25668=CARTESIAN_POINT('Ctrl Pts',(-40.7959968527561,10.8198099757795,0.));
#25669=CARTESIAN_POINT('Ctrl Pts',(-40.8714161092412,10.8878623066646,0.));
#25670=CARTESIAN_POINT('Ctrl Pts',(-40.9465764747798,10.956399476781,0.));
#25671=CARTESIAN_POINT('Ctrl Pts',(-41.0214778832142,11.0254168609972,0.));
#25672=CARTESIAN_POINT('Ctrl Pts',(-41.0961202807715,11.0949099155251,0.));
#25673=CARTESIAN_POINT('Ctrl Pts',(-41.1705036228854,11.1648742640378,0.));
#25674=CARTESIAN_POINT('Ctrl Pts',(-41.2446278781981,11.2353057980338,0.));
#25675=CARTESIAN_POINT('Ctrl Pts',(-41.3184930194148,11.3062006993745,0.));
#25676=CARTESIAN_POINT('Ctrl Pts',(-41.3920989905986,11.3775553120176,0.));
#25677=CARTESIAN_POINT('Ctrl Pts',(-41.4654456796071,11.4493660393849,0.));
#25678=CARTESIAN_POINT('Ctrl Pts',(-41.5385328935506,11.5216292382388,0.));
#25679=CARTESIAN_POINT('Ctrl Pts',(-41.6113603270596,11.5943410868252,0.));
#25680=CARTESIAN_POINT('Ctrl Pts',(-41.6839275596248,11.6674975352852,0.));
#25681=CARTESIAN_POINT('Ctrl Pts',(-41.7562341395977,11.7410945211992,0.));
#25682=CARTESIAN_POINT('Ctrl Pts',(-41.8282796562569,11.81512813804,0.));
#25683=CARTESIAN_POINT('Ctrl Pts',(-41.9000638152266,11.8895948153349,0.));
#25684=CARTESIAN_POINT('Ctrl Pts',(-41.9715865222182,11.9644914999263,0.));
#25685=CARTESIAN_POINT('Ctrl Pts',(-42.0571002269437,12.054880669507,0.));
#25686=CARTESIAN_POINT('Ctrl Pts',(-42.1280354231517,12.1307372881904,0.));
#25687=CARTESIAN_POINT('Ctrl Pts',(-42.18457517013,12.1917619768791,0.));
#25688=CARTESIAN_POINT('Ctrl Pts',(-42.2268628664988,12.2377212115625,0.));
#25689=CARTESIAN_POINT('Ctrl Pts',(-42.2550026135057,12.2684454652018,0.));
#25690=CARTESIAN_POINT('',(-42.2550026135057,12.2684454652017,15.));
#25691=CARTESIAN_POINT('Ctrl Pts',(-42.2550026135057,12.2684454652018,15.));
#25692=CARTESIAN_POINT('Ctrl Pts',(-42.2409327400055,12.2530833383985,15.));
#25693=CARTESIAN_POINT('Ctrl Pts',(-42.2127669677092,12.222401466668,15.));
#25694=CARTESIAN_POINT('Ctrl Pts',(-42.1704402333854,12.1765058047069,15.));
#25695=CARTESIAN_POINT('Ctrl Pts',(-42.1138483839101,12.1155659644537,15.));
#25696=CARTESIAN_POINT('Ctrl Pts',(-42.0428479428228,12.0398158079102,15.));
#25697=CARTESIAN_POINT('Ctrl Pts',(-41.9715865222182,11.9644914999263,15.));
#25698=CARTESIAN_POINT('Ctrl Pts',(-41.9000638152266,11.8895948153349,15.));
#25699=CARTESIAN_POINT('Ctrl Pts',(-41.8282796562569,11.81512813804,15.));
#25700=CARTESIAN_POINT('Ctrl Pts',(-41.7562341395977,11.7410945211992,15.));
#25701=CARTESIAN_POINT('Ctrl Pts',(-41.6839275596248,11.6674975352852,15.));
#25702=CARTESIAN_POINT('Ctrl Pts',(-41.6113603270596,11.5943410868252,15.));
#25703=CARTESIAN_POINT('Ctrl Pts',(-41.5385328935506,11.5216292382388,15.));
#25704=CARTESIAN_POINT('Ctrl Pts',(-41.4654456796071,11.4493660393849,15.));
#25705=CARTESIAN_POINT('Ctrl Pts',(-41.3920989905986,11.3775553120176,15.));
#25706=CARTESIAN_POINT('Ctrl Pts',(-41.3184930194148,11.3062006993745,15.));
#25707=CARTESIAN_POINT('Ctrl Pts',(-41.2446278781981,11.2353057980338,15.));
#25708=CARTESIAN_POINT('Ctrl Pts',(-41.1705036228854,11.1648742640378,15.));
#25709=CARTESIAN_POINT('Ctrl Pts',(-41.0961202807715,11.0949099155251,15.));
#25710=CARTESIAN_POINT('Ctrl Pts',(-41.0214778832142,11.0254168609972,15.));
#25711=CARTESIAN_POINT('Ctrl Pts',(-40.9465764747798,10.956399476781,15.));
#25712=CARTESIAN_POINT('Ctrl Pts',(-40.8714161092412,10.8878623066646,15.));
#25713=CARTESIAN_POINT('Ctrl Pts',(-40.7959968527561,10.8198099757795,15.));
#25714=CARTESIAN_POINT('Ctrl Pts',(-40.7203187831783,10.7522471109694,15.));
#25715=CARTESIAN_POINT('Ctrl Pts',(-40.6443819999244,10.6851782157325,15.));
#25716=CARTESIAN_POINT('Ctrl Pts',(-40.5681866012103,10.618607730849,15.));
#25717=CARTESIAN_POINT('Ctrl Pts',(-40.4917326404439,10.5525402237951,15.));
#25718=CARTESIAN_POINT('Ctrl Pts',(-40.4150200869536,10.48698054978,15.));
#25719=CARTESIAN_POINT('Ctrl Pts',(-40.3380487942952,10.4219339932951,15.));
#25720=CARTESIAN_POINT('Ctrl Pts',(-40.2608184485326,10.3574064830678,15.));
#25721=CARTESIAN_POINT('Ctrl Pts',(-40.1833286010098,10.2934044990237,15.));
#25722=CARTESIAN_POINT('Ctrl Pts',(-40.1055787732578,10.2299347125857,15.));
#25723=CARTESIAN_POINT('Ctrl Pts',(-40.0275685525923,10.1670036683795,15.));
#25724=CARTESIAN_POINT('Ctrl Pts',(-39.9492976736738,10.1046175096878,15.));
#25725=CARTESIAN_POINT('Ctrl Pts',(-39.8707661565233,10.0427815229883,15.));
#25726=CARTESIAN_POINT('Ctrl Pts',(-39.7919742367922,9.98150036150823,15.));
#25727=CARTESIAN_POINT('Ctrl Pts',(-39.712922089547,9.92077894513192,15.));
#25728=CARTESIAN_POINT('Ctrl Pts',(-39.6336095893767,9.8606232424256,15.));
#25729=CARTESIAN_POINT('Ctrl Pts',(-39.5540361022309,9.80104095251614,15.));
#25730=CARTESIAN_POINT('Ctrl Pts',(-39.4742001555227,9.74204258152664,15.));
#25731=CARTESIAN_POINT('Ctrl Pts',(-39.3940995760289,9.68364100883827,15.));
#25732=CARTESIAN_POINT('Ctrl Pts',(-39.3137321153686,9.62584947846543,15.));
#25733=CARTESIAN_POINT('Ctrl Pts',(-39.2330959982788,9.56867984233623,15.));
#25734=CARTESIAN_POINT('Ctrl Pts',(-39.1521903958955,9.51214104535621,15.));
#25735=CARTESIAN_POINT('Ctrl Pts',(-39.071016199495,9.45623664577432,15.));
#25736=CARTESIAN_POINT('Ctrl Pts',(-38.9895756526779,9.40096600877644,15.));
#25737=CARTESIAN_POINT('Ctrl Pts',(-38.9078708427078,9.34632917154637,15.));
#25738=CARTESIAN_POINT('Ctrl Pts',(-38.8259023794241,9.29233110570903,15.));
#25739=CARTESIAN_POINT('Ctrl Pts',(-38.7436682576832,9.23898539199332,15.));
#25740=CARTESIAN_POINT('Ctrl Pts',(-38.6611620045193,9.1863201939433,15.));
#25741=CARTESIAN_POINT('Ctrl Pts',(-38.5783736628826,9.13437512010586,15.));
#25742=CARTESIAN_POINT('Ctrl Pts',(-38.4952932486131,9.08319014288086,15.));
#25743=CARTESIAN_POINT('Ctrl Pts',(-38.4119138099805,9.03279579360191,15.));
#25744=CARTESIAN_POINT('Ctrl Pts',(-38.3282340281403,8.9832048378576,15.));
#25745=CARTESIAN_POINT('Ctrl Pts',(-38.2442625706309,8.93439830996339,15.));
#25746=CARTESIAN_POINT('Ctrl Pts',(-38.1600150482528,8.88633535238434,15.));
#25747=CARTESIAN_POINT('Ctrl Pts',(-38.0755058326913,8.83897959763349,15.));
#25748=CARTESIAN_POINT('Ctrl Pts',(-37.9907407304174,8.79232279131092,15.));
#25749=CARTESIAN_POINT('Ctrl Pts',(-37.9057107230066,8.74640499479002,15.));
#25750=CARTESIAN_POINT('Ctrl Pts',(-37.8203816669031,8.70134776631143,15.));
#25751=CARTESIAN_POINT('Ctrl Pts',(-37.7347032383719,8.65732553894525,15.));
#25752=CARTESIAN_POINT('Ctrl Pts',(-37.6486274754754,8.61450621749155,15.));
#25753=CARTESIAN_POINT('Ctrl Pts',(-37.5621256752108,8.57299698459466,15.));
#25754=CARTESIAN_POINT('Ctrl Pts',(-37.4752030152968,8.53279758643785,15.));
#25755=CARTESIAN_POINT('Ctrl Pts',(-37.3879218093514,8.49372546467076,15.));
#25756=CARTESIAN_POINT('Ctrl Pts',(-37.3003733151561,8.4555084943396,15.));
#25757=CARTESIAN_POINT('Ctrl Pts',(-37.2126332013933,8.41793088313261,15.));
#25758=CARTESIAN_POINT('Ctrl Pts',(-37.1247207489179,8.38096706211448,15.));
#25759=CARTESIAN_POINT('Ctrl Pts',(-37.0365602155148,8.3449081895264,15.));
#25760=CARTESIAN_POINT('Ctrl Pts',(-36.9479311729484,8.31052547794592,15.));
#25761=CARTESIAN_POINT('Ctrl Pts',(-36.8585291300917,8.27886599440785,15.));
#25762=CARTESIAN_POINT('Ctrl Pts',(-36.7861403757604,8.25656657451821,15.));
#25763=CARTESIAN_POINT('Ctrl Pts',(-36.7312504697652,8.24192165947368,15.));
#25764=CARTESIAN_POINT('Ctrl Pts',(-36.6943771018148,8.23313075335377,15.));
#25765=CARTESIAN_POINT('Ctrl Pts',(-36.6758703925241,8.22897839625061,15.));
#25766=CARTESIAN_POINT('',(-42.2550026135057,12.2684454652017,0.));
#25767=CARTESIAN_POINT('Origin',(-1.07784724682657E-11,3.50213800024364E-12,
0.));
#25768=CARTESIAN_POINT('',(-41.396226524684,14.911486495888,0.));
#25769=CARTESIAN_POINT('Origin',(-1.07784724682657E-11,3.50213800024364E-12,
0.));
#25770=CARTESIAN_POINT('',(-41.396226524684,14.911486495888,15.));
#25771=CARTESIAN_POINT('Origin',(-1.07784724682657E-11,3.50213800024364E-12,
15.));
#25772=CARTESIAN_POINT('',(-41.396226524684,14.911486495888,0.));
#25773=CARTESIAN_POINT('Ctrl Pts',(-34.5082745737944,14.9001523628048,0.));
#25774=CARTESIAN_POINT('Ctrl Pts',(-34.5082745737944,14.9001523628048,18.));
#25775=CARTESIAN_POINT('Ctrl Pts',(-34.525687510388,14.9076710061311,0.));
#25776=CARTESIAN_POINT('Ctrl Pts',(-34.525687510388,14.9076710061311,18.));
#25777=CARTESIAN_POINT('Ctrl Pts',(-34.5606858566713,14.9222326355678,0.));
#25778=CARTESIAN_POINT('Ctrl Pts',(-34.5606858566713,14.9222326355678,18.));
#25779=CARTESIAN_POINT('Ctrl Pts',(-34.6137007885254,14.9426481276593,0.));
#25780=CARTESIAN_POINT('Ctrl Pts',(-34.6137007885254,14.9426481276593,18.));
#25781=CARTESIAN_POINT('Ctrl Pts',(-34.6853717911268,14.9671565602316,0.));
#25782=CARTESIAN_POINT('Ctrl Pts',(-34.6853717911268,14.9671565602316,18.));
#25783=CARTESIAN_POINT('Ctrl Pts',(-34.7763085406486,14.9940927023322,0.));
#25784=CARTESIAN_POINT('Ctrl Pts',(-34.7763085406486,14.9940927023322,18.));
#25785=CARTESIAN_POINT('Ctrl Pts',(-34.8682205930809,15.0183713484962,0.));
#25786=CARTESIAN_POINT('Ctrl Pts',(-34.8682205930809,15.0183713484962,18.));
#25787=CARTESIAN_POINT('Ctrl Pts',(-34.9607388363587,15.041018569143,0.));
#25788=CARTESIAN_POINT('Ctrl Pts',(-34.9607388363587,15.041018569143,18.));
#25789=CARTESIAN_POINT('Ctrl Pts',(-35.0535882932913,15.0627878528202,0.));
#25790=CARTESIAN_POINT('Ctrl Pts',(-35.0535882932913,15.0627878528202,18.));
#25791=CARTESIAN_POINT('Ctrl Pts',(-35.1466591020976,15.08395927165,0.));
#25792=CARTESIAN_POINT('Ctrl Pts',(-35.1466591020976,15.08395927165,18.));
#25793=CARTESIAN_POINT('Ctrl Pts',(-35.2399506932815,15.104500806927,0.));
#25794=CARTESIAN_POINT('Ctrl Pts',(-35.2399506932815,15.104500806927,18.));
#25795=CARTESIAN_POINT('Ctrl Pts',(-35.3335286891314,15.1241934020682,0.));
#25796=CARTESIAN_POINT('Ctrl Pts',(-35.3335286891314,15.1241934020682,18.));
#25797=CARTESIAN_POINT('Ctrl Pts',(-35.4274792115856,15.1427632633831,0.));
#25798=CARTESIAN_POINT('Ctrl Pts',(-35.4274792115856,15.1427632633831,18.));
#25799=CARTESIAN_POINT('Ctrl Pts',(-35.5218591529746,15.1600260710384,0.));
#25800=CARTESIAN_POINT('Ctrl Pts',(-35.5218591529746,15.1600260710384,18.));
#25801=CARTESIAN_POINT('Ctrl Pts',(-35.6166644736253,15.1759785763051,0.));
#25802=CARTESIAN_POINT('Ctrl Pts',(-35.6166644736253,15.1759785763051,18.));
#25803=CARTESIAN_POINT('Ctrl Pts',(-35.7118553943773,15.1907243629659,0.));
#25804=CARTESIAN_POINT('Ctrl Pts',(-35.7118553943773,15.1907243629659,18.));
#25805=CARTESIAN_POINT('Ctrl Pts',(-35.8073720252878,15.2044274601769,0.));
#25806=CARTESIAN_POINT('Ctrl Pts',(-35.8073720252878,15.2044274601769,18.));
#25807=CARTESIAN_POINT('Ctrl Pts',(-35.9031525499277,15.2172585668056,0.));
#25808=CARTESIAN_POINT('Ctrl Pts',(-35.9031525499277,15.2172585668056,18.));
#25809=CARTESIAN_POINT('Ctrl Pts',(-35.9991531408727,15.2293360946131,0.));
#25810=CARTESIAN_POINT('Ctrl Pts',(-35.9991531408727,15.2293360946131,18.));
#25811=CARTESIAN_POINT('Ctrl Pts',(-36.095357546697,15.240697754828,0.));
#25812=CARTESIAN_POINT('Ctrl Pts',(-36.095357546697,15.240697754828,18.));
#25813=CARTESIAN_POINT('Ctrl Pts',(-36.1917659216814,15.2513334565427,0.));
#25814=CARTESIAN_POINT('Ctrl Pts',(-36.1917659216814,15.2513334565427,18.));
#25815=CARTESIAN_POINT('Ctrl Pts',(-36.2883880151607,15.2612053303773,0.));
#25816=CARTESIAN_POINT('Ctrl Pts',(-36.2883880151607,15.2612053303773,18.));
#25817=CARTESIAN_POINT('Ctrl Pts',(-36.3852352131887,15.2702711460937,0.));
#25818=CARTESIAN_POINT('Ctrl Pts',(-36.3852352131887,15.2702711460937,18.));
#25819=CARTESIAN_POINT('Ctrl Pts',(-36.4823116513289,15.2785104654792,0.));
#25820=CARTESIAN_POINT('Ctrl Pts',(-36.4823116513289,15.2785104654792,18.));
#25821=CARTESIAN_POINT('Ctrl Pts',(-36.5796108931244,15.2859343913094,0.));
#25822=CARTESIAN_POINT('Ctrl Pts',(-36.5796108931244,15.2859343913094,18.));
#25823=CARTESIAN_POINT('Ctrl Pts',(-36.6771206167756,15.2925717100767,0.));
#25824=CARTESIAN_POINT('Ctrl Pts',(-36.6771206167756,15.2925717100767,18.));
#25825=CARTESIAN_POINT('Ctrl Pts',(-36.7748254044502,15.2984606286737,0.));
#25826=CARTESIAN_POINT('Ctrl Pts',(-36.7748254044502,15.2984606286737,18.));
#25827=CARTESIAN_POINT('Ctrl Pts',(-36.8727100302512,15.3036390436952,0.));
#25828=CARTESIAN_POINT('Ctrl Pts',(-36.8727100302512,15.3036390436952,18.));
#25829=CARTESIAN_POINT('Ctrl Pts',(-36.970763176802,15.3081335446406,0.));
#25830=CARTESIAN_POINT('Ctrl Pts',(-36.970763176802,15.3081335446406,18.));
#25831=CARTESIAN_POINT('Ctrl Pts',(-37.0689784837457,15.3119562971444,0.));
#25832=CARTESIAN_POINT('Ctrl Pts',(-37.0689784837457,15.3119562971444,18.));
#25833=CARTESIAN_POINT('Ctrl Pts',(-37.1673525354642,15.3151109648809,0.));
#25834=CARTESIAN_POINT('Ctrl Pts',(-37.1673525354642,15.3151109648809,18.));
#25835=CARTESIAN_POINT('Ctrl Pts',(-37.2658836214694,15.3175963510698,0.));
#25836=CARTESIAN_POINT('Ctrl Pts',(-37.2658836214694,15.3175963510698,18.));
#25837=CARTESIAN_POINT('Ctrl Pts',(-37.3645702997848,15.3194106233801,0.));
#25838=CARTESIAN_POINT('Ctrl Pts',(-37.3645702997848,15.3194106233801,18.));
#25839=CARTESIAN_POINT('Ctrl Pts',(-37.4634097578665,15.3205561366169,0.));
#25840=CARTESIAN_POINT('Ctrl Pts',(-37.4634097578665,15.3205561366169,18.));
#25841=CARTESIAN_POINT('Ctrl Pts',(-37.562397408596,15.3210406145546,0.));
#25842=CARTESIAN_POINT('Ctrl Pts',(-37.562397408596,15.3210406145546,18.));
#25843=CARTESIAN_POINT('Ctrl Pts',(-37.6615277218027,15.3208746890781,0.));
#25844=CARTESIAN_POINT('Ctrl Pts',(-37.6615277218027,15.3208746890781,18.));
#25845=CARTESIAN_POINT('Ctrl Pts',(-37.7607947318286,15.320070396385,0.));
#25846=CARTESIAN_POINT('Ctrl Pts',(-37.7607947318286,15.320070396385,18.));
#25847=CARTESIAN_POINT('Ctrl Pts',(-37.8601926265378,15.3186394335023,0.));
#25848=CARTESIAN_POINT('Ctrl Pts',(-37.8601926265378,15.3186394335023,18.));
#25849=CARTESIAN_POINT('Ctrl Pts',(-37.959716421934,15.3165911656268,0.));
#25850=CARTESIAN_POINT('Ctrl Pts',(-37.959716421934,15.3165911656268,18.));
#25851=CARTESIAN_POINT('Ctrl Pts',(-38.0593621055415,15.3139321941687,0.));
#25852=CARTESIAN_POINT('Ctrl Pts',(-38.0593621055415,15.3139321941687,18.));
#25853=CARTESIAN_POINT('Ctrl Pts',(-38.1591262705847,15.310667421514,0.));
#25854=CARTESIAN_POINT('Ctrl Pts',(-38.1591262705847,15.310667421514,18.));
#25855=CARTESIAN_POINT('Ctrl Pts',(-38.2590058835965,15.3068007250314,0.));
#25856=CARTESIAN_POINT('Ctrl Pts',(-38.2590058835965,15.3068007250314,18.));
#25857=CARTESIAN_POINT('Ctrl Pts',(-38.3589980188324,15.3023357307483,0.));
#25858=CARTESIAN_POINT('Ctrl Pts',(-38.3589980188324,15.3023357307483,18.));
#25859=CARTESIAN_POINT('Ctrl Pts',(-38.4590995527814,15.2972767037469,0.));
#25860=CARTESIAN_POINT('Ctrl Pts',(-38.4590995527814,15.2972767037469,18.));
#25861=CARTESIAN_POINT('Ctrl Pts',(-38.5593070891769,15.2916287700102,0.));
#25862=CARTESIAN_POINT('Ctrl Pts',(-38.5593070891769,15.2916287700102,18.));
#25863=CARTESIAN_POINT('Ctrl Pts',(-38.659617115053,15.2853974668211,0.));
#25864=CARTESIAN_POINT('Ctrl Pts',(-38.659617115053,15.2853974668211,18.));
#25865=CARTESIAN_POINT('Ctrl Pts',(-38.7600260961351,15.2785884727112,0.));
#25866=CARTESIAN_POINT('Ctrl Pts',(-38.7600260961351,15.2785884727112,18.));
#25867=CARTESIAN_POINT('Ctrl Pts',(-38.860530586589,15.2712072937639,0.));
#25868=CARTESIAN_POINT('Ctrl Pts',(-38.860530586589,15.2712072937639,18.));
#25869=CARTESIAN_POINT('Ctrl Pts',(-38.9611273555758,15.2632589109473,0.));
#25870=CARTESIAN_POINT('Ctrl Pts',(-38.9611273555758,15.2632589109473,18.));
#25871=CARTESIAN_POINT('Ctrl Pts',(-39.061813415425,15.2547476855825,0.));
#25872=CARTESIAN_POINT('Ctrl Pts',(-39.061813415425,15.2547476855825,18.));
#25873=CARTESIAN_POINT('Ctrl Pts',(-39.1625859371304,15.2456775636447,0.));
#25874=CARTESIAN_POINT('Ctrl Pts',(-39.1625859371304,15.2456775636447,18.));
#25875=CARTESIAN_POINT('Ctrl Pts',(-39.2634421927888,15.2360522089072,0.));
#25876=CARTESIAN_POINT('Ctrl Pts',(-39.2634421927888,15.2360522089072,18.));
#25877=CARTESIAN_POINT('Ctrl Pts',(-39.3643794927167,15.225875156307,0.));
#25878=CARTESIAN_POINT('Ctrl Pts',(-39.3643794927167,15.225875156307,18.));
#25879=CARTESIAN_POINT('Ctrl Pts',(-39.4653951093947,15.2151499908149,0.));
#25880=CARTESIAN_POINT('Ctrl Pts',(-39.4653951093947,15.2151499908149,18.));
#25881=CARTESIAN_POINT('Ctrl Pts',(-39.5664862602472,15.2038804098649,0.));
#25882=CARTESIAN_POINT('Ctrl Pts',(-39.5664862602472,15.2038804098649,18.));
#25883=CARTESIAN_POINT('Ctrl Pts',(-39.6676501731673,15.1920701163803,0.));
#25884=CARTESIAN_POINT('Ctrl Pts',(-39.6676501731673,15.1920701163803,18.));
#25885=CARTESIAN_POINT('Ctrl Pts',(-39.7688841338802,15.1797227547562,0.));
#25886=CARTESIAN_POINT('Ctrl Pts',(-39.7688841338802,15.1797227547562,18.));
#25887=CARTESIAN_POINT('Ctrl Pts',(-39.8701855339908,15.1668418393198,0.));
#25888=CARTESIAN_POINT('Ctrl Pts',(-39.8701855339908,15.1668418393198,18.));
#25889=CARTESIAN_POINT('Ctrl Pts',(-39.9715519332134,15.1534306754871,0.));
#25890=CARTESIAN_POINT('Ctrl Pts',(-39.9715519332134,15.1534306754871,18.));
#25891=CARTESIAN_POINT('Ctrl Pts',(-40.0729810652204,15.1394923361537,0.));
#25892=CARTESIAN_POINT('Ctrl Pts',(-40.0729810652204,15.1394923361537,18.));
#25893=CARTESIAN_POINT('Ctrl Pts',(-40.1744707357902,15.1250297462408,0.));
#25894=CARTESIAN_POINT('Ctrl Pts',(-40.1744707357902,15.1250297462408,18.));
#25895=CARTESIAN_POINT('Ctrl Pts',(-40.2760187401822,15.1100457495259,0.));
#25896=CARTESIAN_POINT('Ctrl Pts',(-40.2760187401822,15.1100457495259,18.));
#25897=CARTESIAN_POINT('Ctrl Pts',(-40.3776227809037,15.0945431800723,0.));
#25898=CARTESIAN_POINT('Ctrl Pts',(-40.3776227809037,15.0945431800723,18.));
#25899=CARTESIAN_POINT('Ctrl Pts',(-40.4792803645352,15.0785249502524,0.));
#25900=CARTESIAN_POINT('Ctrl Pts',(-40.4792803645352,15.0785249502524,18.));
#25901=CARTESIAN_POINT('Ctrl Pts',(-40.58098877043,15.0619940893017,0.));
#25902=CARTESIAN_POINT('Ctrl Pts',(-40.58098877043,15.0619940893017,18.));
#25903=CARTESIAN_POINT('Ctrl Pts',(-40.6827452453667,15.0449536183143,0.));
#25904=CARTESIAN_POINT('Ctrl Pts',(-40.6827452453667,15.0449536183143,18.));
#25905=CARTESIAN_POINT('Ctrl Pts',(-40.7845471608654,15.0274064563211,0.));
#25906=CARTESIAN_POINT('Ctrl Pts',(-40.7845471608654,15.0274064563211,18.));
#25907=CARTESIAN_POINT('Ctrl Pts',(-40.8863921801,15.0093553188655,0.));
#25908=CARTESIAN_POINT('Ctrl Pts',(-40.8863921801,15.0093553188655,18.));
#25909=CARTESIAN_POINT('Ctrl Pts',(-40.9882784321884,14.9908026205824,0.));
#25910=CARTESIAN_POINT('Ctrl Pts',(-40.9882784321884,14.9908026205824,18.));
#25911=CARTESIAN_POINT('Ctrl Pts',(-41.0902046498729,14.9717503874227,0.));
#25912=CARTESIAN_POINT('Ctrl Pts',(-41.0902046498729,14.9717503874227,18.));
#25913=CARTESIAN_POINT('Ctrl Pts',(-41.1921700381957,14.9522002356298,0.));
#25914=CARTESIAN_POINT('Ctrl Pts',(-41.1921700381957,14.9522002356298,18.));
#25915=CARTESIAN_POINT('Ctrl Pts',(-41.2737733455422,14.936162723752,0.));
#25916=CARTESIAN_POINT('Ctrl Pts',(-41.2737733455422,14.936162723752,18.));
#25917=CARTESIAN_POINT('Ctrl Pts',(-41.3349931861715,14.9239113834707,0.));
#25918=CARTESIAN_POINT('Ctrl Pts',(-41.3349931861715,14.9239113834707,18.));
#25919=CARTESIAN_POINT('Ctrl Pts',(-41.3758141263348,14.9156446533966,0.));
#25920=CARTESIAN_POINT('Ctrl Pts',(-41.3758141263348,14.9156446533966,18.));
#25921=CARTESIAN_POINT('Ctrl Pts',(-41.396226524684,14.911486495888,0.));
#25922=CARTESIAN_POINT('Ctrl Pts',(-41.396226524684,14.911486495888,18.));
#25923=CARTESIAN_POINT('Ctrl Pts',(-34.5082745737944,14.9001523628048,0.));
#25924=CARTESIAN_POINT('Ctrl Pts',(-34.525687510388,14.9076710061311,0.));
#25925=CARTESIAN_POINT('Ctrl Pts',(-34.5606858566713,14.9222326355678,0.));
#25926=CARTESIAN_POINT('Ctrl Pts',(-34.6137007885254,14.9426481276593,0.));
#25927=CARTESIAN_POINT('Ctrl Pts',(-34.6853717911268,14.9671565602316,0.));
#25928=CARTESIAN_POINT('Ctrl Pts',(-34.7763085406486,14.9940927023322,0.));
#25929=CARTESIAN_POINT('Ctrl Pts',(-34.8682205930809,15.0183713484962,0.));
#25930=CARTESIAN_POINT('Ctrl Pts',(-34.9607388363587,15.041018569143,0.));
#25931=CARTESIAN_POINT('Ctrl Pts',(-35.0535882932913,15.0627878528202,0.));
#25932=CARTESIAN_POINT('Ctrl Pts',(-35.1466591020976,15.08395927165,0.));
#25933=CARTESIAN_POINT('Ctrl Pts',(-35.2399506932815,15.104500806927,0.));
#25934=CARTESIAN_POINT('Ctrl Pts',(-35.3335286891314,15.1241934020682,0.));
#25935=CARTESIAN_POINT('Ctrl Pts',(-35.4274792115856,15.1427632633831,0.));
#25936=CARTESIAN_POINT('Ctrl Pts',(-35.5218591529746,15.1600260710384,0.));
#25937=CARTESIAN_POINT('Ctrl Pts',(-35.6166644736253,15.1759785763051,0.));
#25938=CARTESIAN_POINT('Ctrl Pts',(-35.7118553943773,15.1907243629659,0.));
#25939=CARTESIAN_POINT('Ctrl Pts',(-35.8073720252878,15.2044274601769,0.));
#25940=CARTESIAN_POINT('Ctrl Pts',(-35.9031525499277,15.2172585668056,0.));
#25941=CARTESIAN_POINT('Ctrl Pts',(-35.9991531408727,15.2293360946131,0.));
#25942=CARTESIAN_POINT('Ctrl Pts',(-36.095357546697,15.240697754828,0.));
#25943=CARTESIAN_POINT('Ctrl Pts',(-36.1917659216814,15.2513334565427,0.));
#25944=CARTESIAN_POINT('Ctrl Pts',(-36.2883880151607,15.2612053303773,0.));
#25945=CARTESIAN_POINT('Ctrl Pts',(-36.3852352131887,15.2702711460937,0.));
#25946=CARTESIAN_POINT('Ctrl Pts',(-36.4823116513289,15.2785104654792,0.));
#25947=CARTESIAN_POINT('Ctrl Pts',(-36.5796108931244,15.2859343913094,0.));
#25948=CARTESIAN_POINT('Ctrl Pts',(-36.6771206167756,15.2925717100767,0.));
#25949=CARTESIAN_POINT('Ctrl Pts',(-36.7748254044502,15.2984606286737,0.));
#25950=CARTESIAN_POINT('Ctrl Pts',(-36.8727100302512,15.3036390436952,0.));
#25951=CARTESIAN_POINT('Ctrl Pts',(-36.970763176802,15.3081335446406,0.));
#25952=CARTESIAN_POINT('Ctrl Pts',(-37.0689784837457,15.3119562971444,0.));
#25953=CARTESIAN_POINT('Ctrl Pts',(-37.1673525354642,15.3151109648809,0.));
#25954=CARTESIAN_POINT('Ctrl Pts',(-37.2658836214694,15.3175963510698,0.));
#25955=CARTESIAN_POINT('Ctrl Pts',(-37.3645702997848,15.3194106233801,0.));
#25956=CARTESIAN_POINT('Ctrl Pts',(-37.4634097578665,15.3205561366169,0.));
#25957=CARTESIAN_POINT('Ctrl Pts',(-37.562397408596,15.3210406145546,0.));
#25958=CARTESIAN_POINT('Ctrl Pts',(-37.6615277218027,15.3208746890781,0.));
#25959=CARTESIAN_POINT('Ctrl Pts',(-37.7607947318286,15.320070396385,0.));
#25960=CARTESIAN_POINT('Ctrl Pts',(-37.8601926265378,15.3186394335023,0.));
#25961=CARTESIAN_POINT('Ctrl Pts',(-37.959716421934,15.3165911656268,0.));
#25962=CARTESIAN_POINT('Ctrl Pts',(-38.0593621055415,15.3139321941687,0.));
#25963=CARTESIAN_POINT('Ctrl Pts',(-38.1591262705847,15.310667421514,0.));
#25964=CARTESIAN_POINT('Ctrl Pts',(-38.2590058835965,15.3068007250314,0.));
#25965=CARTESIAN_POINT('Ctrl Pts',(-38.3589980188324,15.3023357307483,0.));
#25966=CARTESIAN_POINT('Ctrl Pts',(-38.4590995527814,15.2972767037469,0.));
#25967=CARTESIAN_POINT('Ctrl Pts',(-38.5593070891769,15.2916287700102,0.));
#25968=CARTESIAN_POINT('Ctrl Pts',(-38.659617115053,15.2853974668211,0.));
#25969=CARTESIAN_POINT('Ctrl Pts',(-38.7600260961351,15.2785884727112,0.));
#25970=CARTESIAN_POINT('Ctrl Pts',(-38.860530586589,15.2712072937639,0.));
#25971=CARTESIAN_POINT('Ctrl Pts',(-38.9611273555758,15.2632589109473,0.));
#25972=CARTESIAN_POINT('Ctrl Pts',(-39.061813415425,15.2547476855825,0.));
#25973=CARTESIAN_POINT('Ctrl Pts',(-39.1625859371304,15.2456775636447,0.));
#25974=CARTESIAN_POINT('Ctrl Pts',(-39.2634421927888,15.2360522089072,0.));
#25975=CARTESIAN_POINT('Ctrl Pts',(-39.3643794927167,15.225875156307,0.));
#25976=CARTESIAN_POINT('Ctrl Pts',(-39.4653951093947,15.2151499908149,0.));
#25977=CARTESIAN_POINT('Ctrl Pts',(-39.5664862602472,15.2038804098649,0.));
#25978=CARTESIAN_POINT('Ctrl Pts',(-39.6676501731673,15.1920701163803,0.));
#25979=CARTESIAN_POINT('Ctrl Pts',(-39.7688841338802,15.1797227547562,0.));
#25980=CARTESIAN_POINT('Ctrl Pts',(-39.8701855339908,15.1668418393198,0.));
#25981=CARTESIAN_POINT('Ctrl Pts',(-39.9715519332134,15.1534306754871,0.));
#25982=CARTESIAN_POINT('Ctrl Pts',(-40.0729810652204,15.1394923361537,0.));
#25983=CARTESIAN_POINT('Ctrl Pts',(-40.1744707357902,15.1250297462408,0.));
#25984=CARTESIAN_POINT('Ctrl Pts',(-40.2760187401822,15.1100457495259,0.));
#25985=CARTESIAN_POINT('Ctrl Pts',(-40.3776227809037,15.0945431800723,0.));
#25986=CARTESIAN_POINT('Ctrl Pts',(-40.4792803645352,15.0785249502524,0.));
#25987=CARTESIAN_POINT('Ctrl Pts',(-40.58098877043,15.0619940893017,0.));
#25988=CARTESIAN_POINT('Ctrl Pts',(-40.6827452453667,15.0449536183143,0.));
#25989=CARTESIAN_POINT('Ctrl Pts',(-40.7845471608654,15.0274064563211,0.));
#25990=CARTESIAN_POINT('Ctrl Pts',(-40.8863921801,15.0093553188655,0.));
#25991=CARTESIAN_POINT('Ctrl Pts',(-40.9882784321884,14.9908026205824,0.));
#25992=CARTESIAN_POINT('Ctrl Pts',(-41.1105898934098,14.9679399407908,0.));
#25993=CARTESIAN_POINT('Ctrl Pts',(-41.2125650743922,14.9482653093396,0.));
#25994=CARTESIAN_POINT('Ctrl Pts',(-41.2941761025922,14.9321285285561,0.));
#25995=CARTESIAN_POINT('Ctrl Pts',(-41.3554017279611,14.919802810928,0.));
#25996=CARTESIAN_POINT('Ctrl Pts',(-41.396226524684,14.911486495888,0.));
#25997=CARTESIAN_POINT('Ctrl Pts',(-34.5082745737944,14.9001523628048,15.));
#25998=CARTESIAN_POINT('Ctrl Pts',(-34.525687510388,14.9076710061311,15.));
#25999=CARTESIAN_POINT('Ctrl Pts',(-34.5606858566713,14.9222326355678,15.));
#26000=CARTESIAN_POINT('Ctrl Pts',(-34.6137007885254,14.9426481276593,15.));
#26001=CARTESIAN_POINT('Ctrl Pts',(-34.6853717911268,14.9671565602316,15.));
#26002=CARTESIAN_POINT('Ctrl Pts',(-34.7763085406486,14.9940927023322,15.));
#26003=CARTESIAN_POINT('Ctrl Pts',(-34.8682205930809,15.0183713484962,15.));
#26004=CARTESIAN_POINT('Ctrl Pts',(-34.9607388363587,15.041018569143,15.));
#26005=CARTESIAN_POINT('Ctrl Pts',(-35.0535882932913,15.0627878528202,15.));
#26006=CARTESIAN_POINT('Ctrl Pts',(-35.1466591020976,15.08395927165,15.));
#26007=CARTESIAN_POINT('Ctrl Pts',(-35.2399506932815,15.104500806927,15.));
#26008=CARTESIAN_POINT('Ctrl Pts',(-35.3335286891314,15.1241934020682,15.));
#26009=CARTESIAN_POINT('Ctrl Pts',(-35.4274792115856,15.1427632633831,15.));
#26010=CARTESIAN_POINT('Ctrl Pts',(-35.5218591529746,15.1600260710384,15.));
#26011=CARTESIAN_POINT('Ctrl Pts',(-35.6166644736253,15.1759785763051,15.));
#26012=CARTESIAN_POINT('Ctrl Pts',(-35.7118553943773,15.1907243629659,15.));
#26013=CARTESIAN_POINT('Ctrl Pts',(-35.8073720252878,15.2044274601769,15.));
#26014=CARTESIAN_POINT('Ctrl Pts',(-35.9031525499277,15.2172585668056,15.));
#26015=CARTESIAN_POINT('Ctrl Pts',(-35.9991531408727,15.2293360946131,15.));
#26016=CARTESIAN_POINT('Ctrl Pts',(-36.095357546697,15.240697754828,15.));
#26017=CARTESIAN_POINT('Ctrl Pts',(-36.1917659216814,15.2513334565427,15.));
#26018=CARTESIAN_POINT('Ctrl Pts',(-36.2883880151607,15.2612053303773,15.));
#26019=CARTESIAN_POINT('Ctrl Pts',(-36.3852352131887,15.2702711460937,15.));
#26020=CARTESIAN_POINT('Ctrl Pts',(-36.4823116513289,15.2785104654792,15.));
#26021=CARTESIAN_POINT('Ctrl Pts',(-36.5796108931244,15.2859343913094,15.));
#26022=CARTESIAN_POINT('Ctrl Pts',(-36.6771206167756,15.2925717100767,15.));
#26023=CARTESIAN_POINT('Ctrl Pts',(-36.7748254044502,15.2984606286737,15.));
#26024=CARTESIAN_POINT('Ctrl Pts',(-36.8727100302512,15.3036390436952,15.));
#26025=CARTESIAN_POINT('Ctrl Pts',(-36.970763176802,15.3081335446406,15.));
#26026=CARTESIAN_POINT('Ctrl Pts',(-37.0689784837457,15.3119562971444,15.));
#26027=CARTESIAN_POINT('Ctrl Pts',(-37.1673525354642,15.3151109648809,15.));
#26028=CARTESIAN_POINT('Ctrl Pts',(-37.2658836214694,15.3175963510698,15.));
#26029=CARTESIAN_POINT('Ctrl Pts',(-37.3645702997848,15.3194106233801,15.));
#26030=CARTESIAN_POINT('Ctrl Pts',(-37.4634097578665,15.3205561366169,15.));
#26031=CARTESIAN_POINT('Ctrl Pts',(-37.562397408596,15.3210406145546,15.));
#26032=CARTESIAN_POINT('Ctrl Pts',(-37.6615277218027,15.3208746890781,15.));
#26033=CARTESIAN_POINT('Ctrl Pts',(-37.7607947318286,15.320070396385,15.));
#26034=CARTESIAN_POINT('Ctrl Pts',(-37.8601926265378,15.3186394335023,15.));
#26035=CARTESIAN_POINT('Ctrl Pts',(-37.959716421934,15.3165911656268,15.));
#26036=CARTESIAN_POINT('Ctrl Pts',(-38.0593621055415,15.3139321941687,15.));
#26037=CARTESIAN_POINT('Ctrl Pts',(-38.1591262705847,15.310667421514,15.));
#26038=CARTESIAN_POINT('Ctrl Pts',(-38.2590058835965,15.3068007250314,15.));
#26039=CARTESIAN_POINT('Ctrl Pts',(-38.3589980188324,15.3023357307483,15.));
#26040=CARTESIAN_POINT('Ctrl Pts',(-38.4590995527814,15.2972767037469,15.));
#26041=CARTESIAN_POINT('Ctrl Pts',(-38.5593070891769,15.2916287700102,15.));
#26042=CARTESIAN_POINT('Ctrl Pts',(-38.659617115053,15.2853974668211,15.));
#26043=CARTESIAN_POINT('Ctrl Pts',(-38.7600260961351,15.2785884727112,15.));
#26044=CARTESIAN_POINT('Ctrl Pts',(-38.860530586589,15.2712072937639,15.));
#26045=CARTESIAN_POINT('Ctrl Pts',(-38.9611273555758,15.2632589109473,15.));
#26046=CARTESIAN_POINT('Ctrl Pts',(-39.061813415425,15.2547476855825,15.));
#26047=CARTESIAN_POINT('Ctrl Pts',(-39.1625859371304,15.2456775636447,15.));
#26048=CARTESIAN_POINT('Ctrl Pts',(-39.2634421927888,15.2360522089072,15.));
#26049=CARTESIAN_POINT('Ctrl Pts',(-39.3643794927167,15.225875156307,15.));
#26050=CARTESIAN_POINT('Ctrl Pts',(-39.4653951093947,15.2151499908149,15.));
#26051=CARTESIAN_POINT('Ctrl Pts',(-39.5664862602472,15.2038804098649,15.));
#26052=CARTESIAN_POINT('Ctrl Pts',(-39.6676501731673,15.1920701163803,15.));
#26053=CARTESIAN_POINT('Ctrl Pts',(-39.7688841338802,15.1797227547562,15.));
#26054=CARTESIAN_POINT('Ctrl Pts',(-39.8701855339908,15.1668418393198,15.));
#26055=CARTESIAN_POINT('Ctrl Pts',(-39.9715519332134,15.1534306754871,15.));
#26056=CARTESIAN_POINT('Ctrl Pts',(-40.0729810652204,15.1394923361537,15.));
#26057=CARTESIAN_POINT('Ctrl Pts',(-40.1744707357902,15.1250297462408,15.));
#26058=CARTESIAN_POINT('Ctrl Pts',(-40.2760187401822,15.1100457495259,15.));
#26059=CARTESIAN_POINT('Ctrl Pts',(-40.3776227809037,15.0945431800723,15.));
#26060=CARTESIAN_POINT('Ctrl Pts',(-40.4792803645352,15.0785249502524,15.));
#26061=CARTESIAN_POINT('Ctrl Pts',(-40.58098877043,15.0619940893017,15.));
#26062=CARTESIAN_POINT('Ctrl Pts',(-40.6827452453667,15.0449536183143,15.));
#26063=CARTESIAN_POINT('Ctrl Pts',(-40.7845471608654,15.0274064563211,15.));
#26064=CARTESIAN_POINT('Ctrl Pts',(-40.8863921801,15.0093553188655,15.));
#26065=CARTESIAN_POINT('Ctrl Pts',(-40.9882784321884,14.9908026205824,15.));
#26066=CARTESIAN_POINT('Ctrl Pts',(-41.1105898934098,14.9679399407908,15.));
#26067=CARTESIAN_POINT('Ctrl Pts',(-41.2125650743922,14.9482653093396,15.));
#26068=CARTESIAN_POINT('Ctrl Pts',(-41.2941761025922,14.9321285285561,15.));
#26069=CARTESIAN_POINT('Ctrl Pts',(-41.3554017279611,14.919802810928,15.));
#26070=CARTESIAN_POINT('Ctrl Pts',(-41.396226524684,14.911486495888,15.));
#26071=CARTESIAN_POINT('Ctrl Pts',(-36.3957374383337,24.725498909423,0.));
#26072=CARTESIAN_POINT('Ctrl Pts',(-36.3957374383337,24.725498909423,18.));
#26073=CARTESIAN_POINT('Ctrl Pts',(-36.3871033517098,24.7065408286023,0.));
#26074=CARTESIAN_POINT('Ctrl Pts',(-36.3871033517098,24.7065408286023,18.));
#26075=CARTESIAN_POINT('Ctrl Pts',(-36.369797330215,24.6686569322616,0.));
#26076=CARTESIAN_POINT('Ctrl Pts',(-36.369797330215,24.6686569322616,18.));
#26077=CARTESIAN_POINT('Ctrl Pts',(-36.3437247532368,24.6119278836614,0.));
#26078=CARTESIAN_POINT('Ctrl Pts',(-36.3437247532368,24.6119278836614,18.));
#26079=CARTESIAN_POINT('Ctrl Pts',(-36.3087341522969,24.5364828082556,0.));
#26080=CARTESIAN_POINT('Ctrl Pts',(-36.3087341522969,24.5364828082556,18.));
#26081=CARTESIAN_POINT('Ctrl Pts',(-36.2646168058395,24.4424997853605,0.));
#26082=CARTESIAN_POINT('Ctrl Pts',(-36.2646168058395,24.4424997853605,18.));
#26083=CARTESIAN_POINT('Ctrl Pts',(-36.2201196586696,24.3488411214068,0.));
#26084=CARTESIAN_POINT('Ctrl Pts',(-36.2201196586696,24.3488411214068,18.));
#26085=CARTESIAN_POINT('Ctrl Pts',(-36.1752418704833,24.2555084095332,0.));
#26086=CARTESIAN_POINT('Ctrl Pts',(-36.1752418704833,24.2555084095332,18.));
#26087=CARTESIAN_POINT('Ctrl Pts',(-36.1299825471271,24.1625038657964,0.));
#26088=CARTESIAN_POINT('Ctrl Pts',(-36.1299825471271,24.1625038657964,18.));
#26089=CARTESIAN_POINT('Ctrl Pts',(-36.0843408347974,24.0698304230588,0.));
#26090=CARTESIAN_POINT('Ctrl Pts',(-36.0843408347974,24.0698304230588,18.));
#26091=CARTESIAN_POINT('Ctrl Pts',(-36.0383159101253,23.9774915680089,0.));
#26092=CARTESIAN_POINT('Ctrl Pts',(-36.0383159101253,23.9774915680089,18.));
#26093=CARTESIAN_POINT('Ctrl Pts',(-35.9919069565469,23.8854911428946,0.));
#26094=CARTESIAN_POINT('Ctrl Pts',(-35.9919069565469,23.8854911428946,18.));
#26095=CARTESIAN_POINT('Ctrl Pts',(-35.9451131482488,23.7938331508737,0.));
#26096=CARTESIAN_POINT('Ctrl Pts',(-35.9451131482488,23.7938331508737,18.));
#26097=CARTESIAN_POINT('Ctrl Pts',(-35.8979336336837,23.7025215735353,0.));
#26098=CARTESIAN_POINT('Ctrl Pts',(-35.8979336336837,23.7025215735353,18.));
#26099=CARTESIAN_POINT('Ctrl Pts',(-35.8503675222885,23.611560139948,0.));
#26100=CARTESIAN_POINT('Ctrl Pts',(-35.8503675222885,23.611560139948,18.));
#26101=CARTESIAN_POINT('Ctrl Pts',(-35.8024138716896,23.5209523746427,0.));
#26102=CARTESIAN_POINT('Ctrl Pts',(-35.8024138716896,23.5209523746427,18.));
#26103=CARTESIAN_POINT('Ctrl Pts',(-35.7540716771372,23.4307017328227,0.));
#26104=CARTESIAN_POINT('Ctrl Pts',(-35.7540716771372,23.4307017328227,18.));
#26105=CARTESIAN_POINT('Ctrl Pts',(-35.7053398620512,23.3408117088762,0.));
#26106=CARTESIAN_POINT('Ctrl Pts',(-35.7053398620512,23.3408117088762,18.));
#26107=CARTESIAN_POINT('Ctrl Pts',(-35.6562172725207,23.2512859425032,0.));
#26108=CARTESIAN_POINT('Ctrl Pts',(-35.6562172725207,23.2512859425032,18.));
#26109=CARTESIAN_POINT('Ctrl Pts',(-35.6067026687722,23.1621283508111,0.));
#26110=CARTESIAN_POINT('Ctrl Pts',(-35.6067026687722,23.1621283508111,18.));
#26111=CARTESIAN_POINT('Ctrl Pts',(-35.5567947408311,23.0733431097058,0.));
#26112=CARTESIAN_POINT('Ctrl Pts',(-35.5567947408311,23.0733431097058,18.));
#26113=CARTESIAN_POINT('Ctrl Pts',(-35.5064921357308,22.9849345572033,0.));
#26114=CARTESIAN_POINT('Ctrl Pts',(-35.5064921357308,22.9849345572033,18.));
#26115=CARTESIAN_POINT('Ctrl Pts',(-35.4557934871468,22.8969071125089,0.));
#26116=CARTESIAN_POINT('Ctrl Pts',(-35.4557934871468,22.8969071125089,18.));
#26117=CARTESIAN_POINT('Ctrl Pts',(-35.4046974393492,22.8092652000706,0.));
#26118=CARTESIAN_POINT('Ctrl Pts',(-35.4046974393492,22.8092652000706,18.));
#26119=CARTESIAN_POINT('Ctrl Pts',(-35.3532026952313,22.7220131336912,0.));
#26120=CARTESIAN_POINT('Ctrl Pts',(-35.3532026952313,22.7220131336912,18.));
#26121=CARTESIAN_POINT('Ctrl Pts',(-35.3013079759252,22.635155167154,0.));
#26122=CARTESIAN_POINT('Ctrl Pts',(-35.3013079759252,22.635155167154,18.));
#26123=CARTESIAN_POINT('Ctrl Pts',(-35.2490119207975,22.5486956608909,0.));
#26124=CARTESIAN_POINT('Ctrl Pts',(-35.2490119207975,22.5486956608909,18.));
#26125=CARTESIAN_POINT('Ctrl Pts',(-35.1963130003352,22.4626392230023,0.));
#26126=CARTESIAN_POINT('Ctrl Pts',(-35.1963130003352,22.4626392230023,18.));
#26127=CARTESIAN_POINT('Ctrl Pts',(-35.1432094422642,22.3769908340843,0.));
#26128=CARTESIAN_POINT('Ctrl Pts',(-35.1432094422642,22.3769908340843,18.));
#26129=CARTESIAN_POINT('Ctrl Pts',(-35.0896991159359,22.2917560356803,0.));
#26130=CARTESIAN_POINT('Ctrl Pts',(-35.0896991159359,22.2917560356803,18.));
#26131=CARTESIAN_POINT('Ctrl Pts',(-35.0357795922459,22.2069408519233,0.));
#26132=CARTESIAN_POINT('Ctrl Pts',(-35.0357795922459,22.2069408519233,18.));
#26133=CARTESIAN_POINT('Ctrl Pts',(-34.9814483545602,22.1225514798584,0.));
#26134=CARTESIAN_POINT('Ctrl Pts',(-34.9814483545602,22.1225514798584,18.));
#26135=CARTESIAN_POINT('Ctrl Pts',(-34.9267029879922,22.0385940162683,0.));
#26136=CARTESIAN_POINT('Ctrl Pts',(-34.9267029879922,22.0385940162683,18.));
#26137=CARTESIAN_POINT('Ctrl Pts',(-34.8715413418101,21.9550742217675,0.));
#26138=CARTESIAN_POINT('Ctrl Pts',(-34.8715413418101,21.9550742217675,18.));
#26139=CARTESIAN_POINT('Ctrl Pts',(-34.8159618014436,21.8719971302817,0.));
#26140=CARTESIAN_POINT('Ctrl Pts',(-34.8159618014436,21.8719971302817,18.));
#26141=CARTESIAN_POINT('Ctrl Pts',(-34.7599631530844,21.7893672401137,0.));
#26142=CARTESIAN_POINT('Ctrl Pts',(-34.7599631530844,21.7893672401137,18.));
#26143=CARTESIAN_POINT('Ctrl Pts',(-34.7035440429025,21.7071892844497,0.));
#26144=CARTESIAN_POINT('Ctrl Pts',(-34.7035440429025,21.7071892844497,18.));
#26145=CARTESIAN_POINT('Ctrl Pts',(-34.6467025072367,21.6254689009796,0.));
#26146=CARTESIAN_POINT('Ctrl Pts',(-34.6467025072367,21.6254689009796,18.));
#26147=CARTESIAN_POINT('Ctrl Pts',(-34.5894355639081,21.5442132160757,0.));
#26148=CARTESIAN_POINT('Ctrl Pts',(-34.5894355639081,21.5442132160757,18.));
#26149=CARTESIAN_POINT('Ctrl Pts',(-34.5317385658329,21.4634317666005,0.));
#26150=CARTESIAN_POINT('Ctrl Pts',(-34.5317385658329,21.4634317666005,18.));
#26151=CARTESIAN_POINT('Ctrl Pts',(-34.4736054662052,21.3831361300104,0.));
#26152=CARTESIAN_POINT('Ctrl Pts',(-34.4736054662052,21.3831361300104,18.));
#26153=CARTESIAN_POINT('Ctrl Pts',(-34.4150300340623,21.3033382073239,0.));
#26154=CARTESIAN_POINT('Ctrl Pts',(-34.4150300340623,21.3033382073239,18.));
#26155=CARTESIAN_POINT('Ctrl Pts',(-34.3560069185815,21.2240487218079,0.));
#26156=CARTESIAN_POINT('Ctrl Pts',(-34.3560069185815,21.2240487218079,18.));
#26157=CARTESIAN_POINT('Ctrl Pts',(-34.2965325673384,21.1452759244399,0.));
#26158=CARTESIAN_POINT('Ctrl Pts',(-34.2965325673384,21.1452759244399,18.));
#26159=CARTESIAN_POINT('Ctrl Pts',(-34.2366067284279,21.0670234747355,0.));
#26160=CARTESIAN_POINT('Ctrl Pts',(-34.2366067284279,21.0670234747355,18.));
#26161=CARTESIAN_POINT('Ctrl Pts',(-34.176231731809,20.9892914622612,0.));
#26162=CARTESIAN_POINT('Ctrl Pts',(-34.176231731809,20.9892914622612,18.));
#26163=CARTESIAN_POINT('Ctrl Pts',(-34.1154095510973,20.9120805673809,0.));
#26164=CARTESIAN_POINT('Ctrl Pts',(-34.1154095510973,20.9120805673809,18.));
#26165=CARTESIAN_POINT('Ctrl Pts',(-34.0541392299678,20.8353957068415,0.));
#26166=CARTESIAN_POINT('Ctrl Pts',(-34.0541392299678,20.8353957068415,18.));
#26167=CARTESIAN_POINT('Ctrl Pts',(-33.9924146647395,20.7592491770603,0.));
#26168=CARTESIAN_POINT('Ctrl Pts',(-33.9924146647395,20.7592491770603,18.));
#26169=CARTESIAN_POINT('Ctrl Pts',(-33.9302209962425,20.683665762903,0.));
#26170=CARTESIAN_POINT('Ctrl Pts',(-33.9302209962425,20.683665762903,18.));
#26171=CARTESIAN_POINT('Ctrl Pts',(-33.8675365150454,20.6086800574386,0.));
#26172=CARTESIAN_POINT('Ctrl Pts',(-33.8675365150454,20.6086800574386,18.));
#26173=CARTESIAN_POINT('Ctrl Pts',(-33.8043393734971,20.5343269914034,0.));
#26174=CARTESIAN_POINT('Ctrl Pts',(-33.8043393734971,20.5343269914034,18.));
#26175=CARTESIAN_POINT('Ctrl Pts',(-33.7406135254082,20.4606334536183,0.));
#26176=CARTESIAN_POINT('Ctrl Pts',(-33.7406135254082,20.4606334536183,18.));
#26177=CARTESIAN_POINT('Ctrl Pts',(-33.6763537716992,20.3876111773341,0.));
#26178=CARTESIAN_POINT('Ctrl Pts',(-33.6763537716992,20.3876111773341,18.));
#26179=CARTESIAN_POINT('Ctrl Pts',(-33.6115742164079,20.3152448035298,0.));
#26180=CARTESIAN_POINT('Ctrl Pts',(-33.6115742164079,20.3152448035298,18.));
#26181=CARTESIAN_POINT('Ctrl Pts',(-33.5463023319603,20.243500298383,0.));
#26182=CARTESIAN_POINT('Ctrl Pts',(-33.5463023319603,20.243500298383,18.));
#26183=CARTESIAN_POINT('Ctrl Pts',(-33.480563024813,20.1723475154533,0.));
#26184=CARTESIAN_POINT('Ctrl Pts',(-33.480563024813,20.1723475154533,18.));
#26185=CARTESIAN_POINT('Ctrl Pts',(-33.4143643679979,20.1017803986381,0.));
#26186=CARTESIAN_POINT('Ctrl Pts',(-33.4143643679979,20.1017803986381,18.));
#26187=CARTESIAN_POINT('Ctrl Pts',(-33.3476854048385,20.0318342617213,0.));
#26188=CARTESIAN_POINT('Ctrl Pts',(-33.3476854048385,20.0318342617213,18.));
#26189=CARTESIAN_POINT('Ctrl Pts',(-33.2804560993213,19.9626141625205,0.));
#26190=CARTESIAN_POINT('Ctrl Pts',(-33.2804560993213,19.9626141625205,18.));
#26191=CARTESIAN_POINT('Ctrl Pts',(-33.2125746879471,19.8942704458546,0.));
#26192=CARTESIAN_POINT('Ctrl Pts',(-33.2125746879471,19.8942704458546,18.));
#26193=CARTESIAN_POINT('Ctrl Pts',(-33.1439436707661,19.8269479776239,0.));
#26194=CARTESIAN_POINT('Ctrl Pts',(-33.1439436707661,19.8269479776239,18.));
#26195=CARTESIAN_POINT('Ctrl Pts',(-33.0745026283418,19.7607398248651,0.));
#26196=CARTESIAN_POINT('Ctrl Pts',(-33.0745026283418,19.7607398248651,18.));
#26197=CARTESIAN_POINT('Ctrl Pts',(-33.004256563411,19.6956473461873,0.));
#26198=CARTESIAN_POINT('Ctrl Pts',(-33.004256563411,19.6956473461873,18.));
#26199=CARTESIAN_POINT('Ctrl Pts',(-32.9333211533788,19.6315161742485,0.));
#26200=CARTESIAN_POINT('Ctrl Pts',(-32.9333211533788,19.6315161742485,18.));
#26201=CARTESIAN_POINT('Ctrl Pts',(-32.8618672807884,19.5681157030437,0.));
#26202=CARTESIAN_POINT('Ctrl Pts',(-32.8618672807884,19.5681157030437,18.));
#26203=CARTESIAN_POINT('Ctrl Pts',(-32.7900335943248,19.5052640847974,0.));
#26204=CARTESIAN_POINT('Ctrl Pts',(-32.7900335943248,19.5052640847974,18.));
#26205=CARTESIAN_POINT('Ctrl Pts',(-32.7178463324062,19.4429429601189,0.));
#26206=CARTESIAN_POINT('Ctrl Pts',(-32.7178463324062,19.4429429601189,18.));
#26207=CARTESIAN_POINT('Ctrl Pts',(-32.6451434870609,19.381405831319,0.));
#26208=CARTESIAN_POINT('Ctrl Pts',(-32.6451434870609,19.381405831319,18.));
#26209=CARTESIAN_POINT('Ctrl Pts',(-32.5714771007861,19.3213180490743,0.));
#26210=CARTESIAN_POINT('Ctrl Pts',(-32.5714771007861,19.3213180490743,18.));
#26211=CARTESIAN_POINT('Ctrl Pts',(-32.4962340238036,19.2635813403783,0.));
#26212=CARTESIAN_POINT('Ctrl Pts',(-32.4962340238036,19.2635813403783,18.));
#26213=CARTESIAN_POINT('Ctrl Pts',(-32.4342791270009,19.2200039764927,0.));
#26214=CARTESIAN_POINT('Ctrl Pts',(-32.4342791270009,19.2200039764927,18.));
#26215=CARTESIAN_POINT('Ctrl Pts',(-32.3866012518553,19.1891139208368,0.));
#26216=CARTESIAN_POINT('Ctrl Pts',(-32.3866012518553,19.1891139208368,18.));
#26217=CARTESIAN_POINT('Ctrl Pts',(-32.3542491343753,19.1693587749508,0.));
#26218=CARTESIAN_POINT('Ctrl Pts',(-32.3542491343753,19.1693587749508,18.));
#26219=CARTESIAN_POINT('Ctrl Pts',(-32.3379313568208,19.1596907609891,0.));
#26220=CARTESIAN_POINT('Ctrl Pts',(-32.3379313568208,19.1596907609891,18.));
#26221=CARTESIAN_POINT('',(-36.3957374383337,24.7254989094229,0.));
#26222=CARTESIAN_POINT('Ctrl Pts',(-32.3379313568208,19.1596907609891,0.));
#26223=CARTESIAN_POINT('Ctrl Pts',(-32.3542491343753,19.1693587749508,0.));
#26224=CARTESIAN_POINT('Ctrl Pts',(-32.3866012518553,19.1891139208368,0.));
#26225=CARTESIAN_POINT('Ctrl Pts',(-32.4342791270009,19.2200039764927,0.));
#26226=CARTESIAN_POINT('Ctrl Pts',(-32.4962340238036,19.2635813403783,0.));
#26227=CARTESIAN_POINT('Ctrl Pts',(-32.5714771007861,19.3213180490743,0.));
#26228=CARTESIAN_POINT('Ctrl Pts',(-32.6451434870609,19.381405831319,0.));
#26229=CARTESIAN_POINT('Ctrl Pts',(-32.7178463324062,19.4429429601189,0.));
#26230=CARTESIAN_POINT('Ctrl Pts',(-32.7900335943248,19.5052640847974,0.));
#26231=CARTESIAN_POINT('Ctrl Pts',(-32.8618672807884,19.5681157030437,0.));
#26232=CARTESIAN_POINT('Ctrl Pts',(-32.9333211533788,19.6315161742485,0.));
#26233=CARTESIAN_POINT('Ctrl Pts',(-33.004256563411,19.6956473461873,0.));
#26234=CARTESIAN_POINT('Ctrl Pts',(-33.0745026283418,19.7607398248651,0.));
#26235=CARTESIAN_POINT('Ctrl Pts',(-33.1439436707661,19.8269479776239,0.));
#26236=CARTESIAN_POINT('Ctrl Pts',(-33.2125746879471,19.8942704458546,0.));
#26237=CARTESIAN_POINT('Ctrl Pts',(-33.2804560993213,19.9626141625205,0.));
#26238=CARTESIAN_POINT('Ctrl Pts',(-33.3476854048385,20.0318342617213,0.));
#26239=CARTESIAN_POINT('Ctrl Pts',(-33.4143643679979,20.1017803986381,0.));
#26240=CARTESIAN_POINT('Ctrl Pts',(-33.480563024813,20.1723475154533,0.));
#26241=CARTESIAN_POINT('Ctrl Pts',(-33.5463023319603,20.243500298383,0.));
#26242=CARTESIAN_POINT('Ctrl Pts',(-33.6115742164079,20.3152448035298,0.));
#26243=CARTESIAN_POINT('Ctrl Pts',(-33.6763537716992,20.3876111773341,0.));
#26244=CARTESIAN_POINT('Ctrl Pts',(-33.7406135254082,20.4606334536183,0.));
#26245=CARTESIAN_POINT('Ctrl Pts',(-33.8043393734971,20.5343269914034,0.));
#26246=CARTESIAN_POINT('Ctrl Pts',(-33.8675365150454,20.6086800574386,0.));
#26247=CARTESIAN_POINT('Ctrl Pts',(-33.9302209962425,20.683665762903,0.));
#26248=CARTESIAN_POINT('Ctrl Pts',(-33.9924146647395,20.7592491770603,0.));
#26249=CARTESIAN_POINT('Ctrl Pts',(-34.0541392299678,20.8353957068415,0.));
#26250=CARTESIAN_POINT('Ctrl Pts',(-34.1154095510973,20.9120805673809,0.));
#26251=CARTESIAN_POINT('Ctrl Pts',(-34.176231731809,20.9892914622612,0.));
#26252=CARTESIAN_POINT('Ctrl Pts',(-34.2366067284279,21.0670234747355,0.));
#26253=CARTESIAN_POINT('Ctrl Pts',(-34.2965325673384,21.1452759244399,0.));
#26254=CARTESIAN_POINT('Ctrl Pts',(-34.3560069185815,21.2240487218079,0.));
#26255=CARTESIAN_POINT('Ctrl Pts',(-34.4150300340623,21.3033382073239,0.));
#26256=CARTESIAN_POINT('Ctrl Pts',(-34.4736054662052,21.3831361300104,0.));
#26257=CARTESIAN_POINT('Ctrl Pts',(-34.5317385658329,21.4634317666005,0.));
#26258=CARTESIAN_POINT('Ctrl Pts',(-34.5894355639081,21.5442132160757,0.));
#26259=CARTESIAN_POINT('Ctrl Pts',(-34.6467025072367,21.6254689009796,0.));
#26260=CARTESIAN_POINT('Ctrl Pts',(-34.7035440429025,21.7071892844497,0.));
#26261=CARTESIAN_POINT('Ctrl Pts',(-34.7599631530844,21.7893672401137,0.));
#26262=CARTESIAN_POINT('Ctrl Pts',(-34.8159618014436,21.8719971302817,0.));
#26263=CARTESIAN_POINT('Ctrl Pts',(-34.8715413418101,21.9550742217675,0.));
#26264=CARTESIAN_POINT('Ctrl Pts',(-34.9267029879922,22.0385940162683,0.));
#26265=CARTESIAN_POINT('Ctrl Pts',(-34.9814483545602,22.1225514798584,0.));
#26266=CARTESIAN_POINT('Ctrl Pts',(-35.0357795922459,22.2069408519233,0.));
#26267=CARTESIAN_POINT('Ctrl Pts',(-35.0896991159359,22.2917560356803,0.));
#26268=CARTESIAN_POINT('Ctrl Pts',(-35.1432094422642,22.3769908340843,0.));
#26269=CARTESIAN_POINT('Ctrl Pts',(-35.1963130003352,22.4626392230023,0.));
#26270=CARTESIAN_POINT('Ctrl Pts',(-35.2490119207975,22.5486956608909,0.));
#26271=CARTESIAN_POINT('Ctrl Pts',(-35.3013079759252,22.635155167154,0.));
#26272=CARTESIAN_POINT('Ctrl Pts',(-35.3532026952313,22.7220131336912,0.));
#26273=CARTESIAN_POINT('Ctrl Pts',(-35.4046974393492,22.8092652000706,0.));
#26274=CARTESIAN_POINT('Ctrl Pts',(-35.4557934871468,22.8969071125089,0.));
#26275=CARTESIAN_POINT('Ctrl Pts',(-35.5064921357308,22.9849345572033,0.));
#26276=CARTESIAN_POINT('Ctrl Pts',(-35.5567947408311,23.0733431097058,0.));
#26277=CARTESIAN_POINT('Ctrl Pts',(-35.6067026687722,23.1621283508111,0.));
#26278=CARTESIAN_POINT('Ctrl Pts',(-35.6562172725207,23.2512859425032,0.));
#26279=CARTESIAN_POINT('Ctrl Pts',(-35.7053398620512,23.3408117088762,0.));
#26280=CARTESIAN_POINT('Ctrl Pts',(-35.7540716771372,23.4307017328227,0.));
#26281=CARTESIAN_POINT('Ctrl Pts',(-35.8024138716896,23.5209523746427,0.));
#26282=CARTESIAN_POINT('Ctrl Pts',(-35.8503675222885,23.611560139948,0.));
#26283=CARTESIAN_POINT('Ctrl Pts',(-35.8979336336837,23.7025215735353,0.));
#26284=CARTESIAN_POINT('Ctrl Pts',(-35.9451131482488,23.7938331508737,0.));
#26285=CARTESIAN_POINT('Ctrl Pts',(-35.9919069565469,23.8854911428946,0.));
#26286=CARTESIAN_POINT('Ctrl Pts',(-36.0383159101253,23.9774915680089,0.));
#26287=CARTESIAN_POINT('Ctrl Pts',(-36.0843408347974,24.0698304230588,0.));
#26288=CARTESIAN_POINT('Ctrl Pts',(-36.1299825471271,24.1625038657964,0.));
#26289=CARTESIAN_POINT('Ctrl Pts',(-36.1752418704833,24.2555084095332,0.));
#26290=CARTESIAN_POINT('Ctrl Pts',(-36.2201196586696,24.3488411214068,0.));
#26291=CARTESIAN_POINT('Ctrl Pts',(-36.2735162352735,24.4612315181512,0.));
#26292=CARTESIAN_POINT('Ctrl Pts',(-36.3175386315528,24.5552956307817,0.));
#26293=CARTESIAN_POINT('Ctrl Pts',(-36.3524534604648,24.630805301288,0.));
#26294=CARTESIAN_POINT('Ctrl Pts',(-36.3784692650901,24.6875827477484,0.));
#26295=CARTESIAN_POINT('Ctrl Pts',(-36.3957374383337,24.725498909423,0.));
#26296=CARTESIAN_POINT('',(-36.3957374383337,24.7254989094229,15.));
#26297=CARTESIAN_POINT('Ctrl Pts',(-36.3957374383337,24.725498909423,15.));
#26298=CARTESIAN_POINT('Ctrl Pts',(-36.3871033517098,24.7065408286023,15.));
#26299=CARTESIAN_POINT('Ctrl Pts',(-36.369797330215,24.6686569322616,15.));
#26300=CARTESIAN_POINT('Ctrl Pts',(-36.3437247532368,24.6119278836614,15.));
#26301=CARTESIAN_POINT('Ctrl Pts',(-36.3087341522969,24.5364828082556,15.));
#26302=CARTESIAN_POINT('Ctrl Pts',(-36.2646168058395,24.4424997853605,15.));
#26303=CARTESIAN_POINT('Ctrl Pts',(-36.2201196586696,24.3488411214068,15.));
#26304=CARTESIAN_POINT('Ctrl Pts',(-36.1752418704833,24.2555084095332,15.));
#26305=CARTESIAN_POINT('Ctrl Pts',(-36.1299825471271,24.1625038657964,15.));
#26306=CARTESIAN_POINT('Ctrl Pts',(-36.0843408347974,24.0698304230588,15.));
#26307=CARTESIAN_POINT('Ctrl Pts',(-36.0383159101253,23.9774915680089,15.));
#26308=CARTESIAN_POINT('Ctrl Pts',(-35.9919069565469,23.8854911428946,15.));
#26309=CARTESIAN_POINT('Ctrl Pts',(-35.9451131482488,23.7938331508737,15.));
#26310=CARTESIAN_POINT('Ctrl Pts',(-35.8979336336837,23.7025215735353,15.));
#26311=CARTESIAN_POINT('Ctrl Pts',(-35.8503675222885,23.611560139948,15.));
#26312=CARTESIAN_POINT('Ctrl Pts',(-35.8024138716896,23.5209523746427,15.));
#26313=CARTESIAN_POINT('Ctrl Pts',(-35.7540716771372,23.4307017328227,15.));
#26314=CARTESIAN_POINT('Ctrl Pts',(-35.7053398620512,23.3408117088762,15.));
#26315=CARTESIAN_POINT('Ctrl Pts',(-35.6562172725207,23.2512859425032,15.));
#26316=CARTESIAN_POINT('Ctrl Pts',(-35.6067026687722,23.1621283508111,15.));
#26317=CARTESIAN_POINT('Ctrl Pts',(-35.5567947408311,23.0733431097058,15.));
#26318=CARTESIAN_POINT('Ctrl Pts',(-35.5064921357308,22.9849345572033,15.));
#26319=CARTESIAN_POINT('Ctrl Pts',(-35.4557934871468,22.8969071125089,15.));
#26320=CARTESIAN_POINT('Ctrl Pts',(-35.4046974393492,22.8092652000706,15.));
#26321=CARTESIAN_POINT('Ctrl Pts',(-35.3532026952313,22.7220131336912,15.));
#26322=CARTESIAN_POINT('Ctrl Pts',(-35.3013079759252,22.635155167154,15.));
#26323=CARTESIAN_POINT('Ctrl Pts',(-35.2490119207975,22.5486956608909,15.));
#26324=CARTESIAN_POINT('Ctrl Pts',(-35.1963130003352,22.4626392230023,15.));
#26325=CARTESIAN_POINT('Ctrl Pts',(-35.1432094422642,22.3769908340843,15.));
#26326=CARTESIAN_POINT('Ctrl Pts',(-35.0896991159359,22.2917560356803,15.));
#26327=CARTESIAN_POINT('Ctrl Pts',(-35.0357795922459,22.2069408519233,15.));
#26328=CARTESIAN_POINT('Ctrl Pts',(-34.9814483545602,22.1225514798584,15.));
#26329=CARTESIAN_POINT('Ctrl Pts',(-34.9267029879922,22.0385940162683,15.));
#26330=CARTESIAN_POINT('Ctrl Pts',(-34.8715413418101,21.9550742217675,15.));
#26331=CARTESIAN_POINT('Ctrl Pts',(-34.8159618014436,21.8719971302817,15.));
#26332=CARTESIAN_POINT('Ctrl Pts',(-34.7599631530844,21.7893672401137,15.));
#26333=CARTESIAN_POINT('Ctrl Pts',(-34.7035440429025,21.7071892844497,15.));
#26334=CARTESIAN_POINT('Ctrl Pts',(-34.6467025072367,21.6254689009796,15.));
#26335=CARTESIAN_POINT('Ctrl Pts',(-34.5894355639081,21.5442132160757,15.));
#26336=CARTESIAN_POINT('Ctrl Pts',(-34.5317385658329,21.4634317666005,15.));
#26337=CARTESIAN_POINT('Ctrl Pts',(-34.4736054662052,21.3831361300104,15.));
#26338=CARTESIAN_POINT('Ctrl Pts',(-34.4150300340623,21.3033382073239,15.));
#26339=CARTESIAN_POINT('Ctrl Pts',(-34.3560069185815,21.2240487218079,15.));
#26340=CARTESIAN_POINT('Ctrl Pts',(-34.2965325673384,21.1452759244399,15.));
#26341=CARTESIAN_POINT('Ctrl Pts',(-34.2366067284279,21.0670234747355,15.));
#26342=CARTESIAN_POINT('Ctrl Pts',(-34.176231731809,20.9892914622612,15.));
#26343=CARTESIAN_POINT('Ctrl Pts',(-34.1154095510973,20.9120805673809,15.));
#26344=CARTESIAN_POINT('Ctrl Pts',(-34.0541392299678,20.8353957068415,15.));
#26345=CARTESIAN_POINT('Ctrl Pts',(-33.9924146647395,20.7592491770603,15.));
#26346=CARTESIAN_POINT('Ctrl Pts',(-33.9302209962425,20.683665762903,15.));
#26347=CARTESIAN_POINT('Ctrl Pts',(-33.8675365150454,20.6086800574386,15.));
#26348=CARTESIAN_POINT('Ctrl Pts',(-33.8043393734971,20.5343269914034,15.));
#26349=CARTESIAN_POINT('Ctrl Pts',(-33.7406135254082,20.4606334536183,15.));
#26350=CARTESIAN_POINT('Ctrl Pts',(-33.6763537716992,20.3876111773341,15.));
#26351=CARTESIAN_POINT('Ctrl Pts',(-33.6115742164079,20.3152448035298,15.));
#26352=CARTESIAN_POINT('Ctrl Pts',(-33.5463023319603,20.243500298383,15.));
#26353=CARTESIAN_POINT('Ctrl Pts',(-33.480563024813,20.1723475154533,15.));
#26354=CARTESIAN_POINT('Ctrl Pts',(-33.4143643679979,20.1017803986381,15.));
#26355=CARTESIAN_POINT('Ctrl Pts',(-33.3476854048385,20.0318342617213,15.));
#26356=CARTESIAN_POINT('Ctrl Pts',(-33.2804560993213,19.9626141625205,15.));
#26357=CARTESIAN_POINT('Ctrl Pts',(-33.2125746879471,19.8942704458546,15.));
#26358=CARTESIAN_POINT('Ctrl Pts',(-33.1439436707661,19.8269479776239,15.));
#26359=CARTESIAN_POINT('Ctrl Pts',(-33.0745026283418,19.7607398248651,15.));
#26360=CARTESIAN_POINT('Ctrl Pts',(-33.004256563411,19.6956473461873,15.));
#26361=CARTESIAN_POINT('Ctrl Pts',(-32.9333211533788,19.6315161742485,15.));
#26362=CARTESIAN_POINT('Ctrl Pts',(-32.8618672807884,19.5681157030437,15.));
#26363=CARTESIAN_POINT('Ctrl Pts',(-32.7900335943248,19.5052640847974,15.));
#26364=CARTESIAN_POINT('Ctrl Pts',(-32.7178463324062,19.4429429601189,15.));
#26365=CARTESIAN_POINT('Ctrl Pts',(-32.6451434870609,19.381405831319,15.));
#26366=CARTESIAN_POINT('Ctrl Pts',(-32.5714771007861,19.3213180490743,15.));
#26367=CARTESIAN_POINT('Ctrl Pts',(-32.4962340238036,19.2635813403783,15.));
#26368=CARTESIAN_POINT('Ctrl Pts',(-32.4342791270009,19.2200039764927,15.));
#26369=CARTESIAN_POINT('Ctrl Pts',(-32.3866012518553,19.1891139208368,15.));
#26370=CARTESIAN_POINT('Ctrl Pts',(-32.3542491343753,19.1693587749508,15.));
#26371=CARTESIAN_POINT('Ctrl Pts',(-32.3379313568208,19.1596907609891,15.));
#26372=CARTESIAN_POINT('',(-36.3957374383337,24.7254989094229,0.));
#26373=CARTESIAN_POINT('Origin',(-9.16871631793044E-12,6.66146233219319E-12,
0.));
#26374=CARTESIAN_POINT('',(-34.762248247709,26.9738038986838,0.));
#26375=CARTESIAN_POINT('Origin',(-9.16871631793044E-12,6.66146233219319E-12,
0.));
#26376=CARTESIAN_POINT('',(-34.762248247709,26.9738038986838,15.));
#26377=CARTESIAN_POINT('Origin',(-9.16871631793044E-12,6.66146233219319E-12,
15.));
#26378=CARTESIAN_POINT('',(-34.762248247709,26.9738038986838,0.));
#26379=CARTESIAN_POINT('Ctrl Pts',(-28.2149191006268,24.8345302882955,0.));
#26380=CARTESIAN_POINT('Ctrl Pts',(-28.2149191006268,24.8345302882955,18.));
#26381=CARTESIAN_POINT('Ctrl Pts',(-28.2291563988795,24.8470618363541,0.));
#26382=CARTESIAN_POINT('Ctrl Pts',(-28.2291563988795,24.8470618363541,18.));
#26383=CARTESIAN_POINT('Ctrl Pts',(-28.2579420132101,24.8717258526943,0.));
#26384=CARTESIAN_POINT('Ctrl Pts',(-28.2579420132101,24.8717258526943,18.));
#26385=CARTESIAN_POINT('Ctrl Pts',(-28.302053475606,24.9075246543798,0.));
#26386=CARTESIAN_POINT('Ctrl Pts',(-28.302053475606,24.9075246543798,18.));
#26387=CARTESIAN_POINT('Ctrl Pts',(-28.3626431274892,24.9529811166897,0.));
#26388=CARTESIAN_POINT('Ctrl Pts',(-28.3626431274892,24.9529811166897,18.));
#26389=CARTESIAN_POINT('Ctrl Pts',(-28.4408053900206,25.0066999111736,0.));
#26390=CARTESIAN_POINT('Ctrl Pts',(-28.4408053900206,25.0066999111736,18.));
#26391=CARTESIAN_POINT('Ctrl Pts',(-28.5207164321473,25.0581926620043,0.));
#26392=CARTESIAN_POINT('Ctrl Pts',(-28.5207164321473,25.0581926620043,18.));
#26393=CARTESIAN_POINT('Ctrl Pts',(-28.6017081342376,25.108321158239,0.));
#26394=CARTESIAN_POINT('Ctrl Pts',(-28.6017081342376,25.108321158239,18.));
#26395=CARTESIAN_POINT('Ctrl Pts',(-28.6832861366762,25.1577170374459,0.));
#26396=CARTESIAN_POINT('Ctrl Pts',(-28.6832861366762,25.1577170374459,18.));
#26397=CARTESIAN_POINT('Ctrl Pts',(-28.7652594076549,25.2066127148845,0.));
#26398=CARTESIAN_POINT('Ctrl Pts',(-28.7652594076549,25.2066127148845,18.));
#26399=CARTESIAN_POINT('Ctrl Pts',(-28.8476372998748,25.2549775629725,0.));
#26400=CARTESIAN_POINT('Ctrl Pts',(-28.8476372998748,25.2549775629725,18.));
#26401=CARTESIAN_POINT('Ctrl Pts',(-28.9305499160476,25.3026235249214,0.));
#26402=CARTESIAN_POINT('Ctrl Pts',(-28.9305499160476,25.3026235249214,18.));
#26403=CARTESIAN_POINT('Ctrl Pts',(-29.0141637699076,25.3493168206005,0.));
#26404=CARTESIAN_POINT('Ctrl Pts',(-29.0141637699076,25.3493168206005,18.));
#26405=CARTESIAN_POINT('Ctrl Pts',(-29.098589927237,25.3948997321279,0.));
#26406=CARTESIAN_POINT('Ctrl Pts',(-29.098589927237,25.3948997321279,18.));
#26407=CARTESIAN_POINT('Ctrl Pts',(-29.183825549991,25.4393679214513,0.));
#26408=CARTESIAN_POINT('Ctrl Pts',(-29.183825549991,25.4393679214513,18.));
#26409=CARTESIAN_POINT('Ctrl Pts',(-29.2698007967907,25.4828076101654,0.));
#26410=CARTESIAN_POINT('Ctrl Pts',(-29.2698007967907,25.4828076101654,18.));
#26411=CARTESIAN_POINT('Ctrl Pts',(-29.356408021119,25.5253562922582,0.));
#26412=CARTESIAN_POINT('Ctrl Pts',(-29.356408021119,25.5253562922582,18.));
#26413=CARTESIAN_POINT('Ctrl Pts',(-29.443535683207,25.5671572096726,0.));
#26414=CARTESIAN_POINT('Ctrl Pts',(-29.443535683207,25.5671572096726,18.));
#26415=CARTESIAN_POINT('Ctrl Pts',(-29.5311055094509,25.6083094352667,0.));
#26416=CARTESIAN_POINT('Ctrl Pts',(-29.5311055094509,25.6083094352667,18.));
#26417=CARTESIAN_POINT('Ctrl Pts',(-29.6190903904157,25.6488438125835,0.));
#26418=CARTESIAN_POINT('Ctrl Pts',(-29.6190903904157,25.6488438125835,18.));
#26419=CARTESIAN_POINT('Ctrl Pts',(-29.7074935910931,25.6887507922748,0.));
#26420=CARTESIAN_POINT('Ctrl Pts',(-29.7074935910931,25.6887507922748,18.));
#26421=CARTESIAN_POINT('Ctrl Pts',(-29.7963360859334,25.7279973711305,0.));
#26422=CARTESIAN_POINT('Ctrl Pts',(-29.7963360859334,25.7279973711305,18.));
#26423=CARTESIAN_POINT('Ctrl Pts',(-29.8856417535786,25.7665469042913,0.));
#26424=CARTESIAN_POINT('Ctrl Pts',(-29.8856417535786,25.7665469042913,18.));
#26425=CARTESIAN_POINT('Ctrl Pts',(-29.9754208429384,25.8043812318215,0.));
#26426=CARTESIAN_POINT('Ctrl Pts',(-29.9754208429384,25.8043812318215,18.));
#26427=CARTESIAN_POINT('Ctrl Pts',(-30.0656638016321,25.8415089241134,0.));
#26428=CARTESIAN_POINT('Ctrl Pts',(-30.0656638016321,25.8415089241134,18.));
#26429=CARTESIAN_POINT('Ctrl Pts',(-30.1563500154165,25.8779535511028,0.));
#26430=CARTESIAN_POINT('Ctrl Pts',(-30.1563500154165,25.8779535511028,18.));
#26431=CARTESIAN_POINT('Ctrl Pts',(-30.2474530144827,25.9137466853317,0.));
#26432=CARTESIAN_POINT('Ctrl Pts',(-30.2474530144827,25.9137466853317,18.));
#26433=CARTESIAN_POINT('Ctrl Pts',(-30.3389466074503,25.9489196635424,0.));
#26434=CARTESIAN_POINT('Ctrl Pts',(-30.3389466074503,25.9489196635424,18.));
#26435=CARTESIAN_POINT('Ctrl Pts',(-30.4308118142473,25.9834942765902,0.));
#26436=CARTESIAN_POINT('Ctrl Pts',(-30.4308118142473,25.9834942765902,18.));
#26437=CARTESIAN_POINT('Ctrl Pts',(-30.5230388264271,26.0174801292225,0.));
#26438=CARTESIAN_POINT('Ctrl Pts',(-30.5230388264271,26.0174801292225,18.));
#26439=CARTESIAN_POINT('Ctrl Pts',(-30.6156232634061,26.0508796503166,0.));
#26440=CARTESIAN_POINT('Ctrl Pts',(-30.6156232634061,26.0508796503166,18.));
#26441=CARTESIAN_POINT('Ctrl Pts',(-30.7085638682391,26.0836911730968,0.));
#26442=CARTESIAN_POINT('Ctrl Pts',(-30.7085638682391,26.0836911730968,18.));
#26443=CARTESIAN_POINT('Ctrl Pts',(-30.8018598357461,26.1159125093178,0.));
#26444=CARTESIAN_POINT('Ctrl Pts',(-30.8018598357461,26.1159125093178,18.));
#26445=CARTESIAN_POINT('Ctrl Pts',(-30.8955077633644,26.1475450294082,0.));
#26446=CARTESIAN_POINT('Ctrl Pts',(-30.8955077633644,26.1475450294082,18.));
#26447=CARTESIAN_POINT('Ctrl Pts',(-30.9895009017073,26.1785946616165,0.));
#26448=CARTESIAN_POINT('Ctrl Pts',(-30.9895009017073,26.1785946616165,18.));
#26449=CARTESIAN_POINT('Ctrl Pts',(-31.0838307058369,26.2090698085494,0.));
#26450=CARTESIAN_POINT('Ctrl Pts',(-31.0838307058369,26.2090698085494,18.));
#26451=CARTESIAN_POINT('Ctrl Pts',(-31.1784877826858,26.2389800738215,0.));
#26452=CARTESIAN_POINT('Ctrl Pts',(-31.1784877826858,26.2389800738215,18.));
#26453=CARTESIAN_POINT('Ctrl Pts',(-31.2734629900041,26.2683347859175,0.));
#26454=CARTESIAN_POINT('Ctrl Pts',(-31.2734629900041,26.2683347859175,18.));
#26455=CARTESIAN_POINT('Ctrl Pts',(-31.3687486937246,26.2971413115295,0.));
#26456=CARTESIAN_POINT('Ctrl Pts',(-31.3687486937246,26.2971413115295,18.));
#26457=CARTESIAN_POINT('Ctrl Pts',(-31.4643390378084,26.3254046890485,0.));
#26458=CARTESIAN_POINT('Ctrl Pts',(-31.4643390378084,26.3254046890485,18.));
#26459=CARTESIAN_POINT('Ctrl Pts',(-31.5602292672984,26.353128528169,0.));
#26460=CARTESIAN_POINT('Ctrl Pts',(-31.5602292672984,26.353128528169,18.));
#26461=CARTESIAN_POINT('Ctrl Pts',(-31.6564152990236,26.3803155790949,0.));
#26462=CARTESIAN_POINT('Ctrl Pts',(-31.6564152990236,26.3803155790949,18.));
#26463=CARTESIAN_POINT('Ctrl Pts',(-31.7528932299312,26.4069683862785,0.));
#26464=CARTESIAN_POINT('Ctrl Pts',(-31.7528932299312,26.4069683862785,18.));
#26465=CARTESIAN_POINT('Ctrl Pts',(-31.849658771403,26.433090040836,0.));
#26466=CARTESIAN_POINT('Ctrl Pts',(-31.849658771403,26.433090040836,18.));
#26467=CARTESIAN_POINT('Ctrl Pts',(-31.9467071093816,26.4586843683627,0.));
#26468=CARTESIAN_POINT('Ctrl Pts',(-31.9467071093816,26.4586843683627,18.));
#26469=CARTESIAN_POINT('Ctrl Pts',(-32.0440331917233,26.4837555495616,0.));
#26470=CARTESIAN_POINT('Ctrl Pts',(-32.0440331917233,26.4837555495616,18.));
#26471=CARTESIAN_POINT('Ctrl Pts',(-32.1416319023705,26.5083078928862,0.));
#26472=CARTESIAN_POINT('Ctrl Pts',(-32.1416319023705,26.5083078928862,18.));
#26473=CARTESIAN_POINT('Ctrl Pts',(-32.2394982626669,26.5323455701117,0.));
#26474=CARTESIAN_POINT('Ctrl Pts',(-32.2394982626669,26.5323455701117,18.));
#26475=CARTESIAN_POINT('Ctrl Pts',(-32.3376276606981,26.5558723200361,0.));
#26476=CARTESIAN_POINT('Ctrl Pts',(-32.3376276606981,26.5558723200361,18.));
#26477=CARTESIAN_POINT('Ctrl Pts',(-32.4360159072985,26.5788913672813,0.));
#26478=CARTESIAN_POINT('Ctrl Pts',(-32.4360159072985,26.5788913672813,18.));
#26479=CARTESIAN_POINT('Ctrl Pts',(-32.5346590925498,26.6014055904817,0.));
#26480=CARTESIAN_POINT('Ctrl Pts',(-32.5346590925498,26.6014055904817,18.));
#26481=CARTESIAN_POINT('Ctrl Pts',(-32.6335534898935,26.6234176311245,0.));
#26482=CARTESIAN_POINT('Ctrl Pts',(-32.6335534898935,26.6234176311245,18.));
#26483=CARTESIAN_POINT('Ctrl Pts',(-32.7326954489334,26.6449300199764,0.));
#26484=CARTESIAN_POINT('Ctrl Pts',(-32.7326954489334,26.6449300199764,18.));
#26485=CARTESIAN_POINT('Ctrl Pts',(-32.8320812678271,26.6659453236976,0.));
#26486=CARTESIAN_POINT('Ctrl Pts',(-32.8320812678271,26.6659453236976,18.));
#26487=CARTESIAN_POINT('Ctrl Pts',(-32.9317071576181,26.6864661988935,0.));
#26488=CARTESIAN_POINT('Ctrl Pts',(-32.9317071576181,26.6864661988935,18.));
#26489=CARTESIAN_POINT('Ctrl Pts',(-33.03156933761,26.7064953106254,0.));
#26490=CARTESIAN_POINT('Ctrl Pts',(-33.03156933761,26.7064953106254,18.));
#26491=CARTESIAN_POINT('Ctrl Pts',(-33.131664100194,26.7260352861619,0.));
#26492=CARTESIAN_POINT('Ctrl Pts',(-33.131664100194,26.7260352861619,18.));
#26493=CARTESIAN_POINT('Ctrl Pts',(-33.2319878786519,26.7450886617884,0.));
#26494=CARTESIAN_POINT('Ctrl Pts',(-33.2319878786519,26.7450886617884,18.));
#26495=CARTESIAN_POINT('Ctrl Pts',(-33.3325373307046,26.7636578270526,0.));
#26496=CARTESIAN_POINT('Ctrl Pts',(-33.3325373307046,26.7636578270526,18.));
#26497=CARTESIAN_POINT('Ctrl Pts',(-33.4333093513694,26.7817450041181,0.));
#26498=CARTESIAN_POINT('Ctrl Pts',(-33.4333093513694,26.7817450041181,18.));
#26499=CARTESIAN_POINT('Ctrl Pts',(-33.5343009499673,26.7993522966985,0.));
#26500=CARTESIAN_POINT('Ctrl Pts',(-33.5343009499673,26.7993522966985,18.));
#26501=CARTESIAN_POINT('Ctrl Pts',(-33.6355091508895,26.8164817280846,0.));
#26502=CARTESIAN_POINT('Ctrl Pts',(-33.6355091508895,26.8164817280846,18.));
#26503=CARTESIAN_POINT('Ctrl Pts',(-33.7369308933173,26.8331352836667,0.));
#26504=CARTESIAN_POINT('Ctrl Pts',(-33.7369308933173,26.8331352836667,18.));
#26505=CARTESIAN_POINT('Ctrl Pts',(-33.838562905895,26.8493149627661,0.));
#26506=CARTESIAN_POINT('Ctrl Pts',(-33.838562905895,26.8493149627661,18.));
#26507=CARTESIAN_POINT('Ctrl Pts',(-33.9404016650487,26.8650228056313,0.));
#26508=CARTESIAN_POINT('Ctrl Pts',(-33.9404016650487,26.8650228056313,18.));
#26509=CARTESIAN_POINT('Ctrl Pts',(-34.0424436187397,26.880260834701,0.));
#26510=CARTESIAN_POINT('Ctrl Pts',(-34.0424436187397,26.880260834701,18.));
#26511=CARTESIAN_POINT('Ctrl Pts',(-34.1446853651051,26.895031013894,0.));
#26512=CARTESIAN_POINT('Ctrl Pts',(-34.1446853651051,26.895031013894,18.));
#26513=CARTESIAN_POINT('Ctrl Pts',(-34.2471238425419,26.9093352037262,0.));
#26514=CARTESIAN_POINT('Ctrl Pts',(-34.2471238425419,26.9093352037262,18.));
#26515=CARTESIAN_POINT('Ctrl Pts',(-34.3497565255724,26.9231751225177,0.));
#26516=CARTESIAN_POINT('Ctrl Pts',(-34.3497565255724,26.9231751225177,18.));
#26517=CARTESIAN_POINT('Ctrl Pts',(-34.4525815829097,26.9365523054581,0.));
#26518=CARTESIAN_POINT('Ctrl Pts',(-34.4525815829097,26.9365523054581,18.));
#26519=CARTESIAN_POINT('Ctrl Pts',(-34.5555977590573,26.9494680440307,0.));
#26520=CARTESIAN_POINT('Ctrl Pts',(-34.5555977590573,26.9494680440307,18.));
#26521=CARTESIAN_POINT('Ctrl Pts',(-34.6381629799782,26.9594322726214,0.));
#26522=CARTESIAN_POINT('Ctrl Pts',(-34.6381629799782,26.9594322726214,18.));
#26523=CARTESIAN_POINT('Ctrl Pts',(-34.700172380686,26.9666985267609,0.));
#26524=CARTESIAN_POINT('Ctrl Pts',(-34.700172380686,26.9666985267609,18.));
#26525=CARTESIAN_POINT('Ctrl Pts',(-34.7415499619104,26.9714507634923,0.));
#26526=CARTESIAN_POINT('Ctrl Pts',(-34.7415499619104,26.9714507634923,18.));
#26527=CARTESIAN_POINT('Ctrl Pts',(-34.7622482477091,26.9738038986838,0.));
#26528=CARTESIAN_POINT('Ctrl Pts',(-34.7622482477091,26.9738038986838,18.));
#26529=CARTESIAN_POINT('Ctrl Pts',(-28.2149191006268,24.8345302882955,0.));
#26530=CARTESIAN_POINT('Ctrl Pts',(-28.2291563988795,24.8470618363541,0.));
#26531=CARTESIAN_POINT('Ctrl Pts',(-28.2579420132101,24.8717258526943,0.));
#26532=CARTESIAN_POINT('Ctrl Pts',(-28.302053475606,24.9075246543798,0.));
#26533=CARTESIAN_POINT('Ctrl Pts',(-28.3626431274892,24.9529811166897,0.));
#26534=CARTESIAN_POINT('Ctrl Pts',(-28.4408053900206,25.0066999111736,0.));
#26535=CARTESIAN_POINT('Ctrl Pts',(-28.5207164321473,25.0581926620043,0.));
#26536=CARTESIAN_POINT('Ctrl Pts',(-28.6017081342376,25.108321158239,0.));
#26537=CARTESIAN_POINT('Ctrl Pts',(-28.6832861366762,25.1577170374459,0.));
#26538=CARTESIAN_POINT('Ctrl Pts',(-28.7652594076549,25.2066127148845,0.));
#26539=CARTESIAN_POINT('Ctrl Pts',(-28.8476372998748,25.2549775629725,0.));
#26540=CARTESIAN_POINT('Ctrl Pts',(-28.9305499160476,25.3026235249214,0.));
#26541=CARTESIAN_POINT('Ctrl Pts',(-29.0141637699076,25.3493168206005,0.));
#26542=CARTESIAN_POINT('Ctrl Pts',(-29.098589927237,25.3948997321279,0.));
#26543=CARTESIAN_POINT('Ctrl Pts',(-29.183825549991,25.4393679214513,0.));
#26544=CARTESIAN_POINT('Ctrl Pts',(-29.2698007967907,25.4828076101654,0.));
#26545=CARTESIAN_POINT('Ctrl Pts',(-29.356408021119,25.5253562922582,0.));
#26546=CARTESIAN_POINT('Ctrl Pts',(-29.443535683207,25.5671572096726,0.));
#26547=CARTESIAN_POINT('Ctrl Pts',(-29.5311055094509,25.6083094352667,0.));
#26548=CARTESIAN_POINT('Ctrl Pts',(-29.6190903904157,25.6488438125835,0.));
#26549=CARTESIAN_POINT('Ctrl Pts',(-29.7074935910931,25.6887507922748,0.));
#26550=CARTESIAN_POINT('Ctrl Pts',(-29.7963360859334,25.7279973711305,0.));
#26551=CARTESIAN_POINT('Ctrl Pts',(-29.8856417535786,25.7665469042913,0.));
#26552=CARTESIAN_POINT('Ctrl Pts',(-29.9754208429384,25.8043812318215,0.));
#26553=CARTESIAN_POINT('Ctrl Pts',(-30.0656638016321,25.8415089241134,0.));
#26554=CARTESIAN_POINT('Ctrl Pts',(-30.1563500154165,25.8779535511028,0.));
#26555=CARTESIAN_POINT('Ctrl Pts',(-30.2474530144827,25.9137466853317,0.));
#26556=CARTESIAN_POINT('Ctrl Pts',(-30.3389466074503,25.9489196635424,0.));
#26557=CARTESIAN_POINT('Ctrl Pts',(-30.4308118142473,25.9834942765902,0.));
#26558=CARTESIAN_POINT('Ctrl Pts',(-30.5230388264271,26.0174801292225,0.));
#26559=CARTESIAN_POINT('Ctrl Pts',(-30.6156232634061,26.0508796503166,0.));
#26560=CARTESIAN_POINT('Ctrl Pts',(-30.7085638682391,26.0836911730968,0.));
#26561=CARTESIAN_POINT('Ctrl Pts',(-30.8018598357461,26.1159125093178,0.));
#26562=CARTESIAN_POINT('Ctrl Pts',(-30.8955077633644,26.1475450294082,0.));
#26563=CARTESIAN_POINT('Ctrl Pts',(-30.9895009017073,26.1785946616165,0.));
#26564=CARTESIAN_POINT('Ctrl Pts',(-31.0838307058369,26.2090698085494,0.));
#26565=CARTESIAN_POINT('Ctrl Pts',(-31.1784877826858,26.2389800738215,0.));
#26566=CARTESIAN_POINT('Ctrl Pts',(-31.2734629900041,26.2683347859175,0.));
#26567=CARTESIAN_POINT('Ctrl Pts',(-31.3687486937246,26.2971413115295,0.));
#26568=CARTESIAN_POINT('Ctrl Pts',(-31.4643390378084,26.3254046890485,0.));
#26569=CARTESIAN_POINT('Ctrl Pts',(-31.5602292672984,26.353128528169,0.));
#26570=CARTESIAN_POINT('Ctrl Pts',(-31.6564152990236,26.3803155790949,0.));
#26571=CARTESIAN_POINT('Ctrl Pts',(-31.7528932299312,26.4069683862785,0.));
#26572=CARTESIAN_POINT('Ctrl Pts',(-31.849658771403,26.433090040836,0.));
#26573=CARTESIAN_POINT('Ctrl Pts',(-31.9467071093816,26.4586843683627,0.));
#26574=CARTESIAN_POINT('Ctrl Pts',(-32.0440331917233,26.4837555495616,0.));
#26575=CARTESIAN_POINT('Ctrl Pts',(-32.1416319023705,26.5083078928862,0.));
#26576=CARTESIAN_POINT('Ctrl Pts',(-32.2394982626669,26.5323455701117,0.));
#26577=CARTESIAN_POINT('Ctrl Pts',(-32.3376276606981,26.5558723200361,0.));
#26578=CARTESIAN_POINT('Ctrl Pts',(-32.4360159072985,26.5788913672813,0.));
#26579=CARTESIAN_POINT('Ctrl Pts',(-32.5346590925498,26.6014055904817,0.));
#26580=CARTESIAN_POINT('Ctrl Pts',(-32.6335534898935,26.6234176311245,0.));
#26581=CARTESIAN_POINT('Ctrl Pts',(-32.7326954489334,26.6449300199764,0.));
#26582=CARTESIAN_POINT('Ctrl Pts',(-32.8320812678271,26.6659453236976,0.));
#26583=CARTESIAN_POINT('Ctrl Pts',(-32.9317071576181,26.6864661988935,0.));
#26584=CARTESIAN_POINT('Ctrl Pts',(-33.03156933761,26.7064953106254,0.));
#26585=CARTESIAN_POINT('Ctrl Pts',(-33.131664100194,26.7260352861619,0.));
#26586=CARTESIAN_POINT('Ctrl Pts',(-33.2319878786519,26.7450886617884,0.));
#26587=CARTESIAN_POINT('Ctrl Pts',(-33.3325373307046,26.7636578270526,0.));
#26588=CARTESIAN_POINT('Ctrl Pts',(-33.4333093513694,26.7817450041181,0.));
#26589=CARTESIAN_POINT('Ctrl Pts',(-33.5343009499673,26.7993522966985,0.));
#26590=CARTESIAN_POINT('Ctrl Pts',(-33.6355091508895,26.8164817280846,0.));
#26591=CARTESIAN_POINT('Ctrl Pts',(-33.7369308933173,26.8331352836667,0.));
#26592=CARTESIAN_POINT('Ctrl Pts',(-33.838562905895,26.8493149627661,0.));
#26593=CARTESIAN_POINT('Ctrl Pts',(-33.9404016650487,26.8650228056313,0.));
#26594=CARTESIAN_POINT('Ctrl Pts',(-34.0424436187397,26.880260834701,0.));
#26595=CARTESIAN_POINT('Ctrl Pts',(-34.1446853651051,26.895031013894,0.));
#26596=CARTESIAN_POINT('Ctrl Pts',(-34.2471238425419,26.9093352037262,0.));
#26597=CARTESIAN_POINT('Ctrl Pts',(-34.3497565255724,26.9231751225177,0.));
#26598=CARTESIAN_POINT('Ctrl Pts',(-34.4731465943772,26.9392277420462,0.));
#26599=CARTESIAN_POINT('Ctrl Pts',(-34.5762105502273,26.9520281195268,0.));
#26600=CARTESIAN_POINT('Ctrl Pts',(-34.6588137898952,26.9619003236529,0.));
#26601=CARTESIAN_POINT('Ctrl Pts',(-34.7208516760814,26.9690976283149,0.));
#26602=CARTESIAN_POINT('Ctrl Pts',(-34.7622482477091,26.9738038986838,0.));
#26603=CARTESIAN_POINT('Ctrl Pts',(-28.2149191006268,24.8345302882955,15.));
#26604=CARTESIAN_POINT('Ctrl Pts',(-28.2291563988795,24.8470618363541,15.));
#26605=CARTESIAN_POINT('Ctrl Pts',(-28.2579420132101,24.8717258526943,15.));
#26606=CARTESIAN_POINT('Ctrl Pts',(-28.302053475606,24.9075246543798,15.));
#26607=CARTESIAN_POINT('Ctrl Pts',(-28.3626431274892,24.9529811166897,15.));
#26608=CARTESIAN_POINT('Ctrl Pts',(-28.4408053900206,25.0066999111736,15.));
#26609=CARTESIAN_POINT('Ctrl Pts',(-28.5207164321473,25.0581926620043,15.));
#26610=CARTESIAN_POINT('Ctrl Pts',(-28.6017081342376,25.108321158239,15.));
#26611=CARTESIAN_POINT('Ctrl Pts',(-28.6832861366762,25.1577170374459,15.));
#26612=CARTESIAN_POINT('Ctrl Pts',(-28.7652594076549,25.2066127148845,15.));
#26613=CARTESIAN_POINT('Ctrl Pts',(-28.8476372998748,25.2549775629725,15.));
#26614=CARTESIAN_POINT('Ctrl Pts',(-28.9305499160476,25.3026235249214,15.));
#26615=CARTESIAN_POINT('Ctrl Pts',(-29.0141637699076,25.3493168206005,15.));
#26616=CARTESIAN_POINT('Ctrl Pts',(-29.098589927237,25.3948997321279,15.));
#26617=CARTESIAN_POINT('Ctrl Pts',(-29.183825549991,25.4393679214513,15.));
#26618=CARTESIAN_POINT('Ctrl Pts',(-29.2698007967907,25.4828076101654,15.));
#26619=CARTESIAN_POINT('Ctrl Pts',(-29.356408021119,25.5253562922582,15.));
#26620=CARTESIAN_POINT('Ctrl Pts',(-29.443535683207,25.5671572096726,15.));
#26621=CARTESIAN_POINT('Ctrl Pts',(-29.5311055094509,25.6083094352667,15.));
#26622=CARTESIAN_POINT('Ctrl Pts',(-29.6190903904157,25.6488438125835,15.));
#26623=CARTESIAN_POINT('Ctrl Pts',(-29.7074935910931,25.6887507922748,15.));
#26624=CARTESIAN_POINT('Ctrl Pts',(-29.7963360859334,25.7279973711305,15.));
#26625=CARTESIAN_POINT('Ctrl Pts',(-29.8856417535786,25.7665469042913,15.));
#26626=CARTESIAN_POINT('Ctrl Pts',(-29.9754208429384,25.8043812318215,15.));
#26627=CARTESIAN_POINT('Ctrl Pts',(-30.0656638016321,25.8415089241134,15.));
#26628=CARTESIAN_POINT('Ctrl Pts',(-30.1563500154165,25.8779535511028,15.));
#26629=CARTESIAN_POINT('Ctrl Pts',(-30.2474530144827,25.9137466853317,15.));
#26630=CARTESIAN_POINT('Ctrl Pts',(-30.3389466074503,25.9489196635424,15.));
#26631=CARTESIAN_POINT('Ctrl Pts',(-30.4308118142473,25.9834942765902,15.));
#26632=CARTESIAN_POINT('Ctrl Pts',(-30.5230388264271,26.0174801292225,15.));
#26633=CARTESIAN_POINT('Ctrl Pts',(-30.6156232634061,26.0508796503166,15.));
#26634=CARTESIAN_POINT('Ctrl Pts',(-30.7085638682391,26.0836911730968,15.));
#26635=CARTESIAN_POINT('Ctrl Pts',(-30.8018598357461,26.1159125093178,15.));
#26636=CARTESIAN_POINT('Ctrl Pts',(-30.8955077633644,26.1475450294082,15.));
#26637=CARTESIAN_POINT('Ctrl Pts',(-30.9895009017073,26.1785946616165,15.));
#26638=CARTESIAN_POINT('Ctrl Pts',(-31.0838307058369,26.2090698085494,15.));
#26639=CARTESIAN_POINT('Ctrl Pts',(-31.1784877826858,26.2389800738215,15.));
#26640=CARTESIAN_POINT('Ctrl Pts',(-31.2734629900041,26.2683347859175,15.));
#26641=CARTESIAN_POINT('Ctrl Pts',(-31.3687486937246,26.2971413115295,15.));
#26642=CARTESIAN_POINT('Ctrl Pts',(-31.4643390378084,26.3254046890485,15.));
#26643=CARTESIAN_POINT('Ctrl Pts',(-31.5602292672984,26.353128528169,15.));
#26644=CARTESIAN_POINT('Ctrl Pts',(-31.6564152990236,26.3803155790949,15.));
#26645=CARTESIAN_POINT('Ctrl Pts',(-31.7528932299312,26.4069683862785,15.));
#26646=CARTESIAN_POINT('Ctrl Pts',(-31.849658771403,26.433090040836,15.));
#26647=CARTESIAN_POINT('Ctrl Pts',(-31.9467071093816,26.4586843683627,15.));
#26648=CARTESIAN_POINT('Ctrl Pts',(-32.0440331917233,26.4837555495616,15.));
#26649=CARTESIAN_POINT('Ctrl Pts',(-32.1416319023705,26.5083078928862,15.));
#26650=CARTESIAN_POINT('Ctrl Pts',(-32.2394982626669,26.5323455701117,15.));
#26651=CARTESIAN_POINT('Ctrl Pts',(-32.3376276606981,26.5558723200361,15.));
#26652=CARTESIAN_POINT('Ctrl Pts',(-32.4360159072985,26.5788913672813,15.));
#26653=CARTESIAN_POINT('Ctrl Pts',(-32.5346590925498,26.6014055904817,15.));
#26654=CARTESIAN_POINT('Ctrl Pts',(-32.6335534898935,26.6234176311245,15.));
#26655=CARTESIAN_POINT('Ctrl Pts',(-32.7326954489334,26.6449300199764,15.));
#26656=CARTESIAN_POINT('Ctrl Pts',(-32.8320812678271,26.6659453236976,15.));
#26657=CARTESIAN_POINT('Ctrl Pts',(-32.9317071576181,26.6864661988935,15.));
#26658=CARTESIAN_POINT('Ctrl Pts',(-33.03156933761,26.7064953106254,15.));
#26659=CARTESIAN_POINT('Ctrl Pts',(-33.131664100194,26.7260352861619,15.));
#26660=CARTESIAN_POINT('Ctrl Pts',(-33.2319878786519,26.7450886617884,15.));
#26661=CARTESIAN_POINT('Ctrl Pts',(-33.3325373307046,26.7636578270526,15.));
#26662=CARTESIAN_POINT('Ctrl Pts',(-33.4333093513694,26.7817450041181,15.));
#26663=CARTESIAN_POINT('Ctrl Pts',(-33.5343009499673,26.7993522966985,15.));
#26664=CARTESIAN_POINT('Ctrl Pts',(-33.6355091508895,26.8164817280846,15.));
#26665=CARTESIAN_POINT('Ctrl Pts',(-33.7369308933173,26.8331352836667,15.));
#26666=CARTESIAN_POINT('Ctrl Pts',(-33.838562905895,26.8493149627661,15.));
#26667=CARTESIAN_POINT('Ctrl Pts',(-33.9404016650487,26.8650228056313,15.));
#26668=CARTESIAN_POINT('Ctrl Pts',(-34.0424436187397,26.880260834701,15.));
#26669=CARTESIAN_POINT('Ctrl Pts',(-34.1446853651051,26.895031013894,15.));
#26670=CARTESIAN_POINT('Ctrl Pts',(-34.2471238425419,26.9093352037262,15.));
#26671=CARTESIAN_POINT('Ctrl Pts',(-34.3497565255724,26.9231751225177,15.));
#26672=CARTESIAN_POINT('Ctrl Pts',(-34.4731465943772,26.9392277420462,15.));
#26673=CARTESIAN_POINT('Ctrl Pts',(-34.5762105502273,26.9520281195268,15.));
#26674=CARTESIAN_POINT('Ctrl Pts',(-34.6588137898952,26.9619003236529,15.));
#26675=CARTESIAN_POINT('Ctrl Pts',(-34.7208516760814,26.9690976283149,15.));
#26676=CARTESIAN_POINT('Ctrl Pts',(-34.7622482477091,26.9738038986838,15.));
#26677=CARTESIAN_POINT('Ctrl Pts',(-26.9738038986838,34.7622482477091,0.));
#26678=CARTESIAN_POINT('Ctrl Pts',(-26.9738038986838,34.7622482477091,18.));
#26679=CARTESIAN_POINT('Ctrl Pts',(-26.9714507634923,34.7415499619104,0.));
#26680=CARTESIAN_POINT('Ctrl Pts',(-26.9714507634923,34.7415499619104,18.));
#26681=CARTESIAN_POINT('Ctrl Pts',(-26.9666985267608,34.700172380686,0.));
#26682=CARTESIAN_POINT('Ctrl Pts',(-26.9666985267608,34.700172380686,18.));
#26683=CARTESIAN_POINT('Ctrl Pts',(-26.9594322726214,34.6381629799782,0.));
#26684=CARTESIAN_POINT('Ctrl Pts',(-26.9594322726214,34.6381629799782,18.));
#26685=CARTESIAN_POINT('Ctrl Pts',(-26.9494680440307,34.5555977590573,0.));
#26686=CARTESIAN_POINT('Ctrl Pts',(-26.9494680440307,34.5555977590573,18.));
#26687=CARTESIAN_POINT('Ctrl Pts',(-26.9365523054581,34.4525815829097,0.));
#26688=CARTESIAN_POINT('Ctrl Pts',(-26.9365523054581,34.4525815829097,18.));
#26689=CARTESIAN_POINT('Ctrl Pts',(-26.9231751225177,34.3497565255724,0.));
#26690=CARTESIAN_POINT('Ctrl Pts',(-26.9231751225177,34.3497565255724,18.));
#26691=CARTESIAN_POINT('Ctrl Pts',(-26.9093352037262,34.2471238425419,0.));
#26692=CARTESIAN_POINT('Ctrl Pts',(-26.9093352037262,34.2471238425419,18.));
#26693=CARTESIAN_POINT('Ctrl Pts',(-26.8950310138939,34.1446853651051,0.));
#26694=CARTESIAN_POINT('Ctrl Pts',(-26.8950310138939,34.1446853651051,18.));
#26695=CARTESIAN_POINT('Ctrl Pts',(-26.880260834701,34.0424436187397,0.));
#26696=CARTESIAN_POINT('Ctrl Pts',(-26.880260834701,34.0424436187397,18.));
#26697=CARTESIAN_POINT('Ctrl Pts',(-26.8650228056313,33.9404016650487,0.));
#26698=CARTESIAN_POINT('Ctrl Pts',(-26.8650228056313,33.9404016650487,18.));
#26699=CARTESIAN_POINT('Ctrl Pts',(-26.8493149627661,33.838562905895,0.));
#26700=CARTESIAN_POINT('Ctrl Pts',(-26.8493149627661,33.838562905895,18.));
#26701=CARTESIAN_POINT('Ctrl Pts',(-26.8331352836666,33.7369308933173,0.));
#26702=CARTESIAN_POINT('Ctrl Pts',(-26.8331352836666,33.7369308933173,18.));
#26703=CARTESIAN_POINT('Ctrl Pts',(-26.8164817280846,33.6355091508895,0.));
#26704=CARTESIAN_POINT('Ctrl Pts',(-26.8164817280846,33.6355091508895,18.));
#26705=CARTESIAN_POINT('Ctrl Pts',(-26.7993522966985,33.5343009499673,0.));
#26706=CARTESIAN_POINT('Ctrl Pts',(-26.7993522966985,33.5343009499673,18.));
#26707=CARTESIAN_POINT('Ctrl Pts',(-26.7817450041181,33.4333093513694,0.));
#26708=CARTESIAN_POINT('Ctrl Pts',(-26.7817450041181,33.4333093513694,18.));
#26709=CARTESIAN_POINT('Ctrl Pts',(-26.7636578270526,33.3325373307046,0.));
#26710=CARTESIAN_POINT('Ctrl Pts',(-26.7636578270526,33.3325373307046,18.));
#26711=CARTESIAN_POINT('Ctrl Pts',(-26.7450886617884,33.2319878786519,0.));
#26712=CARTESIAN_POINT('Ctrl Pts',(-26.7450886617884,33.2319878786519,18.));
#26713=CARTESIAN_POINT('Ctrl Pts',(-26.7260352861619,33.131664100194,0.));
#26714=CARTESIAN_POINT('Ctrl Pts',(-26.7260352861619,33.131664100194,18.));
#26715=CARTESIAN_POINT('Ctrl Pts',(-26.7064953106254,33.03156933761,0.));
#26716=CARTESIAN_POINT('Ctrl Pts',(-26.7064953106254,33.03156933761,18.));
#26717=CARTESIAN_POINT('Ctrl Pts',(-26.6864661988935,32.9317071576181,0.));
#26718=CARTESIAN_POINT('Ctrl Pts',(-26.6864661988935,32.9317071576181,18.));
#26719=CARTESIAN_POINT('Ctrl Pts',(-26.6659453236976,32.8320812678271,0.));
#26720=CARTESIAN_POINT('Ctrl Pts',(-26.6659453236976,32.8320812678271,18.));
#26721=CARTESIAN_POINT('Ctrl Pts',(-26.6449300199763,32.7326954489334,0.));
#26722=CARTESIAN_POINT('Ctrl Pts',(-26.6449300199763,32.7326954489334,18.));
#26723=CARTESIAN_POINT('Ctrl Pts',(-26.6234176311245,32.6335534898936,0.));
#26724=CARTESIAN_POINT('Ctrl Pts',(-26.6234176311245,32.6335534898936,18.));
#26725=CARTESIAN_POINT('Ctrl Pts',(-26.6014055904817,32.5346590925498,0.));
#26726=CARTESIAN_POINT('Ctrl Pts',(-26.6014055904817,32.5346590925498,18.));
#26727=CARTESIAN_POINT('Ctrl Pts',(-26.5788913672813,32.4360159072985,0.));
#26728=CARTESIAN_POINT('Ctrl Pts',(-26.5788913672813,32.4360159072985,18.));
#26729=CARTESIAN_POINT('Ctrl Pts',(-26.5558723200361,32.3376276606981,0.));
#26730=CARTESIAN_POINT('Ctrl Pts',(-26.5558723200361,32.3376276606981,18.));
#26731=CARTESIAN_POINT('Ctrl Pts',(-26.5323455701117,32.2394982626669,0.));
#26732=CARTESIAN_POINT('Ctrl Pts',(-26.5323455701117,32.2394982626669,18.));
#26733=CARTESIAN_POINT('Ctrl Pts',(-26.5083078928862,32.1416319023705,0.));
#26734=CARTESIAN_POINT('Ctrl Pts',(-26.5083078928862,32.1416319023705,18.));
#26735=CARTESIAN_POINT('Ctrl Pts',(-26.4837555495616,32.0440331917233,0.));
#26736=CARTESIAN_POINT('Ctrl Pts',(-26.4837555495616,32.0440331917233,18.));
#26737=CARTESIAN_POINT('Ctrl Pts',(-26.4586843683627,31.9467071093816,0.));
#26738=CARTESIAN_POINT('Ctrl Pts',(-26.4586843683627,31.9467071093816,18.));
#26739=CARTESIAN_POINT('Ctrl Pts',(-26.433090040836,31.849658771403,0.));
#26740=CARTESIAN_POINT('Ctrl Pts',(-26.433090040836,31.849658771403,18.));
#26741=CARTESIAN_POINT('Ctrl Pts',(-26.4069683862784,31.7528932299312,0.));
#26742=CARTESIAN_POINT('Ctrl Pts',(-26.4069683862784,31.7528932299312,18.));
#26743=CARTESIAN_POINT('Ctrl Pts',(-26.3803155790949,31.6564152990236,0.));
#26744=CARTESIAN_POINT('Ctrl Pts',(-26.3803155790949,31.6564152990236,18.));
#26745=CARTESIAN_POINT('Ctrl Pts',(-26.353128528169,31.5602292672984,0.));
#26746=CARTESIAN_POINT('Ctrl Pts',(-26.353128528169,31.5602292672984,18.));
#26747=CARTESIAN_POINT('Ctrl Pts',(-26.3254046890485,31.4643390378084,0.));
#26748=CARTESIAN_POINT('Ctrl Pts',(-26.3254046890485,31.4643390378084,18.));
#26749=CARTESIAN_POINT('Ctrl Pts',(-26.2971413115295,31.3687486937246,0.));
#26750=CARTESIAN_POINT('Ctrl Pts',(-26.2971413115295,31.3687486937246,18.));
#26751=CARTESIAN_POINT('Ctrl Pts',(-26.2683347859175,31.2734629900041,0.));
#26752=CARTESIAN_POINT('Ctrl Pts',(-26.2683347859175,31.2734629900041,18.));
#26753=CARTESIAN_POINT('Ctrl Pts',(-26.2389800738215,31.1784877826858,0.));
#26754=CARTESIAN_POINT('Ctrl Pts',(-26.2389800738215,31.1784877826858,18.));
#26755=CARTESIAN_POINT('Ctrl Pts',(-26.2090698085494,31.0838307058369,0.));
#26756=CARTESIAN_POINT('Ctrl Pts',(-26.2090698085494,31.0838307058369,18.));
#26757=CARTESIAN_POINT('Ctrl Pts',(-26.1785946616165,30.9895009017073,0.));
#26758=CARTESIAN_POINT('Ctrl Pts',(-26.1785946616165,30.9895009017073,18.));
#26759=CARTESIAN_POINT('Ctrl Pts',(-26.1475450294082,30.8955077633644,0.));
#26760=CARTESIAN_POINT('Ctrl Pts',(-26.1475450294082,30.8955077633644,18.));
#26761=CARTESIAN_POINT('Ctrl Pts',(-26.1159125093178,30.8018598357461,0.));
#26762=CARTESIAN_POINT('Ctrl Pts',(-26.1159125093178,30.8018598357461,18.));
#26763=CARTESIAN_POINT('Ctrl Pts',(-26.0836911730968,30.7085638682391,0.));
#26764=CARTESIAN_POINT('Ctrl Pts',(-26.0836911730968,30.7085638682391,18.));
#26765=CARTESIAN_POINT('Ctrl Pts',(-26.0508796503166,30.6156232634061,0.));
#26766=CARTESIAN_POINT('Ctrl Pts',(-26.0508796503166,30.6156232634061,18.));
#26767=CARTESIAN_POINT('Ctrl Pts',(-26.0174801292225,30.5230388264271,0.));
#26768=CARTESIAN_POINT('Ctrl Pts',(-26.0174801292225,30.5230388264271,18.));
#26769=CARTESIAN_POINT('Ctrl Pts',(-25.9834942765902,30.4308118142473,0.));
#26770=CARTESIAN_POINT('Ctrl Pts',(-25.9834942765902,30.4308118142473,18.));
#26771=CARTESIAN_POINT('Ctrl Pts',(-25.9489196635424,30.3389466074503,0.));
#26772=CARTESIAN_POINT('Ctrl Pts',(-25.9489196635424,30.3389466074503,18.));
#26773=CARTESIAN_POINT('Ctrl Pts',(-25.9137466853317,30.2474530144827,0.));
#26774=CARTESIAN_POINT('Ctrl Pts',(-25.9137466853317,30.2474530144827,18.));
#26775=CARTESIAN_POINT('Ctrl Pts',(-25.8779535511027,30.1563500154165,0.));
#26776=CARTESIAN_POINT('Ctrl Pts',(-25.8779535511027,30.1563500154165,18.));
#26777=CARTESIAN_POINT('Ctrl Pts',(-25.8415089241134,30.0656638016321,0.));
#26778=CARTESIAN_POINT('Ctrl Pts',(-25.8415089241134,30.0656638016321,18.));
#26779=CARTESIAN_POINT('Ctrl Pts',(-25.8043812318214,29.9754208429384,0.));
#26780=CARTESIAN_POINT('Ctrl Pts',(-25.8043812318214,29.9754208429384,18.));
#26781=CARTESIAN_POINT('Ctrl Pts',(-25.7665469042913,29.8856417535786,0.));
#26782=CARTESIAN_POINT('Ctrl Pts',(-25.7665469042913,29.8856417535786,18.));
#26783=CARTESIAN_POINT('Ctrl Pts',(-25.7279973711305,29.7963360859334,0.));
#26784=CARTESIAN_POINT('Ctrl Pts',(-25.7279973711305,29.7963360859334,18.));
#26785=CARTESIAN_POINT('Ctrl Pts',(-25.6887507922748,29.7074935910931,0.));
#26786=CARTESIAN_POINT('Ctrl Pts',(-25.6887507922748,29.7074935910931,18.));
#26787=CARTESIAN_POINT('Ctrl Pts',(-25.6488438125835,29.6190903904157,0.));
#26788=CARTESIAN_POINT('Ctrl Pts',(-25.6488438125835,29.6190903904157,18.));
#26789=CARTESIAN_POINT('Ctrl Pts',(-25.6083094352667,29.5311055094509,0.));
#26790=CARTESIAN_POINT('Ctrl Pts',(-25.6083094352667,29.5311055094509,18.));
#26791=CARTESIAN_POINT('Ctrl Pts',(-25.5671572096726,29.443535683207,0.));
#26792=CARTESIAN_POINT('Ctrl Pts',(-25.5671572096726,29.443535683207,18.));
#26793=CARTESIAN_POINT('Ctrl Pts',(-25.5253562922582,29.356408021119,0.));
#26794=CARTESIAN_POINT('Ctrl Pts',(-25.5253562922582,29.356408021119,18.));
#26795=CARTESIAN_POINT('Ctrl Pts',(-25.4828076101654,29.2698007967907,0.));
#26796=CARTESIAN_POINT('Ctrl Pts',(-25.4828076101654,29.2698007967907,18.));
#26797=CARTESIAN_POINT('Ctrl Pts',(-25.4393679214513,29.183825549991,0.));
#26798=CARTESIAN_POINT('Ctrl Pts',(-25.4393679214513,29.183825549991,18.));
#26799=CARTESIAN_POINT('Ctrl Pts',(-25.3948997321279,29.098589927237,0.));
#26800=CARTESIAN_POINT('Ctrl Pts',(-25.3948997321279,29.098589927237,18.));
#26801=CARTESIAN_POINT('Ctrl Pts',(-25.3493168206005,29.0141637699076,0.));
#26802=CARTESIAN_POINT('Ctrl Pts',(-25.3493168206005,29.0141637699076,18.));
#26803=CARTESIAN_POINT('Ctrl Pts',(-25.3026235249214,28.9305499160476,0.));
#26804=CARTESIAN_POINT('Ctrl Pts',(-25.3026235249214,28.9305499160476,18.));
#26805=CARTESIAN_POINT('Ctrl Pts',(-25.2549775629725,28.8476372998748,0.));
#26806=CARTESIAN_POINT('Ctrl Pts',(-25.2549775629725,28.8476372998748,18.));
#26807=CARTESIAN_POINT('Ctrl Pts',(-25.2066127148845,28.7652594076549,0.));
#26808=CARTESIAN_POINT('Ctrl Pts',(-25.2066127148845,28.7652594076549,18.));
#26809=CARTESIAN_POINT('Ctrl Pts',(-25.1577170374459,28.6832861366762,0.));
#26810=CARTESIAN_POINT('Ctrl Pts',(-25.1577170374459,28.6832861366762,18.));
#26811=CARTESIAN_POINT('Ctrl Pts',(-25.108321158239,28.6017081342376,0.));
#26812=CARTESIAN_POINT('Ctrl Pts',(-25.108321158239,28.6017081342376,18.));
#26813=CARTESIAN_POINT('Ctrl Pts',(-25.0581926620043,28.5207164321473,0.));
#26814=CARTESIAN_POINT('Ctrl Pts',(-25.0581926620043,28.5207164321473,18.));
#26815=CARTESIAN_POINT('Ctrl Pts',(-25.0066999111736,28.4408053900206,0.));
#26816=CARTESIAN_POINT('Ctrl Pts',(-25.0066999111736,28.4408053900206,18.));
#26817=CARTESIAN_POINT('Ctrl Pts',(-24.9529811166897,28.3626431274892,0.));
#26818=CARTESIAN_POINT('Ctrl Pts',(-24.9529811166897,28.3626431274892,18.));
#26819=CARTESIAN_POINT('Ctrl Pts',(-24.9075246543798,28.3020534756061,0.));
#26820=CARTESIAN_POINT('Ctrl Pts',(-24.9075246543798,28.3020534756061,18.));
#26821=CARTESIAN_POINT('Ctrl Pts',(-24.8717258526943,28.2579420132101,0.));
#26822=CARTESIAN_POINT('Ctrl Pts',(-24.8717258526943,28.2579420132101,18.));
#26823=CARTESIAN_POINT('Ctrl Pts',(-24.8470618363541,28.2291563988796,0.));
#26824=CARTESIAN_POINT('Ctrl Pts',(-24.8470618363541,28.2291563988796,18.));
#26825=CARTESIAN_POINT('Ctrl Pts',(-24.8345302882955,28.2149191006269,0.));
#26826=CARTESIAN_POINT('Ctrl Pts',(-24.8345302882955,28.2149191006269,18.));
#26827=CARTESIAN_POINT('',(-26.9738038986839,34.762248247709,0.));
#26828=CARTESIAN_POINT('Ctrl Pts',(-24.8345302882955,28.2149191006269,0.));
#26829=CARTESIAN_POINT('Ctrl Pts',(-24.8470618363541,28.2291563988796,0.));
#26830=CARTESIAN_POINT('Ctrl Pts',(-24.8717258526943,28.2579420132101,0.));
#26831=CARTESIAN_POINT('Ctrl Pts',(-24.9075246543798,28.3020534756061,0.));
#26832=CARTESIAN_POINT('Ctrl Pts',(-24.9529811166897,28.3626431274892,0.));
#26833=CARTESIAN_POINT('Ctrl Pts',(-25.0066999111736,28.4408053900206,0.));
#26834=CARTESIAN_POINT('Ctrl Pts',(-25.0581926620043,28.5207164321473,0.));
#26835=CARTESIAN_POINT('Ctrl Pts',(-25.108321158239,28.6017081342376,0.));
#26836=CARTESIAN_POINT('Ctrl Pts',(-25.1577170374459,28.6832861366762,0.));
#26837=CARTESIAN_POINT('Ctrl Pts',(-25.2066127148845,28.7652594076549,0.));
#26838=CARTESIAN_POINT('Ctrl Pts',(-25.2549775629725,28.8476372998748,0.));
#26839=CARTESIAN_POINT('Ctrl Pts',(-25.3026235249214,28.9305499160476,0.));
#26840=CARTESIAN_POINT('Ctrl Pts',(-25.3493168206005,29.0141637699076,0.));
#26841=CARTESIAN_POINT('Ctrl Pts',(-25.3948997321279,29.098589927237,0.));
#26842=CARTESIAN_POINT('Ctrl Pts',(-25.4393679214513,29.183825549991,0.));
#26843=CARTESIAN_POINT('Ctrl Pts',(-25.4828076101654,29.2698007967907,0.));
#26844=CARTESIAN_POINT('Ctrl Pts',(-25.5253562922582,29.356408021119,0.));
#26845=CARTESIAN_POINT('Ctrl Pts',(-25.5671572096726,29.443535683207,0.));
#26846=CARTESIAN_POINT('Ctrl Pts',(-25.6083094352667,29.5311055094509,0.));
#26847=CARTESIAN_POINT('Ctrl Pts',(-25.6488438125835,29.6190903904157,0.));
#26848=CARTESIAN_POINT('Ctrl Pts',(-25.6887507922748,29.7074935910931,0.));
#26849=CARTESIAN_POINT('Ctrl Pts',(-25.7279973711305,29.7963360859334,0.));
#26850=CARTESIAN_POINT('Ctrl Pts',(-25.7665469042913,29.8856417535786,0.));
#26851=CARTESIAN_POINT('Ctrl Pts',(-25.8043812318214,29.9754208429384,0.));
#26852=CARTESIAN_POINT('Ctrl Pts',(-25.8415089241134,30.0656638016321,0.));
#26853=CARTESIAN_POINT('Ctrl Pts',(-25.8779535511027,30.1563500154165,0.));
#26854=CARTESIAN_POINT('Ctrl Pts',(-25.9137466853317,30.2474530144827,0.));
#26855=CARTESIAN_POINT('Ctrl Pts',(-25.9489196635424,30.3389466074503,0.));
#26856=CARTESIAN_POINT('Ctrl Pts',(-25.9834942765902,30.4308118142473,0.));
#26857=CARTESIAN_POINT('Ctrl Pts',(-26.0174801292225,30.5230388264271,0.));
#26858=CARTESIAN_POINT('Ctrl Pts',(-26.0508796503166,30.6156232634061,0.));
#26859=CARTESIAN_POINT('Ctrl Pts',(-26.0836911730968,30.7085638682391,0.));
#26860=CARTESIAN_POINT('Ctrl Pts',(-26.1159125093178,30.8018598357461,0.));
#26861=CARTESIAN_POINT('Ctrl Pts',(-26.1475450294082,30.8955077633644,0.));
#26862=CARTESIAN_POINT('Ctrl Pts',(-26.1785946616165,30.9895009017073,0.));
#26863=CARTESIAN_POINT('Ctrl Pts',(-26.2090698085494,31.0838307058369,0.));
#26864=CARTESIAN_POINT('Ctrl Pts',(-26.2389800738215,31.1784877826858,0.));
#26865=CARTESIAN_POINT('Ctrl Pts',(-26.2683347859175,31.2734629900041,0.));
#26866=CARTESIAN_POINT('Ctrl Pts',(-26.2971413115295,31.3687486937246,0.));
#26867=CARTESIAN_POINT('Ctrl Pts',(-26.3254046890485,31.4643390378084,0.));
#26868=CARTESIAN_POINT('Ctrl Pts',(-26.353128528169,31.5602292672984,0.));
#26869=CARTESIAN_POINT('Ctrl Pts',(-26.3803155790949,31.6564152990236,0.));
#26870=CARTESIAN_POINT('Ctrl Pts',(-26.4069683862784,31.7528932299312,0.));
#26871=CARTESIAN_POINT('Ctrl Pts',(-26.433090040836,31.849658771403,0.));
#26872=CARTESIAN_POINT('Ctrl Pts',(-26.4586843683627,31.9467071093816,0.));
#26873=CARTESIAN_POINT('Ctrl Pts',(-26.4837555495616,32.0440331917233,0.));
#26874=CARTESIAN_POINT('Ctrl Pts',(-26.5083078928862,32.1416319023705,0.));
#26875=CARTESIAN_POINT('Ctrl Pts',(-26.5323455701117,32.2394982626669,0.));
#26876=CARTESIAN_POINT('Ctrl Pts',(-26.5558723200361,32.3376276606981,0.));
#26877=CARTESIAN_POINT('Ctrl Pts',(-26.5788913672813,32.4360159072985,0.));
#26878=CARTESIAN_POINT('Ctrl Pts',(-26.6014055904817,32.5346590925498,0.));
#26879=CARTESIAN_POINT('Ctrl Pts',(-26.6234176311245,32.6335534898936,0.));
#26880=CARTESIAN_POINT('Ctrl Pts',(-26.6449300199763,32.7326954489334,0.));
#26881=CARTESIAN_POINT('Ctrl Pts',(-26.6659453236976,32.8320812678271,0.));
#26882=CARTESIAN_POINT('Ctrl Pts',(-26.6864661988935,32.9317071576181,0.));
#26883=CARTESIAN_POINT('Ctrl Pts',(-26.7064953106254,33.03156933761,0.));
#26884=CARTESIAN_POINT('Ctrl Pts',(-26.7260352861619,33.131664100194,0.));
#26885=CARTESIAN_POINT('Ctrl Pts',(-26.7450886617884,33.2319878786519,0.));
#26886=CARTESIAN_POINT('Ctrl Pts',(-26.7636578270526,33.3325373307046,0.));
#26887=CARTESIAN_POINT('Ctrl Pts',(-26.7817450041181,33.4333093513694,0.));
#26888=CARTESIAN_POINT('Ctrl Pts',(-26.7993522966985,33.5343009499673,0.));
#26889=CARTESIAN_POINT('Ctrl Pts',(-26.8164817280846,33.6355091508895,0.));
#26890=CARTESIAN_POINT('Ctrl Pts',(-26.8331352836666,33.7369308933173,0.));
#26891=CARTESIAN_POINT('Ctrl Pts',(-26.8493149627661,33.838562905895,0.));
#26892=CARTESIAN_POINT('Ctrl Pts',(-26.8650228056313,33.9404016650487,0.));
#26893=CARTESIAN_POINT('Ctrl Pts',(-26.880260834701,34.0424436187397,0.));
#26894=CARTESIAN_POINT('Ctrl Pts',(-26.8950310138939,34.1446853651051,0.));
#26895=CARTESIAN_POINT('Ctrl Pts',(-26.9093352037262,34.2471238425419,0.));
#26896=CARTESIAN_POINT('Ctrl Pts',(-26.9231751225177,34.3497565255724,0.));
#26897=CARTESIAN_POINT('Ctrl Pts',(-26.9392277420462,34.4731465943772,0.));
#26898=CARTESIAN_POINT('Ctrl Pts',(-26.9520281195268,34.5762105502273,0.));
#26899=CARTESIAN_POINT('Ctrl Pts',(-26.9619003236529,34.6588137898952,0.));
#26900=CARTESIAN_POINT('Ctrl Pts',(-26.9690976283147,34.7208516760814,0.));
#26901=CARTESIAN_POINT('Ctrl Pts',(-26.9738038986838,34.7622482477091,0.));
#26902=CARTESIAN_POINT('',(-26.9738038986839,34.762248247709,15.));
#26903=CARTESIAN_POINT('Ctrl Pts',(-26.9738038986838,34.7622482477091,15.));
#26904=CARTESIAN_POINT('Ctrl Pts',(-26.9714507634923,34.7415499619104,15.));
#26905=CARTESIAN_POINT('Ctrl Pts',(-26.9666985267608,34.700172380686,15.));
#26906=CARTESIAN_POINT('Ctrl Pts',(-26.9594322726214,34.6381629799782,15.));
#26907=CARTESIAN_POINT('Ctrl Pts',(-26.9494680440307,34.5555977590573,15.));
#26908=CARTESIAN_POINT('Ctrl Pts',(-26.9365523054581,34.4525815829097,15.));
#26909=CARTESIAN_POINT('Ctrl Pts',(-26.9231751225177,34.3497565255724,15.));
#26910=CARTESIAN_POINT('Ctrl Pts',(-26.9093352037262,34.2471238425419,15.));
#26911=CARTESIAN_POINT('Ctrl Pts',(-26.8950310138939,34.1446853651051,15.));
#26912=CARTESIAN_POINT('Ctrl Pts',(-26.880260834701,34.0424436187397,15.));
#26913=CARTESIAN_POINT('Ctrl Pts',(-26.8650228056313,33.9404016650487,15.));
#26914=CARTESIAN_POINT('Ctrl Pts',(-26.8493149627661,33.838562905895,15.));
#26915=CARTESIAN_POINT('Ctrl Pts',(-26.8331352836666,33.7369308933173,15.));
#26916=CARTESIAN_POINT('Ctrl Pts',(-26.8164817280846,33.6355091508895,15.));
#26917=CARTESIAN_POINT('Ctrl Pts',(-26.7993522966985,33.5343009499673,15.));
#26918=CARTESIAN_POINT('Ctrl Pts',(-26.7817450041181,33.4333093513694,15.));
#26919=CARTESIAN_POINT('Ctrl Pts',(-26.7636578270526,33.3325373307046,15.));
#26920=CARTESIAN_POINT('Ctrl Pts',(-26.7450886617884,33.2319878786519,15.));
#26921=CARTESIAN_POINT('Ctrl Pts',(-26.7260352861619,33.131664100194,15.));
#26922=CARTESIAN_POINT('Ctrl Pts',(-26.7064953106254,33.03156933761,15.));
#26923=CARTESIAN_POINT('Ctrl Pts',(-26.6864661988935,32.9317071576181,15.));
#26924=CARTESIAN_POINT('Ctrl Pts',(-26.6659453236976,32.8320812678271,15.));
#26925=CARTESIAN_POINT('Ctrl Pts',(-26.6449300199763,32.7326954489334,15.));
#26926=CARTESIAN_POINT('Ctrl Pts',(-26.6234176311245,32.6335534898936,15.));
#26927=CARTESIAN_POINT('Ctrl Pts',(-26.6014055904817,32.5346590925498,15.));
#26928=CARTESIAN_POINT('Ctrl Pts',(-26.5788913672813,32.4360159072985,15.));
#26929=CARTESIAN_POINT('Ctrl Pts',(-26.5558723200361,32.3376276606981,15.));
#26930=CARTESIAN_POINT('Ctrl Pts',(-26.5323455701117,32.2394982626669,15.));
#26931=CARTESIAN_POINT('Ctrl Pts',(-26.5083078928862,32.1416319023705,15.));
#26932=CARTESIAN_POINT('Ctrl Pts',(-26.4837555495616,32.0440331917233,15.));
#26933=CARTESIAN_POINT('Ctrl Pts',(-26.4586843683627,31.9467071093816,15.));
#26934=CARTESIAN_POINT('Ctrl Pts',(-26.433090040836,31.849658771403,15.));
#26935=CARTESIAN_POINT('Ctrl Pts',(-26.4069683862784,31.7528932299312,15.));
#26936=CARTESIAN_POINT('Ctrl Pts',(-26.3803155790949,31.6564152990236,15.));
#26937=CARTESIAN_POINT('Ctrl Pts',(-26.353128528169,31.5602292672984,15.));
#26938=CARTESIAN_POINT('Ctrl Pts',(-26.3254046890485,31.4643390378084,15.));
#26939=CARTESIAN_POINT('Ctrl Pts',(-26.2971413115295,31.3687486937246,15.));
#26940=CARTESIAN_POINT('Ctrl Pts',(-26.2683347859175,31.2734629900041,15.));
#26941=CARTESIAN_POINT('Ctrl Pts',(-26.2389800738215,31.1784877826858,15.));
#26942=CARTESIAN_POINT('Ctrl Pts',(-26.2090698085494,31.0838307058369,15.));
#26943=CARTESIAN_POINT('Ctrl Pts',(-26.1785946616165,30.9895009017073,15.));
#26944=CARTESIAN_POINT('Ctrl Pts',(-26.1475450294082,30.8955077633644,15.));
#26945=CARTESIAN_POINT('Ctrl Pts',(-26.1159125093178,30.8018598357461,15.));
#26946=CARTESIAN_POINT('Ctrl Pts',(-26.0836911730968,30.7085638682391,15.));
#26947=CARTESIAN_POINT('Ctrl Pts',(-26.0508796503166,30.6156232634061,15.));
#26948=CARTESIAN_POINT('Ctrl Pts',(-26.0174801292225,30.5230388264271,15.));
#26949=CARTESIAN_POINT('Ctrl Pts',(-25.9834942765902,30.4308118142473,15.));
#26950=CARTESIAN_POINT('Ctrl Pts',(-25.9489196635424,30.3389466074503,15.));
#26951=CARTESIAN_POINT('Ctrl Pts',(-25.9137466853317,30.2474530144827,15.));
#26952=CARTESIAN_POINT('Ctrl Pts',(-25.8779535511027,30.1563500154165,15.));
#26953=CARTESIAN_POINT('Ctrl Pts',(-25.8415089241134,30.0656638016321,15.));
#26954=CARTESIAN_POINT('Ctrl Pts',(-25.8043812318214,29.9754208429384,15.));
#26955=CARTESIAN_POINT('Ctrl Pts',(-25.7665469042913,29.8856417535786,15.));
#26956=CARTESIAN_POINT('Ctrl Pts',(-25.7279973711305,29.7963360859334,15.));
#26957=CARTESIAN_POINT('Ctrl Pts',(-25.6887507922748,29.7074935910931,15.));
#26958=CARTESIAN_POINT('Ctrl Pts',(-25.6488438125835,29.6190903904157,15.));
#26959=CARTESIAN_POINT('Ctrl Pts',(-25.6083094352667,29.5311055094509,15.));
#26960=CARTESIAN_POINT('Ctrl Pts',(-25.5671572096726,29.443535683207,15.));
#26961=CARTESIAN_POINT('Ctrl Pts',(-25.5253562922582,29.356408021119,15.));
#26962=CARTESIAN_POINT('Ctrl Pts',(-25.4828076101654,29.2698007967907,15.));
#26963=CARTESIAN_POINT('Ctrl Pts',(-25.4393679214513,29.183825549991,15.));
#26964=CARTESIAN_POINT('Ctrl Pts',(-25.3948997321279,29.098589927237,15.));
#26965=CARTESIAN_POINT('Ctrl Pts',(-25.3493168206005,29.0141637699076,15.));
#26966=CARTESIAN_POINT('Ctrl Pts',(-25.3026235249214,28.9305499160476,15.));
#26967=CARTESIAN_POINT('Ctrl Pts',(-25.2549775629725,28.8476372998748,15.));
#26968=CARTESIAN_POINT('Ctrl Pts',(-25.2066127148845,28.7652594076549,15.));
#26969=CARTESIAN_POINT('Ctrl Pts',(-25.1577170374459,28.6832861366762,15.));
#26970=CARTESIAN_POINT('Ctrl Pts',(-25.108321158239,28.6017081342376,15.));
#26971=CARTESIAN_POINT('Ctrl Pts',(-25.0581926620043,28.5207164321473,15.));
#26972=CARTESIAN_POINT('Ctrl Pts',(-25.0066999111736,28.4408053900206,15.));
#26973=CARTESIAN_POINT('Ctrl Pts',(-24.9529811166897,28.3626431274892,15.));
#26974=CARTESIAN_POINT('Ctrl Pts',(-24.9075246543798,28.3020534756061,15.));
#26975=CARTESIAN_POINT('Ctrl Pts',(-24.8717258526943,28.2579420132101,15.));
#26976=CARTESIAN_POINT('Ctrl Pts',(-24.8470618363541,28.2291563988796,15.));
#26977=CARTESIAN_POINT('Ctrl Pts',(-24.8345302882955,28.2149191006269,15.));
#26978=CARTESIAN_POINT('',(-26.9738038986839,34.762248247709,0.));
#26979=CARTESIAN_POINT('Origin',(-6.66146233219319E-12,9.16871631793044E-12,
0.));
#26980=CARTESIAN_POINT('',(-24.725498909423,36.3957374383337,0.));
#26981=CARTESIAN_POINT('Origin',(-6.66146233219319E-12,9.16871631793044E-12,
0.));
#26982=CARTESIAN_POINT('',(-24.725498909423,36.3957374383337,15.));
#26983=CARTESIAN_POINT('Origin',(-6.66146233219319E-12,9.16871631793044E-12,
15.));
#26984=CARTESIAN_POINT('',(-24.725498909423,36.3957374383337,0.));
#26985=CARTESIAN_POINT('Ctrl Pts',(-19.1596907609891,32.3379313568208,0.));
#26986=CARTESIAN_POINT('Ctrl Pts',(-19.1596907609891,32.3379313568208,18.));
#26987=CARTESIAN_POINT('Ctrl Pts',(-19.1693587749508,32.3542491343753,0.));
#26988=CARTESIAN_POINT('Ctrl Pts',(-19.1693587749508,32.3542491343753,18.));
#26989=CARTESIAN_POINT('Ctrl Pts',(-19.1891139208368,32.3866012518553,0.));
#26990=CARTESIAN_POINT('Ctrl Pts',(-19.1891139208368,32.3866012518553,18.));
#26991=CARTESIAN_POINT('Ctrl Pts',(-19.2200039764927,32.4342791270009,0.));
#26992=CARTESIAN_POINT('Ctrl Pts',(-19.2200039764927,32.4342791270009,18.));
#26993=CARTESIAN_POINT('Ctrl Pts',(-19.2635813403783,32.4962340238036,0.));
#26994=CARTESIAN_POINT('Ctrl Pts',(-19.2635813403783,32.4962340238036,18.));
#26995=CARTESIAN_POINT('Ctrl Pts',(-19.3213180490743,32.5714771007861,0.));
#26996=CARTESIAN_POINT('Ctrl Pts',(-19.3213180490743,32.5714771007861,18.));
#26997=CARTESIAN_POINT('Ctrl Pts',(-19.381405831319,32.6451434870609,0.));
#26998=CARTESIAN_POINT('Ctrl Pts',(-19.381405831319,32.6451434870609,18.));
#26999=CARTESIAN_POINT('Ctrl Pts',(-19.4429429601189,32.7178463324062,0.));
#27000=CARTESIAN_POINT('Ctrl Pts',(-19.4429429601189,32.7178463324062,18.));
#27001=CARTESIAN_POINT('Ctrl Pts',(-19.5052640847974,32.7900335943248,0.));
#27002=CARTESIAN_POINT('Ctrl Pts',(-19.5052640847974,32.7900335943248,18.));
#27003=CARTESIAN_POINT('Ctrl Pts',(-19.5681157030437,32.8618672807884,0.));
#27004=CARTESIAN_POINT('Ctrl Pts',(-19.5681157030437,32.8618672807884,18.));
#27005=CARTESIAN_POINT('Ctrl Pts',(-19.6315161742485,32.9333211533788,0.));
#27006=CARTESIAN_POINT('Ctrl Pts',(-19.6315161742485,32.9333211533788,18.));
#27007=CARTESIAN_POINT('Ctrl Pts',(-19.6956473461873,33.004256563411,0.));
#27008=CARTESIAN_POINT('Ctrl Pts',(-19.6956473461873,33.004256563411,18.));
#27009=CARTESIAN_POINT('Ctrl Pts',(-19.7607398248651,33.0745026283418,0.));
#27010=CARTESIAN_POINT('Ctrl Pts',(-19.7607398248651,33.0745026283418,18.));
#27011=CARTESIAN_POINT('Ctrl Pts',(-19.8269479776239,33.1439436707661,0.));
#27012=CARTESIAN_POINT('Ctrl Pts',(-19.8269479776239,33.1439436707661,18.));
#27013=CARTESIAN_POINT('Ctrl Pts',(-19.8942704458546,33.2125746879472,0.));
#27014=CARTESIAN_POINT('Ctrl Pts',(-19.8942704458546,33.2125746879472,18.));
#27015=CARTESIAN_POINT('Ctrl Pts',(-19.9626141625205,33.2804560993213,0.));
#27016=CARTESIAN_POINT('Ctrl Pts',(-19.9626141625205,33.2804560993213,18.));
#27017=CARTESIAN_POINT('Ctrl Pts',(-20.0318342617212,33.3476854048385,0.));
#27018=CARTESIAN_POINT('Ctrl Pts',(-20.0318342617212,33.3476854048385,18.));
#27019=CARTESIAN_POINT('Ctrl Pts',(-20.1017803986381,33.4143643679979,0.));
#27020=CARTESIAN_POINT('Ctrl Pts',(-20.1017803986381,33.4143643679979,18.));
#27021=CARTESIAN_POINT('Ctrl Pts',(-20.1723475154533,33.480563024813,0.));
#27022=CARTESIAN_POINT('Ctrl Pts',(-20.1723475154533,33.480563024813,18.));
#27023=CARTESIAN_POINT('Ctrl Pts',(-20.243500298383,33.5463023319603,0.));
#27024=CARTESIAN_POINT('Ctrl Pts',(-20.243500298383,33.5463023319603,18.));
#27025=CARTESIAN_POINT('Ctrl Pts',(-20.3152448035298,33.6115742164079,0.));
#27026=CARTESIAN_POINT('Ctrl Pts',(-20.3152448035298,33.6115742164079,18.));
#27027=CARTESIAN_POINT('Ctrl Pts',(-20.3876111773341,33.6763537716992,0.));
#27028=CARTESIAN_POINT('Ctrl Pts',(-20.3876111773341,33.6763537716992,18.));
#27029=CARTESIAN_POINT('Ctrl Pts',(-20.4606334536183,33.7406135254083,0.));
#27030=CARTESIAN_POINT('Ctrl Pts',(-20.4606334536183,33.7406135254083,18.));
#27031=CARTESIAN_POINT('Ctrl Pts',(-20.5343269914034,33.8043393734971,0.));
#27032=CARTESIAN_POINT('Ctrl Pts',(-20.5343269914034,33.8043393734971,18.));
#27033=CARTESIAN_POINT('Ctrl Pts',(-20.6086800574386,33.8675365150454,0.));
#27034=CARTESIAN_POINT('Ctrl Pts',(-20.6086800574386,33.8675365150454,18.));
#27035=CARTESIAN_POINT('Ctrl Pts',(-20.683665762903,33.9302209962425,0.));
#27036=CARTESIAN_POINT('Ctrl Pts',(-20.683665762903,33.9302209962425,18.));
#27037=CARTESIAN_POINT('Ctrl Pts',(-20.7592491770603,33.9924146647395,0.));
#27038=CARTESIAN_POINT('Ctrl Pts',(-20.7592491770603,33.9924146647395,18.));
#27039=CARTESIAN_POINT('Ctrl Pts',(-20.8353957068415,34.0541392299678,0.));
#27040=CARTESIAN_POINT('Ctrl Pts',(-20.8353957068415,34.0541392299678,18.));
#27041=CARTESIAN_POINT('Ctrl Pts',(-20.9120805673809,34.1154095510973,0.));
#27042=CARTESIAN_POINT('Ctrl Pts',(-20.9120805673809,34.1154095510973,18.));
#27043=CARTESIAN_POINT('Ctrl Pts',(-20.9892914622612,34.176231731809,0.));
#27044=CARTESIAN_POINT('Ctrl Pts',(-20.9892914622612,34.176231731809,18.));
#27045=CARTESIAN_POINT('Ctrl Pts',(-21.0670234747355,34.2366067284279,0.));
#27046=CARTESIAN_POINT('Ctrl Pts',(-21.0670234747355,34.2366067284279,18.));
#27047=CARTESIAN_POINT('Ctrl Pts',(-21.1452759244399,34.2965325673384,0.));
#27048=CARTESIAN_POINT('Ctrl Pts',(-21.1452759244399,34.2965325673384,18.));
#27049=CARTESIAN_POINT('Ctrl Pts',(-21.2240487218079,34.3560069185815,0.));
#27050=CARTESIAN_POINT('Ctrl Pts',(-21.2240487218079,34.3560069185815,18.));
#27051=CARTESIAN_POINT('Ctrl Pts',(-21.3033382073239,34.4150300340623,0.));
#27052=CARTESIAN_POINT('Ctrl Pts',(-21.3033382073239,34.4150300340623,18.));
#27053=CARTESIAN_POINT('Ctrl Pts',(-21.3831361300104,34.4736054662052,0.));
#27054=CARTESIAN_POINT('Ctrl Pts',(-21.3831361300104,34.4736054662052,18.));
#27055=CARTESIAN_POINT('Ctrl Pts',(-21.4634317666005,34.5317385658329,0.));
#27056=CARTESIAN_POINT('Ctrl Pts',(-21.4634317666005,34.5317385658329,18.));
#27057=CARTESIAN_POINT('Ctrl Pts',(-21.5442132160757,34.5894355639082,0.));
#27058=CARTESIAN_POINT('Ctrl Pts',(-21.5442132160757,34.5894355639082,18.));
#27059=CARTESIAN_POINT('Ctrl Pts',(-21.6254689009796,34.6467025072367,0.));
#27060=CARTESIAN_POINT('Ctrl Pts',(-21.6254689009796,34.6467025072367,18.));
#27061=CARTESIAN_POINT('Ctrl Pts',(-21.7071892844497,34.7035440429025,0.));
#27062=CARTESIAN_POINT('Ctrl Pts',(-21.7071892844497,34.7035440429025,18.));
#27063=CARTESIAN_POINT('Ctrl Pts',(-21.7893672401137,34.7599631530844,0.));
#27064=CARTESIAN_POINT('Ctrl Pts',(-21.7893672401137,34.7599631530844,18.));
#27065=CARTESIAN_POINT('Ctrl Pts',(-21.8719971302817,34.8159618014436,0.));
#27066=CARTESIAN_POINT('Ctrl Pts',(-21.8719971302817,34.8159618014436,18.));
#27067=CARTESIAN_POINT('Ctrl Pts',(-21.9550742217675,34.8715413418101,0.));
#27068=CARTESIAN_POINT('Ctrl Pts',(-21.9550742217675,34.8715413418101,18.));
#27069=CARTESIAN_POINT('Ctrl Pts',(-22.0385940162683,34.9267029879922,0.));
#27070=CARTESIAN_POINT('Ctrl Pts',(-22.0385940162683,34.9267029879922,18.));
#27071=CARTESIAN_POINT('Ctrl Pts',(-22.1225514798584,34.9814483545602,0.));
#27072=CARTESIAN_POINT('Ctrl Pts',(-22.1225514798584,34.9814483545602,18.));
#27073=CARTESIAN_POINT('Ctrl Pts',(-22.2069408519232,35.0357795922459,0.));
#27074=CARTESIAN_POINT('Ctrl Pts',(-22.2069408519232,35.0357795922459,18.));
#27075=CARTESIAN_POINT('Ctrl Pts',(-22.2917560356803,35.0896991159359,0.));
#27076=CARTESIAN_POINT('Ctrl Pts',(-22.2917560356803,35.0896991159359,18.));
#27077=CARTESIAN_POINT('Ctrl Pts',(-22.3769908340843,35.1432094422642,0.));
#27078=CARTESIAN_POINT('Ctrl Pts',(-22.3769908340843,35.1432094422642,18.));
#27079=CARTESIAN_POINT('Ctrl Pts',(-22.4626392230023,35.1963130003352,0.));
#27080=CARTESIAN_POINT('Ctrl Pts',(-22.4626392230023,35.1963130003352,18.));
#27081=CARTESIAN_POINT('Ctrl Pts',(-22.5486956608909,35.2490119207975,0.));
#27082=CARTESIAN_POINT('Ctrl Pts',(-22.5486956608909,35.2490119207975,18.));
#27083=CARTESIAN_POINT('Ctrl Pts',(-22.635155167154,35.3013079759252,0.));
#27084=CARTESIAN_POINT('Ctrl Pts',(-22.635155167154,35.3013079759252,18.));
#27085=CARTESIAN_POINT('Ctrl Pts',(-22.7220131336912,35.3532026952313,0.));
#27086=CARTESIAN_POINT('Ctrl Pts',(-22.7220131336912,35.3532026952313,18.));
#27087=CARTESIAN_POINT('Ctrl Pts',(-22.8092652000706,35.4046974393492,0.));
#27088=CARTESIAN_POINT('Ctrl Pts',(-22.8092652000706,35.4046974393492,18.));
#27089=CARTESIAN_POINT('Ctrl Pts',(-22.8969071125089,35.4557934871468,0.));
#27090=CARTESIAN_POINT('Ctrl Pts',(-22.8969071125089,35.4557934871468,18.));
#27091=CARTESIAN_POINT('Ctrl Pts',(-22.9849345572033,35.5064921357308,0.));
#27092=CARTESIAN_POINT('Ctrl Pts',(-22.9849345572033,35.5064921357308,18.));
#27093=CARTESIAN_POINT('Ctrl Pts',(-23.0733431097058,35.5567947408311,0.));
#27094=CARTESIAN_POINT('Ctrl Pts',(-23.0733431097058,35.5567947408311,18.));
#27095=CARTESIAN_POINT('Ctrl Pts',(-23.1621283508111,35.6067026687722,0.));
#27096=CARTESIAN_POINT('Ctrl Pts',(-23.1621283508111,35.6067026687722,18.));
#27097=CARTESIAN_POINT('Ctrl Pts',(-23.2512859425032,35.6562172725207,0.));
#27098=CARTESIAN_POINT('Ctrl Pts',(-23.2512859425032,35.6562172725207,18.));
#27099=CARTESIAN_POINT('Ctrl Pts',(-23.3408117088761,35.7053398620512,0.));
#27100=CARTESIAN_POINT('Ctrl Pts',(-23.3408117088761,35.7053398620512,18.));
#27101=CARTESIAN_POINT('Ctrl Pts',(-23.4307017328227,35.7540716771372,0.));
#27102=CARTESIAN_POINT('Ctrl Pts',(-23.4307017328227,35.7540716771372,18.));
#27103=CARTESIAN_POINT('Ctrl Pts',(-23.5209523746427,35.8024138716897,0.));
#27104=CARTESIAN_POINT('Ctrl Pts',(-23.5209523746427,35.8024138716897,18.));
#27105=CARTESIAN_POINT('Ctrl Pts',(-23.611560139948,35.8503675222885,0.));
#27106=CARTESIAN_POINT('Ctrl Pts',(-23.611560139948,35.8503675222885,18.));
#27107=CARTESIAN_POINT('Ctrl Pts',(-23.7025215735353,35.8979336336837,0.));
#27108=CARTESIAN_POINT('Ctrl Pts',(-23.7025215735353,35.8979336336837,18.));
#27109=CARTESIAN_POINT('Ctrl Pts',(-23.7938331508737,35.9451131482488,0.));
#27110=CARTESIAN_POINT('Ctrl Pts',(-23.7938331508737,35.9451131482488,18.));
#27111=CARTESIAN_POINT('Ctrl Pts',(-23.8854911428946,35.991906956547,0.));
#27112=CARTESIAN_POINT('Ctrl Pts',(-23.8854911428946,35.991906956547,18.));
#27113=CARTESIAN_POINT('Ctrl Pts',(-23.9774915680089,36.0383159101254,0.));
#27114=CARTESIAN_POINT('Ctrl Pts',(-23.9774915680089,36.0383159101254,18.));
#27115=CARTESIAN_POINT('Ctrl Pts',(-24.0698304230588,36.0843408347974,0.));
#27116=CARTESIAN_POINT('Ctrl Pts',(-24.0698304230588,36.0843408347974,18.));
#27117=CARTESIAN_POINT('Ctrl Pts',(-24.1625038657964,36.1299825471271,0.));
#27118=CARTESIAN_POINT('Ctrl Pts',(-24.1625038657964,36.1299825471271,18.));
#27119=CARTESIAN_POINT('Ctrl Pts',(-24.2555084095332,36.1752418704833,0.));
#27120=CARTESIAN_POINT('Ctrl Pts',(-24.2555084095332,36.1752418704833,18.));
#27121=CARTESIAN_POINT('Ctrl Pts',(-24.3488411214068,36.2201196586697,0.));
#27122=CARTESIAN_POINT('Ctrl Pts',(-24.3488411214068,36.2201196586697,18.));
#27123=CARTESIAN_POINT('Ctrl Pts',(-24.4424997853605,36.2646168058396,0.));
#27124=CARTESIAN_POINT('Ctrl Pts',(-24.4424997853605,36.2646168058396,18.));
#27125=CARTESIAN_POINT('Ctrl Pts',(-24.5364828082556,36.308734152297,0.));
#27126=CARTESIAN_POINT('Ctrl Pts',(-24.5364828082556,36.308734152297,18.));
#27127=CARTESIAN_POINT('Ctrl Pts',(-24.6119278836614,36.3437247532369,0.));
#27128=CARTESIAN_POINT('Ctrl Pts',(-24.6119278836614,36.3437247532369,18.));
#27129=CARTESIAN_POINT('Ctrl Pts',(-24.6686569322616,36.369797330215,0.));
#27130=CARTESIAN_POINT('Ctrl Pts',(-24.6686569322616,36.369797330215,18.));
#27131=CARTESIAN_POINT('Ctrl Pts',(-24.7065408286023,36.3871033517098,0.));
#27132=CARTESIAN_POINT('Ctrl Pts',(-24.7065408286023,36.3871033517098,18.));
#27133=CARTESIAN_POINT('Ctrl Pts',(-24.725498909423,36.3957374383337,0.));
#27134=CARTESIAN_POINT('Ctrl Pts',(-24.725498909423,36.3957374383337,18.));
#27135=CARTESIAN_POINT('Ctrl Pts',(-19.1596907609891,32.3379313568208,0.));
#27136=CARTESIAN_POINT('Ctrl Pts',(-19.1693587749508,32.3542491343753,0.));
#27137=CARTESIAN_POINT('Ctrl Pts',(-19.1891139208368,32.3866012518553,0.));
#27138=CARTESIAN_POINT('Ctrl Pts',(-19.2200039764927,32.4342791270009,0.));
#27139=CARTESIAN_POINT('Ctrl Pts',(-19.2635813403783,32.4962340238036,0.));
#27140=CARTESIAN_POINT('Ctrl Pts',(-19.3213180490743,32.5714771007861,0.));
#27141=CARTESIAN_POINT('Ctrl Pts',(-19.381405831319,32.6451434870609,0.));
#27142=CARTESIAN_POINT('Ctrl Pts',(-19.4429429601189,32.7178463324062,0.));
#27143=CARTESIAN_POINT('Ctrl Pts',(-19.5052640847974,32.7900335943248,0.));
#27144=CARTESIAN_POINT('Ctrl Pts',(-19.5681157030437,32.8618672807884,0.));
#27145=CARTESIAN_POINT('Ctrl Pts',(-19.6315161742485,32.9333211533788,0.));
#27146=CARTESIAN_POINT('Ctrl Pts',(-19.6956473461873,33.004256563411,0.));
#27147=CARTESIAN_POINT('Ctrl Pts',(-19.7607398248651,33.0745026283418,0.));
#27148=CARTESIAN_POINT('Ctrl Pts',(-19.8269479776239,33.1439436707661,0.));
#27149=CARTESIAN_POINT('Ctrl Pts',(-19.8942704458546,33.2125746879472,0.));
#27150=CARTESIAN_POINT('Ctrl Pts',(-19.9626141625205,33.2804560993213,0.));
#27151=CARTESIAN_POINT('Ctrl Pts',(-20.0318342617212,33.3476854048385,0.));
#27152=CARTESIAN_POINT('Ctrl Pts',(-20.1017803986381,33.4143643679979,0.));
#27153=CARTESIAN_POINT('Ctrl Pts',(-20.1723475154533,33.480563024813,0.));
#27154=CARTESIAN_POINT('Ctrl Pts',(-20.243500298383,33.5463023319603,0.));
#27155=CARTESIAN_POINT('Ctrl Pts',(-20.3152448035298,33.6115742164079,0.));
#27156=CARTESIAN_POINT('Ctrl Pts',(-20.3876111773341,33.6763537716992,0.));
#27157=CARTESIAN_POINT('Ctrl Pts',(-20.4606334536183,33.7406135254083,0.));
#27158=CARTESIAN_POINT('Ctrl Pts',(-20.5343269914034,33.8043393734971,0.));
#27159=CARTESIAN_POINT('Ctrl Pts',(-20.6086800574386,33.8675365150454,0.));
#27160=CARTESIAN_POINT('Ctrl Pts',(-20.683665762903,33.9302209962425,0.));
#27161=CARTESIAN_POINT('Ctrl Pts',(-20.7592491770603,33.9924146647395,0.));
#27162=CARTESIAN_POINT('Ctrl Pts',(-20.8353957068415,34.0541392299678,0.));
#27163=CARTESIAN_POINT('Ctrl Pts',(-20.9120805673809,34.1154095510973,0.));
#27164=CARTESIAN_POINT('Ctrl Pts',(-20.9892914622612,34.176231731809,0.));
#27165=CARTESIAN_POINT('Ctrl Pts',(-21.0670234747355,34.2366067284279,0.));
#27166=CARTESIAN_POINT('Ctrl Pts',(-21.1452759244399,34.2965325673384,0.));
#27167=CARTESIAN_POINT('Ctrl Pts',(-21.2240487218079,34.3560069185815,0.));
#27168=CARTESIAN_POINT('Ctrl Pts',(-21.3033382073239,34.4150300340623,0.));
#27169=CARTESIAN_POINT('Ctrl Pts',(-21.3831361300104,34.4736054662052,0.));
#27170=CARTESIAN_POINT('Ctrl Pts',(-21.4634317666005,34.5317385658329,0.));
#27171=CARTESIAN_POINT('Ctrl Pts',(-21.5442132160757,34.5894355639082,0.));
#27172=CARTESIAN_POINT('Ctrl Pts',(-21.6254689009796,34.6467025072367,0.));
#27173=CARTESIAN_POINT('Ctrl Pts',(-21.7071892844497,34.7035440429025,0.));
#27174=CARTESIAN_POINT('Ctrl Pts',(-21.7893672401137,34.7599631530844,0.));
#27175=CARTESIAN_POINT('Ctrl Pts',(-21.8719971302817,34.8159618014436,0.));
#27176=CARTESIAN_POINT('Ctrl Pts',(-21.9550742217675,34.8715413418101,0.));
#27177=CARTESIAN_POINT('Ctrl Pts',(-22.0385940162683,34.9267029879922,0.));
#27178=CARTESIAN_POINT('Ctrl Pts',(-22.1225514798584,34.9814483545602,0.));
#27179=CARTESIAN_POINT('Ctrl Pts',(-22.2069408519232,35.0357795922459,0.));
#27180=CARTESIAN_POINT('Ctrl Pts',(-22.2917560356803,35.0896991159359,0.));
#27181=CARTESIAN_POINT('Ctrl Pts',(-22.3769908340843,35.1432094422642,0.));
#27182=CARTESIAN_POINT('Ctrl Pts',(-22.4626392230023,35.1963130003352,0.));
#27183=CARTESIAN_POINT('Ctrl Pts',(-22.5486956608909,35.2490119207975,0.));
#27184=CARTESIAN_POINT('Ctrl Pts',(-22.635155167154,35.3013079759252,0.));
#27185=CARTESIAN_POINT('Ctrl Pts',(-22.7220131336912,35.3532026952313,0.));
#27186=CARTESIAN_POINT('Ctrl Pts',(-22.8092652000706,35.4046974393492,0.));
#27187=CARTESIAN_POINT('Ctrl Pts',(-22.8969071125089,35.4557934871468,0.));
#27188=CARTESIAN_POINT('Ctrl Pts',(-22.9849345572033,35.5064921357308,0.));
#27189=CARTESIAN_POINT('Ctrl Pts',(-23.0733431097058,35.5567947408311,0.));
#27190=CARTESIAN_POINT('Ctrl Pts',(-23.1621283508111,35.6067026687722,0.));
#27191=CARTESIAN_POINT('Ctrl Pts',(-23.2512859425032,35.6562172725207,0.));
#27192=CARTESIAN_POINT('Ctrl Pts',(-23.3408117088761,35.7053398620512,0.));
#27193=CARTESIAN_POINT('Ctrl Pts',(-23.4307017328227,35.7540716771372,0.));
#27194=CARTESIAN_POINT('Ctrl Pts',(-23.5209523746427,35.8024138716897,0.));
#27195=CARTESIAN_POINT('Ctrl Pts',(-23.611560139948,35.8503675222885,0.));
#27196=CARTESIAN_POINT('Ctrl Pts',(-23.7025215735353,35.8979336336837,0.));
#27197=CARTESIAN_POINT('Ctrl Pts',(-23.7938331508737,35.9451131482488,0.));
#27198=CARTESIAN_POINT('Ctrl Pts',(-23.8854911428946,35.991906956547,0.));
#27199=CARTESIAN_POINT('Ctrl Pts',(-23.9774915680089,36.0383159101254,0.));
#27200=CARTESIAN_POINT('Ctrl Pts',(-24.0698304230588,36.0843408347974,0.));
#27201=CARTESIAN_POINT('Ctrl Pts',(-24.1625038657964,36.1299825471271,0.));
#27202=CARTESIAN_POINT('Ctrl Pts',(-24.2555084095332,36.1752418704833,0.));
#27203=CARTESIAN_POINT('Ctrl Pts',(-24.3488411214068,36.2201196586697,0.));
#27204=CARTESIAN_POINT('Ctrl Pts',(-24.4612315181512,36.2735162352736,0.));
#27205=CARTESIAN_POINT('Ctrl Pts',(-24.5552956307817,36.3175386315529,0.));
#27206=CARTESIAN_POINT('Ctrl Pts',(-24.630805301288,36.3524534604649,0.));
#27207=CARTESIAN_POINT('Ctrl Pts',(-24.6875827477484,36.37846926509,0.));
#27208=CARTESIAN_POINT('Ctrl Pts',(-24.725498909423,36.3957374383337,0.));
#27209=CARTESIAN_POINT('Ctrl Pts',(-19.1596907609891,32.3379313568208,15.));
#27210=CARTESIAN_POINT('Ctrl Pts',(-19.1693587749508,32.3542491343753,15.));
#27211=CARTESIAN_POINT('Ctrl Pts',(-19.1891139208368,32.3866012518553,15.));
#27212=CARTESIAN_POINT('Ctrl Pts',(-19.2200039764927,32.4342791270009,15.));
#27213=CARTESIAN_POINT('Ctrl Pts',(-19.2635813403783,32.4962340238036,15.));
#27214=CARTESIAN_POINT('Ctrl Pts',(-19.3213180490743,32.5714771007861,15.));
#27215=CARTESIAN_POINT('Ctrl Pts',(-19.381405831319,32.6451434870609,15.));
#27216=CARTESIAN_POINT('Ctrl Pts',(-19.4429429601189,32.7178463324062,15.));
#27217=CARTESIAN_POINT('Ctrl Pts',(-19.5052640847974,32.7900335943248,15.));
#27218=CARTESIAN_POINT('Ctrl Pts',(-19.5681157030437,32.8618672807884,15.));
#27219=CARTESIAN_POINT('Ctrl Pts',(-19.6315161742485,32.9333211533788,15.));
#27220=CARTESIAN_POINT('Ctrl Pts',(-19.6956473461873,33.004256563411,15.));
#27221=CARTESIAN_POINT('Ctrl Pts',(-19.7607398248651,33.0745026283418,15.));
#27222=CARTESIAN_POINT('Ctrl Pts',(-19.8269479776239,33.1439436707661,15.));
#27223=CARTESIAN_POINT('Ctrl Pts',(-19.8942704458546,33.2125746879472,15.));
#27224=CARTESIAN_POINT('Ctrl Pts',(-19.9626141625205,33.2804560993213,15.));
#27225=CARTESIAN_POINT('Ctrl Pts',(-20.0318342617212,33.3476854048385,15.));
#27226=CARTESIAN_POINT('Ctrl Pts',(-20.1017803986381,33.4143643679979,15.));
#27227=CARTESIAN_POINT('Ctrl Pts',(-20.1723475154533,33.480563024813,15.));
#27228=CARTESIAN_POINT('Ctrl Pts',(-20.243500298383,33.5463023319603,15.));
#27229=CARTESIAN_POINT('Ctrl Pts',(-20.3152448035298,33.6115742164079,15.));
#27230=CARTESIAN_POINT('Ctrl Pts',(-20.3876111773341,33.6763537716992,15.));
#27231=CARTESIAN_POINT('Ctrl Pts',(-20.4606334536183,33.7406135254083,15.));
#27232=CARTESIAN_POINT('Ctrl Pts',(-20.5343269914034,33.8043393734971,15.));
#27233=CARTESIAN_POINT('Ctrl Pts',(-20.6086800574386,33.8675365150454,15.));
#27234=CARTESIAN_POINT('Ctrl Pts',(-20.683665762903,33.9302209962425,15.));
#27235=CARTESIAN_POINT('Ctrl Pts',(-20.7592491770603,33.9924146647395,15.));
#27236=CARTESIAN_POINT('Ctrl Pts',(-20.8353957068415,34.0541392299678,15.));
#27237=CARTESIAN_POINT('Ctrl Pts',(-20.9120805673809,34.1154095510973,15.));
#27238=CARTESIAN_POINT('Ctrl Pts',(-20.9892914622612,34.176231731809,15.));
#27239=CARTESIAN_POINT('Ctrl Pts',(-21.0670234747355,34.2366067284279,15.));
#27240=CARTESIAN_POINT('Ctrl Pts',(-21.1452759244399,34.2965325673384,15.));
#27241=CARTESIAN_POINT('Ctrl Pts',(-21.2240487218079,34.3560069185815,15.));
#27242=CARTESIAN_POINT('Ctrl Pts',(-21.3033382073239,34.4150300340623,15.));
#27243=CARTESIAN_POINT('Ctrl Pts',(-21.3831361300104,34.4736054662052,15.));
#27244=CARTESIAN_POINT('Ctrl Pts',(-21.4634317666005,34.5317385658329,15.));
#27245=CARTESIAN_POINT('Ctrl Pts',(-21.5442132160757,34.5894355639082,15.));
#27246=CARTESIAN_POINT('Ctrl Pts',(-21.6254689009796,34.6467025072367,15.));
#27247=CARTESIAN_POINT('Ctrl Pts',(-21.7071892844497,34.7035440429025,15.));
#27248=CARTESIAN_POINT('Ctrl Pts',(-21.7893672401137,34.7599631530844,15.));
#27249=CARTESIAN_POINT('Ctrl Pts',(-21.8719971302817,34.8159618014436,15.));
#27250=CARTESIAN_POINT('Ctrl Pts',(-21.9550742217675,34.8715413418101,15.));
#27251=CARTESIAN_POINT('Ctrl Pts',(-22.0385940162683,34.9267029879922,15.));
#27252=CARTESIAN_POINT('Ctrl Pts',(-22.1225514798584,34.9814483545602,15.));
#27253=CARTESIAN_POINT('Ctrl Pts',(-22.2069408519232,35.0357795922459,15.));
#27254=CARTESIAN_POINT('Ctrl Pts',(-22.2917560356803,35.0896991159359,15.));
#27255=CARTESIAN_POINT('Ctrl Pts',(-22.3769908340843,35.1432094422642,15.));
#27256=CARTESIAN_POINT('Ctrl Pts',(-22.4626392230023,35.1963130003352,15.));
#27257=CARTESIAN_POINT('Ctrl Pts',(-22.5486956608909,35.2490119207975,15.));
#27258=CARTESIAN_POINT('Ctrl Pts',(-22.635155167154,35.3013079759252,15.));
#27259=CARTESIAN_POINT('Ctrl Pts',(-22.7220131336912,35.3532026952313,15.));
#27260=CARTESIAN_POINT('Ctrl Pts',(-22.8092652000706,35.4046974393492,15.));
#27261=CARTESIAN_POINT('Ctrl Pts',(-22.8969071125089,35.4557934871468,15.));
#27262=CARTESIAN_POINT('Ctrl Pts',(-22.9849345572033,35.5064921357308,15.));
#27263=CARTESIAN_POINT('Ctrl Pts',(-23.0733431097058,35.5567947408311,15.));
#27264=CARTESIAN_POINT('Ctrl Pts',(-23.1621283508111,35.6067026687722,15.));
#27265=CARTESIAN_POINT('Ctrl Pts',(-23.2512859425032,35.6562172725207,15.));
#27266=CARTESIAN_POINT('Ctrl Pts',(-23.3408117088761,35.7053398620512,15.));
#27267=CARTESIAN_POINT('Ctrl Pts',(-23.4307017328227,35.7540716771372,15.));
#27268=CARTESIAN_POINT('Ctrl Pts',(-23.5209523746427,35.8024138716897,15.));
#27269=CARTESIAN_POINT('Ctrl Pts',(-23.611560139948,35.8503675222885,15.));
#27270=CARTESIAN_POINT('Ctrl Pts',(-23.7025215735353,35.8979336336837,15.));
#27271=CARTESIAN_POINT('Ctrl Pts',(-23.7938331508737,35.9451131482488,15.));
#27272=CARTESIAN_POINT('Ctrl Pts',(-23.8854911428946,35.991906956547,15.));
#27273=CARTESIAN_POINT('Ctrl Pts',(-23.9774915680089,36.0383159101254,15.));
#27274=CARTESIAN_POINT('Ctrl Pts',(-24.0698304230588,36.0843408347974,15.));
#27275=CARTESIAN_POINT('Ctrl Pts',(-24.1625038657964,36.1299825471271,15.));
#27276=CARTESIAN_POINT('Ctrl Pts',(-24.2555084095332,36.1752418704833,15.));
#27277=CARTESIAN_POINT('Ctrl Pts',(-24.3488411214068,36.2201196586697,15.));
#27278=CARTESIAN_POINT('Ctrl Pts',(-24.4612315181512,36.2735162352736,15.));
#27279=CARTESIAN_POINT('Ctrl Pts',(-24.5552956307817,36.3175386315529,15.));
#27280=CARTESIAN_POINT('Ctrl Pts',(-24.630805301288,36.3524534604649,15.));
#27281=CARTESIAN_POINT('Ctrl Pts',(-24.6875827477484,36.37846926509,15.));
#27282=CARTESIAN_POINT('Ctrl Pts',(-24.725498909423,36.3957374383337,15.));
#27283=CARTESIAN_POINT('Ctrl Pts',(-14.911486495888,41.396226524684,0.));
#27284=CARTESIAN_POINT('Ctrl Pts',(-14.911486495888,41.396226524684,18.));
#27285=CARTESIAN_POINT('Ctrl Pts',(-14.9156446533966,41.3758141263348,0.));
#27286=CARTESIAN_POINT('Ctrl Pts',(-14.9156446533966,41.3758141263348,18.));
#27287=CARTESIAN_POINT('Ctrl Pts',(-14.9239113834707,41.3349931861715,0.));
#27288=CARTESIAN_POINT('Ctrl Pts',(-14.9239113834707,41.3349931861715,18.));
#27289=CARTESIAN_POINT('Ctrl Pts',(-14.936162723752,41.2737733455422,0.));
#27290=CARTESIAN_POINT('Ctrl Pts',(-14.936162723752,41.2737733455422,18.));
#27291=CARTESIAN_POINT('Ctrl Pts',(-14.9522002356298,41.1921700381957,0.));
#27292=CARTESIAN_POINT('Ctrl Pts',(-14.9522002356298,41.1921700381957,18.));
#27293=CARTESIAN_POINT('Ctrl Pts',(-14.9717503874227,41.0902046498729,0.));
#27294=CARTESIAN_POINT('Ctrl Pts',(-14.9717503874227,41.0902046498729,18.));
#27295=CARTESIAN_POINT('Ctrl Pts',(-14.9908026205824,40.9882784321884,0.));
#27296=CARTESIAN_POINT('Ctrl Pts',(-14.9908026205824,40.9882784321884,18.));
#27297=CARTESIAN_POINT('Ctrl Pts',(-15.0093553188655,40.8863921801,0.));
#27298=CARTESIAN_POINT('Ctrl Pts',(-15.0093553188655,40.8863921801,18.));
#27299=CARTESIAN_POINT('Ctrl Pts',(-15.0274064563211,40.7845471608654,0.));
#27300=CARTESIAN_POINT('Ctrl Pts',(-15.0274064563211,40.7845471608654,18.));
#27301=CARTESIAN_POINT('Ctrl Pts',(-15.0449536183143,40.6827452453667,0.));
#27302=CARTESIAN_POINT('Ctrl Pts',(-15.0449536183143,40.6827452453667,18.));
#27303=CARTESIAN_POINT('Ctrl Pts',(-15.0619940893017,40.58098877043,0.));
#27304=CARTESIAN_POINT('Ctrl Pts',(-15.0619940893017,40.58098877043,18.));
#27305=CARTESIAN_POINT('Ctrl Pts',(-15.0785249502524,40.4792803645352,0.));
#27306=CARTESIAN_POINT('Ctrl Pts',(-15.0785249502524,40.4792803645352,18.));
#27307=CARTESIAN_POINT('Ctrl Pts',(-15.0945431800723,40.3776227809037,0.));
#27308=CARTESIAN_POINT('Ctrl Pts',(-15.0945431800723,40.3776227809037,18.));
#27309=CARTESIAN_POINT('Ctrl Pts',(-15.1100457495259,40.2760187401821,0.));
#27310=CARTESIAN_POINT('Ctrl Pts',(-15.1100457495259,40.2760187401821,18.));
#27311=CARTESIAN_POINT('Ctrl Pts',(-15.1250297462408,40.1744707357902,0.));
#27312=CARTESIAN_POINT('Ctrl Pts',(-15.1250297462408,40.1744707357902,18.));
#27313=CARTESIAN_POINT('Ctrl Pts',(-15.1394923361537,40.0729810652204,0.));
#27314=CARTESIAN_POINT('Ctrl Pts',(-15.1394923361537,40.0729810652204,18.));
#27315=CARTESIAN_POINT('Ctrl Pts',(-15.1534306754871,39.9715519332134,0.));
#27316=CARTESIAN_POINT('Ctrl Pts',(-15.1534306754871,39.9715519332134,18.));
#27317=CARTESIAN_POINT('Ctrl Pts',(-15.1668418393198,39.8701855339908,0.));
#27318=CARTESIAN_POINT('Ctrl Pts',(-15.1668418393198,39.8701855339908,18.));
#27319=CARTESIAN_POINT('Ctrl Pts',(-15.1797227547561,39.7688841338802,0.));
#27320=CARTESIAN_POINT('Ctrl Pts',(-15.1797227547561,39.7688841338802,18.));
#27321=CARTESIAN_POINT('Ctrl Pts',(-15.1920701163803,39.6676501731673,0.));
#27322=CARTESIAN_POINT('Ctrl Pts',(-15.1920701163803,39.6676501731673,18.));
#27323=CARTESIAN_POINT('Ctrl Pts',(-15.2038804098649,39.5664862602472,0.));
#27324=CARTESIAN_POINT('Ctrl Pts',(-15.2038804098649,39.5664862602472,18.));
#27325=CARTESIAN_POINT('Ctrl Pts',(-15.2151499908149,39.4653951093947,0.));
#27326=CARTESIAN_POINT('Ctrl Pts',(-15.2151499908149,39.4653951093947,18.));
#27327=CARTESIAN_POINT('Ctrl Pts',(-15.2258751563069,39.3643794927167,0.));
#27328=CARTESIAN_POINT('Ctrl Pts',(-15.2258751563069,39.3643794927167,18.));
#27329=CARTESIAN_POINT('Ctrl Pts',(-15.2360522089072,39.2634421927888,0.));
#27330=CARTESIAN_POINT('Ctrl Pts',(-15.2360522089072,39.2634421927888,18.));
#27331=CARTESIAN_POINT('Ctrl Pts',(-15.2456775636447,39.1625859371304,0.));
#27332=CARTESIAN_POINT('Ctrl Pts',(-15.2456775636447,39.1625859371304,18.));
#27333=CARTESIAN_POINT('Ctrl Pts',(-15.2547476855825,39.061813415425,0.));
#27334=CARTESIAN_POINT('Ctrl Pts',(-15.2547476855825,39.061813415425,18.));
#27335=CARTESIAN_POINT('Ctrl Pts',(-15.2632589109473,38.9611273555758,0.));
#27336=CARTESIAN_POINT('Ctrl Pts',(-15.2632589109473,38.9611273555758,18.));
#27337=CARTESIAN_POINT('Ctrl Pts',(-15.2712072937639,38.860530586589,0.));
#27338=CARTESIAN_POINT('Ctrl Pts',(-15.2712072937639,38.860530586589,18.));
#27339=CARTESIAN_POINT('Ctrl Pts',(-15.2785884727112,38.7600260961351,0.));
#27340=CARTESIAN_POINT('Ctrl Pts',(-15.2785884727112,38.7600260961351,18.));
#27341=CARTESIAN_POINT('Ctrl Pts',(-15.2853974668211,38.659617115053,0.));
#27342=CARTESIAN_POINT('Ctrl Pts',(-15.2853974668211,38.659617115053,18.));
#27343=CARTESIAN_POINT('Ctrl Pts',(-15.2916287700102,38.5593070891769,0.));
#27344=CARTESIAN_POINT('Ctrl Pts',(-15.2916287700102,38.5593070891769,18.));
#27345=CARTESIAN_POINT('Ctrl Pts',(-15.2972767037469,38.4590995527814,0.));
#27346=CARTESIAN_POINT('Ctrl Pts',(-15.2972767037469,38.4590995527814,18.));
#27347=CARTESIAN_POINT('Ctrl Pts',(-15.3023357307483,38.3589980188324,0.));
#27348=CARTESIAN_POINT('Ctrl Pts',(-15.3023357307483,38.3589980188324,18.));
#27349=CARTESIAN_POINT('Ctrl Pts',(-15.3068007250314,38.2590058835965,0.));
#27350=CARTESIAN_POINT('Ctrl Pts',(-15.3068007250314,38.2590058835965,18.));
#27351=CARTESIAN_POINT('Ctrl Pts',(-15.310667421514,38.1591262705847,0.));
#27352=CARTESIAN_POINT('Ctrl Pts',(-15.310667421514,38.1591262705847,18.));
#27353=CARTESIAN_POINT('Ctrl Pts',(-15.3139321941687,38.0593621055415,0.));
#27354=CARTESIAN_POINT('Ctrl Pts',(-15.3139321941687,38.0593621055415,18.));
#27355=CARTESIAN_POINT('Ctrl Pts',(-15.3165911656268,37.959716421934,0.));
#27356=CARTESIAN_POINT('Ctrl Pts',(-15.3165911656268,37.959716421934,18.));
#27357=CARTESIAN_POINT('Ctrl Pts',(-15.3186394335023,37.8601926265378,0.));
#27358=CARTESIAN_POINT('Ctrl Pts',(-15.3186394335023,37.8601926265378,18.));
#27359=CARTESIAN_POINT('Ctrl Pts',(-15.320070396385,37.7607947318286,0.));
#27360=CARTESIAN_POINT('Ctrl Pts',(-15.320070396385,37.7607947318286,18.));
#27361=CARTESIAN_POINT('Ctrl Pts',(-15.320874689078,37.6615277218027,0.));
#27362=CARTESIAN_POINT('Ctrl Pts',(-15.320874689078,37.6615277218027,18.));
#27363=CARTESIAN_POINT('Ctrl Pts',(-15.3210406145546,37.562397408596,0.));
#27364=CARTESIAN_POINT('Ctrl Pts',(-15.3210406145546,37.562397408596,18.));
#27365=CARTESIAN_POINT('Ctrl Pts',(-15.3205561366169,37.4634097578665,0.));
#27366=CARTESIAN_POINT('Ctrl Pts',(-15.3205561366169,37.4634097578665,18.));
#27367=CARTESIAN_POINT('Ctrl Pts',(-15.3194106233801,37.3645702997848,0.));
#27368=CARTESIAN_POINT('Ctrl Pts',(-15.3194106233801,37.3645702997848,18.));
#27369=CARTESIAN_POINT('Ctrl Pts',(-15.3175963510697,37.2658836214694,0.));
#27370=CARTESIAN_POINT('Ctrl Pts',(-15.3175963510697,37.2658836214694,18.));
#27371=CARTESIAN_POINT('Ctrl Pts',(-15.3151109648809,37.1673525354642,0.));
#27372=CARTESIAN_POINT('Ctrl Pts',(-15.3151109648809,37.1673525354642,18.));
#27373=CARTESIAN_POINT('Ctrl Pts',(-15.3119562971444,37.0689784837457,0.));
#27374=CARTESIAN_POINT('Ctrl Pts',(-15.3119562971444,37.0689784837457,18.));
#27375=CARTESIAN_POINT('Ctrl Pts',(-15.3081335446406,36.970763176802,0.));
#27376=CARTESIAN_POINT('Ctrl Pts',(-15.3081335446406,36.970763176802,18.));
#27377=CARTESIAN_POINT('Ctrl Pts',(-15.3036390436952,36.8727100302512,0.));
#27378=CARTESIAN_POINT('Ctrl Pts',(-15.3036390436952,36.8727100302512,18.));
#27379=CARTESIAN_POINT('Ctrl Pts',(-15.2984606286737,36.7748254044502,0.));
#27380=CARTESIAN_POINT('Ctrl Pts',(-15.2984606286737,36.7748254044502,18.));
#27381=CARTESIAN_POINT('Ctrl Pts',(-15.2925717100767,36.6771206167756,0.));
#27382=CARTESIAN_POINT('Ctrl Pts',(-15.2925717100767,36.6771206167756,18.));
#27383=CARTESIAN_POINT('Ctrl Pts',(-15.2859343913094,36.5796108931244,0.));
#27384=CARTESIAN_POINT('Ctrl Pts',(-15.2859343913094,36.5796108931244,18.));
#27385=CARTESIAN_POINT('Ctrl Pts',(-15.2785104654792,36.4823116513289,0.));
#27386=CARTESIAN_POINT('Ctrl Pts',(-15.2785104654792,36.4823116513289,18.));
#27387=CARTESIAN_POINT('Ctrl Pts',(-15.2702711460937,36.3852352131887,0.));
#27388=CARTESIAN_POINT('Ctrl Pts',(-15.2702711460937,36.3852352131887,18.));
#27389=CARTESIAN_POINT('Ctrl Pts',(-15.2612053303773,36.2883880151607,0.));
#27390=CARTESIAN_POINT('Ctrl Pts',(-15.2612053303773,36.2883880151607,18.));
#27391=CARTESIAN_POINT('Ctrl Pts',(-15.2513334565427,36.1917659216814,0.));
#27392=CARTESIAN_POINT('Ctrl Pts',(-15.2513334565427,36.1917659216814,18.));
#27393=CARTESIAN_POINT('Ctrl Pts',(-15.240697754828,36.095357546697,0.));
#27394=CARTESIAN_POINT('Ctrl Pts',(-15.240697754828,36.095357546697,18.));
#27395=CARTESIAN_POINT('Ctrl Pts',(-15.2293360946131,35.9991531408727,0.));
#27396=CARTESIAN_POINT('Ctrl Pts',(-15.2293360946131,35.9991531408727,18.));
#27397=CARTESIAN_POINT('Ctrl Pts',(-15.2172585668056,35.9031525499277,0.));
#27398=CARTESIAN_POINT('Ctrl Pts',(-15.2172585668056,35.9031525499277,18.));
#27399=CARTESIAN_POINT('Ctrl Pts',(-15.2044274601769,35.8073720252878,0.));
#27400=CARTESIAN_POINT('Ctrl Pts',(-15.2044274601769,35.8073720252878,18.));
#27401=CARTESIAN_POINT('Ctrl Pts',(-15.1907243629659,35.7118553943773,0.));
#27402=CARTESIAN_POINT('Ctrl Pts',(-15.1907243629659,35.7118553943773,18.));
#27403=CARTESIAN_POINT('Ctrl Pts',(-15.1759785763051,35.6166644736253,0.));
#27404=CARTESIAN_POINT('Ctrl Pts',(-15.1759785763051,35.6166644736253,18.));
#27405=CARTESIAN_POINT('Ctrl Pts',(-15.1600260710384,35.5218591529745,0.));
#27406=CARTESIAN_POINT('Ctrl Pts',(-15.1600260710384,35.5218591529745,18.));
#27407=CARTESIAN_POINT('Ctrl Pts',(-15.1427632633831,35.4274792115856,0.));
#27408=CARTESIAN_POINT('Ctrl Pts',(-15.1427632633831,35.4274792115856,18.));
#27409=CARTESIAN_POINT('Ctrl Pts',(-15.1241934020681,35.3335286891314,0.));
#27410=CARTESIAN_POINT('Ctrl Pts',(-15.1241934020681,35.3335286891314,18.));
#27411=CARTESIAN_POINT('Ctrl Pts',(-15.104500806927,35.2399506932815,0.));
#27412=CARTESIAN_POINT('Ctrl Pts',(-15.104500806927,35.2399506932815,18.));
#27413=CARTESIAN_POINT('Ctrl Pts',(-15.08395927165,35.1466591020976,0.));
#27414=CARTESIAN_POINT('Ctrl Pts',(-15.08395927165,35.1466591020976,18.));
#27415=CARTESIAN_POINT('Ctrl Pts',(-15.0627878528202,35.0535882932913,0.));
#27416=CARTESIAN_POINT('Ctrl Pts',(-15.0627878528202,35.0535882932913,18.));
#27417=CARTESIAN_POINT('Ctrl Pts',(-15.041018569143,34.9607388363587,0.));
#27418=CARTESIAN_POINT('Ctrl Pts',(-15.041018569143,34.9607388363587,18.));
#27419=CARTESIAN_POINT('Ctrl Pts',(-15.0183713484962,34.8682205930809,0.));
#27420=CARTESIAN_POINT('Ctrl Pts',(-15.0183713484962,34.8682205930809,18.));
#27421=CARTESIAN_POINT('Ctrl Pts',(-14.9940927023322,34.7763085406486,0.));
#27422=CARTESIAN_POINT('Ctrl Pts',(-14.9940927023322,34.7763085406486,18.));
#27423=CARTESIAN_POINT('Ctrl Pts',(-14.9671565602316,34.6853717911268,0.));
#27424=CARTESIAN_POINT('Ctrl Pts',(-14.9671565602316,34.6853717911268,18.));
#27425=CARTESIAN_POINT('Ctrl Pts',(-14.9426481276593,34.6137007885254,0.));
#27426=CARTESIAN_POINT('Ctrl Pts',(-14.9426481276593,34.6137007885254,18.));
#27427=CARTESIAN_POINT('Ctrl Pts',(-14.9222326355678,34.5606858566713,0.));
#27428=CARTESIAN_POINT('Ctrl Pts',(-14.9222326355678,34.5606858566713,18.));
#27429=CARTESIAN_POINT('Ctrl Pts',(-14.9076710061311,34.525687510388,0.));
#27430=CARTESIAN_POINT('Ctrl Pts',(-14.9076710061311,34.525687510388,18.));
#27431=CARTESIAN_POINT('Ctrl Pts',(-14.9001523628048,34.5082745737944,0.));
#27432=CARTESIAN_POINT('Ctrl Pts',(-14.9001523628048,34.5082745737944,18.));
#27433=CARTESIAN_POINT('',(-14.9114864958881,41.3962265246839,0.));
#27434=CARTESIAN_POINT('Ctrl Pts',(-14.9001523628048,34.5082745737944,0.));
#27435=CARTESIAN_POINT('Ctrl Pts',(-14.9076710061311,34.525687510388,0.));
#27436=CARTESIAN_POINT('Ctrl Pts',(-14.9222326355678,34.5606858566713,0.));
#27437=CARTESIAN_POINT('Ctrl Pts',(-14.9426481276593,34.6137007885254,0.));
#27438=CARTESIAN_POINT('Ctrl Pts',(-14.9671565602316,34.6853717911268,0.));
#27439=CARTESIAN_POINT('Ctrl Pts',(-14.9940927023322,34.7763085406486,0.));
#27440=CARTESIAN_POINT('Ctrl Pts',(-15.0183713484962,34.8682205930809,0.));
#27441=CARTESIAN_POINT('Ctrl Pts',(-15.041018569143,34.9607388363587,0.));
#27442=CARTESIAN_POINT('Ctrl Pts',(-15.0627878528202,35.0535882932913,0.));
#27443=CARTESIAN_POINT('Ctrl Pts',(-15.08395927165,35.1466591020976,0.));
#27444=CARTESIAN_POINT('Ctrl Pts',(-15.104500806927,35.2399506932815,0.));
#27445=CARTESIAN_POINT('Ctrl Pts',(-15.1241934020681,35.3335286891314,0.));
#27446=CARTESIAN_POINT('Ctrl Pts',(-15.1427632633831,35.4274792115856,0.));
#27447=CARTESIAN_POINT('Ctrl Pts',(-15.1600260710384,35.5218591529745,0.));
#27448=CARTESIAN_POINT('Ctrl Pts',(-15.1759785763051,35.6166644736253,0.));
#27449=CARTESIAN_POINT('Ctrl Pts',(-15.1907243629659,35.7118553943773,0.));
#27450=CARTESIAN_POINT('Ctrl Pts',(-15.2044274601769,35.8073720252878,0.));
#27451=CARTESIAN_POINT('Ctrl Pts',(-15.2172585668056,35.9031525499277,0.));
#27452=CARTESIAN_POINT('Ctrl Pts',(-15.2293360946131,35.9991531408727,0.));
#27453=CARTESIAN_POINT('Ctrl Pts',(-15.240697754828,36.095357546697,0.));
#27454=CARTESIAN_POINT('Ctrl Pts',(-15.2513334565427,36.1917659216814,0.));
#27455=CARTESIAN_POINT('Ctrl Pts',(-15.2612053303773,36.2883880151607,0.));
#27456=CARTESIAN_POINT('Ctrl Pts',(-15.2702711460937,36.3852352131887,0.));
#27457=CARTESIAN_POINT('Ctrl Pts',(-15.2785104654792,36.4823116513289,0.));
#27458=CARTESIAN_POINT('Ctrl Pts',(-15.2859343913094,36.5796108931244,0.));
#27459=CARTESIAN_POINT('Ctrl Pts',(-15.2925717100767,36.6771206167756,0.));
#27460=CARTESIAN_POINT('Ctrl Pts',(-15.2984606286737,36.7748254044502,0.));
#27461=CARTESIAN_POINT('Ctrl Pts',(-15.3036390436952,36.8727100302512,0.));
#27462=CARTESIAN_POINT('Ctrl Pts',(-15.3081335446406,36.970763176802,0.));
#27463=CARTESIAN_POINT('Ctrl Pts',(-15.3119562971444,37.0689784837457,0.));
#27464=CARTESIAN_POINT('Ctrl Pts',(-15.3151109648809,37.1673525354642,0.));
#27465=CARTESIAN_POINT('Ctrl Pts',(-15.3175963510697,37.2658836214694,0.));
#27466=CARTESIAN_POINT('Ctrl Pts',(-15.3194106233801,37.3645702997848,0.));
#27467=CARTESIAN_POINT('Ctrl Pts',(-15.3205561366169,37.4634097578665,0.));
#27468=CARTESIAN_POINT('Ctrl Pts',(-15.3210406145546,37.562397408596,0.));
#27469=CARTESIAN_POINT('Ctrl Pts',(-15.320874689078,37.6615277218027,0.));
#27470=CARTESIAN_POINT('Ctrl Pts',(-15.320070396385,37.7607947318286,0.));
#27471=CARTESIAN_POINT('Ctrl Pts',(-15.3186394335023,37.8601926265378,0.));
#27472=CARTESIAN_POINT('Ctrl Pts',(-15.3165911656268,37.959716421934,0.));
#27473=CARTESIAN_POINT('Ctrl Pts',(-15.3139321941687,38.0593621055415,0.));
#27474=CARTESIAN_POINT('Ctrl Pts',(-15.310667421514,38.1591262705847,0.));
#27475=CARTESIAN_POINT('Ctrl Pts',(-15.3068007250314,38.2590058835965,0.));
#27476=CARTESIAN_POINT('Ctrl Pts',(-15.3023357307483,38.3589980188324,0.));
#27477=CARTESIAN_POINT('Ctrl Pts',(-15.2972767037469,38.4590995527814,0.));
#27478=CARTESIAN_POINT('Ctrl Pts',(-15.2916287700102,38.5593070891769,0.));
#27479=CARTESIAN_POINT('Ctrl Pts',(-15.2853974668211,38.659617115053,0.));
#27480=CARTESIAN_POINT('Ctrl Pts',(-15.2785884727112,38.7600260961351,0.));
#27481=CARTESIAN_POINT('Ctrl Pts',(-15.2712072937639,38.860530586589,0.));
#27482=CARTESIAN_POINT('Ctrl Pts',(-15.2632589109473,38.9611273555758,0.));
#27483=CARTESIAN_POINT('Ctrl Pts',(-15.2547476855825,39.061813415425,0.));
#27484=CARTESIAN_POINT('Ctrl Pts',(-15.2456775636447,39.1625859371304,0.));
#27485=CARTESIAN_POINT('Ctrl Pts',(-15.2360522089072,39.2634421927888,0.));
#27486=CARTESIAN_POINT('Ctrl Pts',(-15.2258751563069,39.3643794927167,0.));
#27487=CARTESIAN_POINT('Ctrl Pts',(-15.2151499908149,39.4653951093947,0.));
#27488=CARTESIAN_POINT('Ctrl Pts',(-15.2038804098649,39.5664862602472,0.));
#27489=CARTESIAN_POINT('Ctrl Pts',(-15.1920701163803,39.6676501731673,0.));
#27490=CARTESIAN_POINT('Ctrl Pts',(-15.1797227547561,39.7688841338802,0.));
#27491=CARTESIAN_POINT('Ctrl Pts',(-15.1668418393198,39.8701855339908,0.));
#27492=CARTESIAN_POINT('Ctrl Pts',(-15.1534306754871,39.9715519332134,0.));
#27493=CARTESIAN_POINT('Ctrl Pts',(-15.1394923361537,40.0729810652204,0.));
#27494=CARTESIAN_POINT('Ctrl Pts',(-15.1250297462408,40.1744707357902,0.));
#27495=CARTESIAN_POINT('Ctrl Pts',(-15.1100457495259,40.2760187401821,0.));
#27496=CARTESIAN_POINT('Ctrl Pts',(-15.0945431800723,40.3776227809037,0.));
#27497=CARTESIAN_POINT('Ctrl Pts',(-15.0785249502524,40.4792803645352,0.));
#27498=CARTESIAN_POINT('Ctrl Pts',(-15.0619940893017,40.58098877043,0.));
#27499=CARTESIAN_POINT('Ctrl Pts',(-15.0449536183143,40.6827452453667,0.));
#27500=CARTESIAN_POINT('Ctrl Pts',(-15.0274064563211,40.7845471608654,0.));
#27501=CARTESIAN_POINT('Ctrl Pts',(-15.0093553188655,40.8863921801,0.));
#27502=CARTESIAN_POINT('Ctrl Pts',(-14.9908026205824,40.9882784321884,0.));
#27503=CARTESIAN_POINT('Ctrl Pts',(-14.9679399407908,41.1105898934098,0.));
#27504=CARTESIAN_POINT('Ctrl Pts',(-14.9482653093396,41.2125650743922,0.));
#27505=CARTESIAN_POINT('Ctrl Pts',(-14.9321285285561,41.2941761025922,0.));
#27506=CARTESIAN_POINT('Ctrl Pts',(-14.919802810928,41.3554017279611,0.));
#27507=CARTESIAN_POINT('Ctrl Pts',(-14.911486495888,41.396226524684,0.));
#27508=CARTESIAN_POINT('',(-14.9114864958881,41.3962265246839,15.));
#27509=CARTESIAN_POINT('Ctrl Pts',(-14.911486495888,41.396226524684,15.));
#27510=CARTESIAN_POINT('Ctrl Pts',(-14.9156446533966,41.3758141263348,15.));
#27511=CARTESIAN_POINT('Ctrl Pts',(-14.9239113834707,41.3349931861715,15.));
#27512=CARTESIAN_POINT('Ctrl Pts',(-14.936162723752,41.2737733455422,15.));
#27513=CARTESIAN_POINT('Ctrl Pts',(-14.9522002356298,41.1921700381957,15.));
#27514=CARTESIAN_POINT('Ctrl Pts',(-14.9717503874227,41.0902046498729,15.));
#27515=CARTESIAN_POINT('Ctrl Pts',(-14.9908026205824,40.9882784321884,15.));
#27516=CARTESIAN_POINT('Ctrl Pts',(-15.0093553188655,40.8863921801,15.));
#27517=CARTESIAN_POINT('Ctrl Pts',(-15.0274064563211,40.7845471608654,15.));
#27518=CARTESIAN_POINT('Ctrl Pts',(-15.0449536183143,40.6827452453667,15.));
#27519=CARTESIAN_POINT('Ctrl Pts',(-15.0619940893017,40.58098877043,15.));
#27520=CARTESIAN_POINT('Ctrl Pts',(-15.0785249502524,40.4792803645352,15.));
#27521=CARTESIAN_POINT('Ctrl Pts',(-15.0945431800723,40.3776227809037,15.));
#27522=CARTESIAN_POINT('Ctrl Pts',(-15.1100457495259,40.2760187401821,15.));
#27523=CARTESIAN_POINT('Ctrl Pts',(-15.1250297462408,40.1744707357902,15.));
#27524=CARTESIAN_POINT('Ctrl Pts',(-15.1394923361537,40.0729810652204,15.));
#27525=CARTESIAN_POINT('Ctrl Pts',(-15.1534306754871,39.9715519332134,15.));
#27526=CARTESIAN_POINT('Ctrl Pts',(-15.1668418393198,39.8701855339908,15.));
#27527=CARTESIAN_POINT('Ctrl Pts',(-15.1797227547561,39.7688841338802,15.));
#27528=CARTESIAN_POINT('Ctrl Pts',(-15.1920701163803,39.6676501731673,15.));
#27529=CARTESIAN_POINT('Ctrl Pts',(-15.2038804098649,39.5664862602472,15.));
#27530=CARTESIAN_POINT('Ctrl Pts',(-15.2151499908149,39.4653951093947,15.));
#27531=CARTESIAN_POINT('Ctrl Pts',(-15.2258751563069,39.3643794927167,15.));
#27532=CARTESIAN_POINT('Ctrl Pts',(-15.2360522089072,39.2634421927888,15.));
#27533=CARTESIAN_POINT('Ctrl Pts',(-15.2456775636447,39.1625859371304,15.));
#27534=CARTESIAN_POINT('Ctrl Pts',(-15.2547476855825,39.061813415425,15.));
#27535=CARTESIAN_POINT('Ctrl Pts',(-15.2632589109473,38.9611273555758,15.));
#27536=CARTESIAN_POINT('Ctrl Pts',(-15.2712072937639,38.860530586589,15.));
#27537=CARTESIAN_POINT('Ctrl Pts',(-15.2785884727112,38.7600260961351,15.));
#27538=CARTESIAN_POINT('Ctrl Pts',(-15.2853974668211,38.659617115053,15.));
#27539=CARTESIAN_POINT('Ctrl Pts',(-15.2916287700102,38.5593070891769,15.));
#27540=CARTESIAN_POINT('Ctrl Pts',(-15.2972767037469,38.4590995527814,15.));
#27541=CARTESIAN_POINT('Ctrl Pts',(-15.3023357307483,38.3589980188324,15.));
#27542=CARTESIAN_POINT('Ctrl Pts',(-15.3068007250314,38.2590058835965,15.));
#27543=CARTESIAN_POINT('Ctrl Pts',(-15.310667421514,38.1591262705847,15.));
#27544=CARTESIAN_POINT('Ctrl Pts',(-15.3139321941687,38.0593621055415,15.));
#27545=CARTESIAN_POINT('Ctrl Pts',(-15.3165911656268,37.959716421934,15.));
#27546=CARTESIAN_POINT('Ctrl Pts',(-15.3186394335023,37.8601926265378,15.));
#27547=CARTESIAN_POINT('Ctrl Pts',(-15.320070396385,37.7607947318286,15.));
#27548=CARTESIAN_POINT('Ctrl Pts',(-15.320874689078,37.6615277218027,15.));
#27549=CARTESIAN_POINT('Ctrl Pts',(-15.3210406145546,37.562397408596,15.));
#27550=CARTESIAN_POINT('Ctrl Pts',(-15.3205561366169,37.4634097578665,15.));
#27551=CARTESIAN_POINT('Ctrl Pts',(-15.3194106233801,37.3645702997848,15.));
#27552=CARTESIAN_POINT('Ctrl Pts',(-15.3175963510697,37.2658836214694,15.));
#27553=CARTESIAN_POINT('Ctrl Pts',(-15.3151109648809,37.1673525354642,15.));
#27554=CARTESIAN_POINT('Ctrl Pts',(-15.3119562971444,37.0689784837457,15.));
#27555=CARTESIAN_POINT('Ctrl Pts',(-15.3081335446406,36.970763176802,15.));
#27556=CARTESIAN_POINT('Ctrl Pts',(-15.3036390436952,36.8727100302512,15.));
#27557=CARTESIAN_POINT('Ctrl Pts',(-15.2984606286737,36.7748254044502,15.));
#27558=CARTESIAN_POINT('Ctrl Pts',(-15.2925717100767,36.6771206167756,15.));
#27559=CARTESIAN_POINT('Ctrl Pts',(-15.2859343913094,36.5796108931244,15.));
#27560=CARTESIAN_POINT('Ctrl Pts',(-15.2785104654792,36.4823116513289,15.));
#27561=CARTESIAN_POINT('Ctrl Pts',(-15.2702711460937,36.3852352131887,15.));
#27562=CARTESIAN_POINT('Ctrl Pts',(-15.2612053303773,36.2883880151607,15.));
#27563=CARTESIAN_POINT('Ctrl Pts',(-15.2513334565427,36.1917659216814,15.));
#27564=CARTESIAN_POINT('Ctrl Pts',(-15.240697754828,36.095357546697,15.));
#27565=CARTESIAN_POINT('Ctrl Pts',(-15.2293360946131,35.9991531408727,15.));
#27566=CARTESIAN_POINT('Ctrl Pts',(-15.2172585668056,35.9031525499277,15.));
#27567=CARTESIAN_POINT('Ctrl Pts',(-15.2044274601769,35.8073720252878,15.));
#27568=CARTESIAN_POINT('Ctrl Pts',(-15.1907243629659,35.7118553943773,15.));
#27569=CARTESIAN_POINT('Ctrl Pts',(-15.1759785763051,35.6166644736253,15.));
#27570=CARTESIAN_POINT('Ctrl Pts',(-15.1600260710384,35.5218591529745,15.));
#27571=CARTESIAN_POINT('Ctrl Pts',(-15.1427632633831,35.4274792115856,15.));
#27572=CARTESIAN_POINT('Ctrl Pts',(-15.1241934020681,35.3335286891314,15.));
#27573=CARTESIAN_POINT('Ctrl Pts',(-15.104500806927,35.2399506932815,15.));
#27574=CARTESIAN_POINT('Ctrl Pts',(-15.08395927165,35.1466591020976,15.));
#27575=CARTESIAN_POINT('Ctrl Pts',(-15.0627878528202,35.0535882932913,15.));
#27576=CARTESIAN_POINT('Ctrl Pts',(-15.041018569143,34.9607388363587,15.));
#27577=CARTESIAN_POINT('Ctrl Pts',(-15.0183713484962,34.8682205930809,15.));
#27578=CARTESIAN_POINT('Ctrl Pts',(-14.9940927023322,34.7763085406486,15.));
#27579=CARTESIAN_POINT('Ctrl Pts',(-14.9671565602316,34.6853717911268,15.));
#27580=CARTESIAN_POINT('Ctrl Pts',(-14.9426481276593,34.6137007885254,15.));
#27581=CARTESIAN_POINT('Ctrl Pts',(-14.9222326355678,34.5606858566713,15.));
#27582=CARTESIAN_POINT('Ctrl Pts',(-14.9076710061311,34.525687510388,15.));
#27583=CARTESIAN_POINT('Ctrl Pts',(-14.9001523628048,34.5082745737944,15.));
#27584=CARTESIAN_POINT('',(-14.9114864958881,41.3962265246839,0.));
#27585=CARTESIAN_POINT('Origin',(-3.50213800024364E-12,1.07784724682657E-11,
0.));
#27586=CARTESIAN_POINT('',(-12.2684454652018,42.2550026135057,0.));
#27587=CARTESIAN_POINT('Origin',(-3.50213800024364E-12,1.07784724682657E-11,
0.));
#27588=CARTESIAN_POINT('',(-12.2684454652018,42.2550026135057,15.));
#27589=CARTESIAN_POINT('Origin',(-3.50213800024364E-12,1.07784724682657E-11,
15.));
#27590=CARTESIAN_POINT('',(-12.2684454652018,42.2550026135057,0.));
#27591=CARTESIAN_POINT('Ctrl Pts',(-8.22897839625061,36.6758703925241,0.));
#27592=CARTESIAN_POINT('Ctrl Pts',(-8.22897839625061,36.6758703925241,18.));
#27593=CARTESIAN_POINT('Ctrl Pts',(-8.23313075335376,36.6943771018148,0.));
#27594=CARTESIAN_POINT('Ctrl Pts',(-8.23313075335376,36.6943771018148,18.));
#27595=CARTESIAN_POINT('Ctrl Pts',(-8.24192165947367,36.7312504697652,0.));
#27596=CARTESIAN_POINT('Ctrl Pts',(-8.24192165947367,36.7312504697652,18.));
#27597=CARTESIAN_POINT('Ctrl Pts',(-8.2565665745182,36.7861403757604,0.));
#27598=CARTESIAN_POINT('Ctrl Pts',(-8.2565665745182,36.7861403757604,18.));
#27599=CARTESIAN_POINT('Ctrl Pts',(-8.27886599440784,36.8585291300917,0.));
#27600=CARTESIAN_POINT('Ctrl Pts',(-8.27886599440784,36.8585291300917,18.));
#27601=CARTESIAN_POINT('Ctrl Pts',(-8.31052547794591,36.9479311729484,0.));
#27602=CARTESIAN_POINT('Ctrl Pts',(-8.31052547794591,36.9479311729484,18.));
#27603=CARTESIAN_POINT('Ctrl Pts',(-8.34490818952639,37.0365602155148,0.));
#27604=CARTESIAN_POINT('Ctrl Pts',(-8.34490818952639,37.0365602155148,18.));
#27605=CARTESIAN_POINT('Ctrl Pts',(-8.38096706211447,37.1247207489179,0.));
#27606=CARTESIAN_POINT('Ctrl Pts',(-8.38096706211447,37.1247207489179,18.));
#27607=CARTESIAN_POINT('Ctrl Pts',(-8.4179308831326,37.2126332013933,0.));
#27608=CARTESIAN_POINT('Ctrl Pts',(-8.4179308831326,37.2126332013933,18.));
#27609=CARTESIAN_POINT('Ctrl Pts',(-8.45550849433959,37.3003733151561,0.));
#27610=CARTESIAN_POINT('Ctrl Pts',(-8.45550849433959,37.3003733151561,18.));
#27611=CARTESIAN_POINT('Ctrl Pts',(-8.49372546467075,37.3879218093514,0.));
#27612=CARTESIAN_POINT('Ctrl Pts',(-8.49372546467075,37.3879218093514,18.));
#27613=CARTESIAN_POINT('Ctrl Pts',(-8.53279758643784,37.4752030152968,0.));
#27614=CARTESIAN_POINT('Ctrl Pts',(-8.53279758643784,37.4752030152968,18.));
#27615=CARTESIAN_POINT('Ctrl Pts',(-8.57299698459465,37.5621256752108,0.));
#27616=CARTESIAN_POINT('Ctrl Pts',(-8.57299698459465,37.5621256752108,18.));
#27617=CARTESIAN_POINT('Ctrl Pts',(-8.61450621749155,37.6486274754754,0.));
#27618=CARTESIAN_POINT('Ctrl Pts',(-8.61450621749155,37.6486274754754,18.));
#27619=CARTESIAN_POINT('Ctrl Pts',(-8.65732553894524,37.7347032383719,0.));
#27620=CARTESIAN_POINT('Ctrl Pts',(-8.65732553894524,37.7347032383719,18.));
#27621=CARTESIAN_POINT('Ctrl Pts',(-8.70134776631143,37.8203816669031,0.));
#27622=CARTESIAN_POINT('Ctrl Pts',(-8.70134776631143,37.8203816669031,18.));
#27623=CARTESIAN_POINT('Ctrl Pts',(-8.74640499479002,37.9057107230066,0.));
#27624=CARTESIAN_POINT('Ctrl Pts',(-8.74640499479002,37.9057107230066,18.));
#27625=CARTESIAN_POINT('Ctrl Pts',(-8.79232279131092,37.9907407304174,0.));
#27626=CARTESIAN_POINT('Ctrl Pts',(-8.79232279131092,37.9907407304174,18.));
#27627=CARTESIAN_POINT('Ctrl Pts',(-8.83897959763348,38.0755058326913,0.));
#27628=CARTESIAN_POINT('Ctrl Pts',(-8.83897959763348,38.0755058326913,18.));
#27629=CARTESIAN_POINT('Ctrl Pts',(-8.88633535238434,38.1600150482528,0.));
#27630=CARTESIAN_POINT('Ctrl Pts',(-8.88633535238434,38.1600150482528,18.));
#27631=CARTESIAN_POINT('Ctrl Pts',(-8.93439830996339,38.2442625706309,0.));
#27632=CARTESIAN_POINT('Ctrl Pts',(-8.93439830996339,38.2442625706309,18.));
#27633=CARTESIAN_POINT('Ctrl Pts',(-8.98320483785759,38.3282340281403,0.));
#27634=CARTESIAN_POINT('Ctrl Pts',(-8.98320483785759,38.3282340281403,18.));
#27635=CARTESIAN_POINT('Ctrl Pts',(-9.0327957936019,38.4119138099805,0.));
#27636=CARTESIAN_POINT('Ctrl Pts',(-9.0327957936019,38.4119138099805,18.));
#27637=CARTESIAN_POINT('Ctrl Pts',(-9.08319014288085,38.4952932486131,0.));
#27638=CARTESIAN_POINT('Ctrl Pts',(-9.08319014288085,38.4952932486131,18.));
#27639=CARTESIAN_POINT('Ctrl Pts',(-9.13437512010585,38.5783736628826,0.));
#27640=CARTESIAN_POINT('Ctrl Pts',(-9.13437512010585,38.5783736628826,18.));
#27641=CARTESIAN_POINT('Ctrl Pts',(-9.18632019394329,38.6611620045193,0.));
#27642=CARTESIAN_POINT('Ctrl Pts',(-9.18632019394329,38.6611620045193,18.));
#27643=CARTESIAN_POINT('Ctrl Pts',(-9.23898539199331,38.7436682576832,0.));
#27644=CARTESIAN_POINT('Ctrl Pts',(-9.23898539199331,38.7436682576832,18.));
#27645=CARTESIAN_POINT('Ctrl Pts',(-9.29233110570902,38.8259023794241,0.));
#27646=CARTESIAN_POINT('Ctrl Pts',(-9.29233110570902,38.8259023794241,18.));
#27647=CARTESIAN_POINT('Ctrl Pts',(-9.34632917154636,38.9078708427078,0.));
#27648=CARTESIAN_POINT('Ctrl Pts',(-9.34632917154636,38.9078708427078,18.));
#27649=CARTESIAN_POINT('Ctrl Pts',(-9.40096600877643,38.9895756526779,0.));
#27650=CARTESIAN_POINT('Ctrl Pts',(-9.40096600877643,38.9895756526779,18.));
#27651=CARTESIAN_POINT('Ctrl Pts',(-9.45623664577431,39.0710161994951,0.));
#27652=CARTESIAN_POINT('Ctrl Pts',(-9.45623664577431,39.0710161994951,18.));
#27653=CARTESIAN_POINT('Ctrl Pts',(-9.5121410453562,39.1521903958955,0.));
#27654=CARTESIAN_POINT('Ctrl Pts',(-9.5121410453562,39.1521903958955,18.));
#27655=CARTESIAN_POINT('Ctrl Pts',(-9.56867984233622,39.2330959982788,0.));
#27656=CARTESIAN_POINT('Ctrl Pts',(-9.56867984233622,39.2330959982788,18.));
#27657=CARTESIAN_POINT('Ctrl Pts',(-9.62584947846543,39.3137321153686,0.));
#27658=CARTESIAN_POINT('Ctrl Pts',(-9.62584947846543,39.3137321153686,18.));
#27659=CARTESIAN_POINT('Ctrl Pts',(-9.68364100883826,39.3940995760289,0.));
#27660=CARTESIAN_POINT('Ctrl Pts',(-9.68364100883826,39.3940995760289,18.));
#27661=CARTESIAN_POINT('Ctrl Pts',(-9.74204258152663,39.4742001555227,0.));
#27662=CARTESIAN_POINT('Ctrl Pts',(-9.74204258152663,39.4742001555227,18.));
#27663=CARTESIAN_POINT('Ctrl Pts',(-9.80104095251613,39.5540361022309,0.));
#27664=CARTESIAN_POINT('Ctrl Pts',(-9.80104095251613,39.5540361022309,18.));
#27665=CARTESIAN_POINT('Ctrl Pts',(-9.86062324242559,39.6336095893767,0.));
#27666=CARTESIAN_POINT('Ctrl Pts',(-9.86062324242559,39.6336095893767,18.));
#27667=CARTESIAN_POINT('Ctrl Pts',(-9.92077894513191,39.712922089547,0.));
#27668=CARTESIAN_POINT('Ctrl Pts',(-9.92077894513191,39.712922089547,18.));
#27669=CARTESIAN_POINT('Ctrl Pts',(-9.98150036150822,39.7919742367922,0.));
#27670=CARTESIAN_POINT('Ctrl Pts',(-9.98150036150822,39.7919742367922,18.));
#27671=CARTESIAN_POINT('Ctrl Pts',(-10.0427815229883,39.8707661565233,0.));
#27672=CARTESIAN_POINT('Ctrl Pts',(-10.0427815229883,39.8707661565233,18.));
#27673=CARTESIAN_POINT('Ctrl Pts',(-10.1046175096878,39.9492976736738,0.));
#27674=CARTESIAN_POINT('Ctrl Pts',(-10.1046175096878,39.9492976736738,18.));
#27675=CARTESIAN_POINT('Ctrl Pts',(-10.1670036683795,40.0275685525923,0.));
#27676=CARTESIAN_POINT('Ctrl Pts',(-10.1670036683795,40.0275685525923,18.));
#27677=CARTESIAN_POINT('Ctrl Pts',(-10.2299347125857,40.1055787732578,0.));
#27678=CARTESIAN_POINT('Ctrl Pts',(-10.2299347125857,40.1055787732578,18.));
#27679=CARTESIAN_POINT('Ctrl Pts',(-10.2934044990237,40.1833286010098,0.));
#27680=CARTESIAN_POINT('Ctrl Pts',(-10.2934044990237,40.1833286010098,18.));
#27681=CARTESIAN_POINT('Ctrl Pts',(-10.3574064830678,40.2608184485326,0.));
#27682=CARTESIAN_POINT('Ctrl Pts',(-10.3574064830678,40.2608184485326,18.));
#27683=CARTESIAN_POINT('Ctrl Pts',(-10.421933993295,40.3380487942952,0.));
#27684=CARTESIAN_POINT('Ctrl Pts',(-10.421933993295,40.3380487942952,18.));
#27685=CARTESIAN_POINT('Ctrl Pts',(-10.48698054978,40.4150200869536,0.));
#27686=CARTESIAN_POINT('Ctrl Pts',(-10.48698054978,40.4150200869536,18.));
#27687=CARTESIAN_POINT('Ctrl Pts',(-10.5525402237951,40.4917326404439,0.));
#27688=CARTESIAN_POINT('Ctrl Pts',(-10.5525402237951,40.4917326404439,18.));
#27689=CARTESIAN_POINT('Ctrl Pts',(-10.618607730849,40.5681866012103,0.));
#27690=CARTESIAN_POINT('Ctrl Pts',(-10.618607730849,40.5681866012103,18.));
#27691=CARTESIAN_POINT('Ctrl Pts',(-10.6851782157325,40.6443819999244,0.));
#27692=CARTESIAN_POINT('Ctrl Pts',(-10.6851782157325,40.6443819999244,18.));
#27693=CARTESIAN_POINT('Ctrl Pts',(-10.7522471109694,40.7203187831783,0.));
#27694=CARTESIAN_POINT('Ctrl Pts',(-10.7522471109694,40.7203187831783,18.));
#27695=CARTESIAN_POINT('Ctrl Pts',(-10.8198099757795,40.795996852756,0.));
#27696=CARTESIAN_POINT('Ctrl Pts',(-10.8198099757795,40.795996852756,18.));
#27697=CARTESIAN_POINT('Ctrl Pts',(-10.8878623066646,40.8714161092412,0.));
#27698=CARTESIAN_POINT('Ctrl Pts',(-10.8878623066646,40.8714161092412,18.));
#27699=CARTESIAN_POINT('Ctrl Pts',(-10.956399476781,40.9465764747798,0.));
#27700=CARTESIAN_POINT('Ctrl Pts',(-10.956399476781,40.9465764747798,18.));
#27701=CARTESIAN_POINT('Ctrl Pts',(-11.0254168609972,41.0214778832142,0.));
#27702=CARTESIAN_POINT('Ctrl Pts',(-11.0254168609972,41.0214778832142,18.));
#27703=CARTESIAN_POINT('Ctrl Pts',(-11.0949099155251,41.0961202807715,0.));
#27704=CARTESIAN_POINT('Ctrl Pts',(-11.0949099155251,41.0961202807715,18.));
#27705=CARTESIAN_POINT('Ctrl Pts',(-11.1648742640378,41.1705036228854,0.));
#27706=CARTESIAN_POINT('Ctrl Pts',(-11.1648742640378,41.1705036228854,18.));
#27707=CARTESIAN_POINT('Ctrl Pts',(-11.2353057980338,41.2446278781981,0.));
#27708=CARTESIAN_POINT('Ctrl Pts',(-11.2353057980338,41.2446278781981,18.));
#27709=CARTESIAN_POINT('Ctrl Pts',(-11.3062006993745,41.3184930194148,0.));
#27710=CARTESIAN_POINT('Ctrl Pts',(-11.3062006993745,41.3184930194148,18.));
#27711=CARTESIAN_POINT('Ctrl Pts',(-11.3775553120176,41.3920989905986,0.));
#27712=CARTESIAN_POINT('Ctrl Pts',(-11.3775553120176,41.3920989905986,18.));
#27713=CARTESIAN_POINT('Ctrl Pts',(-11.4493660393849,41.4654456796071,0.));
#27714=CARTESIAN_POINT('Ctrl Pts',(-11.4493660393849,41.4654456796071,18.));
#27715=CARTESIAN_POINT('Ctrl Pts',(-11.5216292382388,41.5385328935506,0.));
#27716=CARTESIAN_POINT('Ctrl Pts',(-11.5216292382388,41.5385328935506,18.));
#27717=CARTESIAN_POINT('Ctrl Pts',(-11.5943410868252,41.6113603270596,0.));
#27718=CARTESIAN_POINT('Ctrl Pts',(-11.5943410868252,41.6113603270596,18.));
#27719=CARTESIAN_POINT('Ctrl Pts',(-11.6674975352851,41.6839275596248,0.));
#27720=CARTESIAN_POINT('Ctrl Pts',(-11.6674975352851,41.6839275596248,18.));
#27721=CARTESIAN_POINT('Ctrl Pts',(-11.7410945211992,41.7562341395977,0.));
#27722=CARTESIAN_POINT('Ctrl Pts',(-11.7410945211992,41.7562341395977,18.));
#27723=CARTESIAN_POINT('Ctrl Pts',(-11.81512813804,41.8282796562569,0.));
#27724=CARTESIAN_POINT('Ctrl Pts',(-11.81512813804,41.8282796562569,18.));
#27725=CARTESIAN_POINT('Ctrl Pts',(-11.8895948153349,41.9000638152266,0.));
#27726=CARTESIAN_POINT('Ctrl Pts',(-11.8895948153349,41.9000638152266,18.));
#27727=CARTESIAN_POINT('Ctrl Pts',(-11.9644914999263,41.9715865222182,0.));
#27728=CARTESIAN_POINT('Ctrl Pts',(-11.9644914999263,41.9715865222182,18.));
#27729=CARTESIAN_POINT('Ctrl Pts',(-12.0398158079102,42.0428479428228,0.));
#27730=CARTESIAN_POINT('Ctrl Pts',(-12.0398158079102,42.0428479428228,18.));
#27731=CARTESIAN_POINT('Ctrl Pts',(-12.1155659644537,42.1138483839101,0.));
#27732=CARTESIAN_POINT('Ctrl Pts',(-12.1155659644537,42.1138483839101,18.));
#27733=CARTESIAN_POINT('Ctrl Pts',(-12.1765058047069,42.1704402333854,0.));
#27734=CARTESIAN_POINT('Ctrl Pts',(-12.1765058047069,42.1704402333854,18.));
#27735=CARTESIAN_POINT('Ctrl Pts',(-12.2224014666679,42.2127669677092,0.));
#27736=CARTESIAN_POINT('Ctrl Pts',(-12.2224014666679,42.2127669677092,18.));
#27737=CARTESIAN_POINT('Ctrl Pts',(-12.2530833383985,42.2409327400055,0.));
#27738=CARTESIAN_POINT('Ctrl Pts',(-12.2530833383985,42.2409327400055,18.));
#27739=CARTESIAN_POINT('Ctrl Pts',(-12.2684454652018,42.2550026135057,0.));
#27740=CARTESIAN_POINT('Ctrl Pts',(-12.2684454652018,42.2550026135057,18.));
#27741=CARTESIAN_POINT('Ctrl Pts',(-8.22897839625061,36.6758703925241,0.));
#27742=CARTESIAN_POINT('Ctrl Pts',(-8.23313075335376,36.6943771018148,0.));
#27743=CARTESIAN_POINT('Ctrl Pts',(-8.24192165947367,36.7312504697652,0.));
#27744=CARTESIAN_POINT('Ctrl Pts',(-8.2565665745182,36.7861403757604,0.));
#27745=CARTESIAN_POINT('Ctrl Pts',(-8.27886599440784,36.8585291300917,0.));
#27746=CARTESIAN_POINT('Ctrl Pts',(-8.31052547794591,36.9479311729484,0.));
#27747=CARTESIAN_POINT('Ctrl Pts',(-8.34490818952639,37.0365602155148,0.));
#27748=CARTESIAN_POINT('Ctrl Pts',(-8.38096706211447,37.1247207489179,0.));
#27749=CARTESIAN_POINT('Ctrl Pts',(-8.4179308831326,37.2126332013933,0.));
#27750=CARTESIAN_POINT('Ctrl Pts',(-8.45550849433959,37.3003733151561,0.));
#27751=CARTESIAN_POINT('Ctrl Pts',(-8.49372546467075,37.3879218093514,0.));
#27752=CARTESIAN_POINT('Ctrl Pts',(-8.53279758643784,37.4752030152968,0.));
#27753=CARTESIAN_POINT('Ctrl Pts',(-8.57299698459465,37.5621256752108,0.));
#27754=CARTESIAN_POINT('Ctrl Pts',(-8.61450621749155,37.6486274754754,0.));
#27755=CARTESIAN_POINT('Ctrl Pts',(-8.65732553894524,37.7347032383719,0.));
#27756=CARTESIAN_POINT('Ctrl Pts',(-8.70134776631143,37.8203816669031,0.));
#27757=CARTESIAN_POINT('Ctrl Pts',(-8.74640499479002,37.9057107230066,0.));
#27758=CARTESIAN_POINT('Ctrl Pts',(-8.79232279131092,37.9907407304174,0.));
#27759=CARTESIAN_POINT('Ctrl Pts',(-8.83897959763348,38.0755058326913,0.));
#27760=CARTESIAN_POINT('Ctrl Pts',(-8.88633535238434,38.1600150482528,0.));
#27761=CARTESIAN_POINT('Ctrl Pts',(-8.93439830996339,38.2442625706309,0.));
#27762=CARTESIAN_POINT('Ctrl Pts',(-8.98320483785759,38.3282340281403,0.));
#27763=CARTESIAN_POINT('Ctrl Pts',(-9.0327957936019,38.4119138099805,0.));
#27764=CARTESIAN_POINT('Ctrl Pts',(-9.08319014288085,38.4952932486131,0.));
#27765=CARTESIAN_POINT('Ctrl Pts',(-9.13437512010585,38.5783736628826,0.));
#27766=CARTESIAN_POINT('Ctrl Pts',(-9.18632019394329,38.6611620045193,0.));
#27767=CARTESIAN_POINT('Ctrl Pts',(-9.23898539199331,38.7436682576832,0.));
#27768=CARTESIAN_POINT('Ctrl Pts',(-9.29233110570902,38.8259023794241,0.));
#27769=CARTESIAN_POINT('Ctrl Pts',(-9.34632917154636,38.9078708427078,0.));
#27770=CARTESIAN_POINT('Ctrl Pts',(-9.40096600877643,38.9895756526779,0.));
#27771=CARTESIAN_POINT('Ctrl Pts',(-9.45623664577431,39.0710161994951,0.));
#27772=CARTESIAN_POINT('Ctrl Pts',(-9.5121410453562,39.1521903958955,0.));
#27773=CARTESIAN_POINT('Ctrl Pts',(-9.56867984233622,39.2330959982788,0.));
#27774=CARTESIAN_POINT('Ctrl Pts',(-9.62584947846543,39.3137321153686,0.));
#27775=CARTESIAN_POINT('Ctrl Pts',(-9.68364100883826,39.3940995760289,0.));
#27776=CARTESIAN_POINT('Ctrl Pts',(-9.74204258152663,39.4742001555227,0.));
#27777=CARTESIAN_POINT('Ctrl Pts',(-9.80104095251613,39.5540361022309,0.));
#27778=CARTESIAN_POINT('Ctrl Pts',(-9.86062324242559,39.6336095893767,0.));
#27779=CARTESIAN_POINT('Ctrl Pts',(-9.92077894513191,39.712922089547,0.));
#27780=CARTESIAN_POINT('Ctrl Pts',(-9.98150036150822,39.7919742367922,0.));
#27781=CARTESIAN_POINT('Ctrl Pts',(-10.0427815229883,39.8707661565233,0.));
#27782=CARTESIAN_POINT('Ctrl Pts',(-10.1046175096878,39.9492976736738,0.));
#27783=CARTESIAN_POINT('Ctrl Pts',(-10.1670036683795,40.0275685525923,0.));
#27784=CARTESIAN_POINT('Ctrl Pts',(-10.2299347125857,40.1055787732578,0.));
#27785=CARTESIAN_POINT('Ctrl Pts',(-10.2934044990237,40.1833286010098,0.));
#27786=CARTESIAN_POINT('Ctrl Pts',(-10.3574064830678,40.2608184485326,0.));
#27787=CARTESIAN_POINT('Ctrl Pts',(-10.421933993295,40.3380487942952,0.));
#27788=CARTESIAN_POINT('Ctrl Pts',(-10.48698054978,40.4150200869536,0.));
#27789=CARTESIAN_POINT('Ctrl Pts',(-10.5525402237951,40.4917326404439,0.));
#27790=CARTESIAN_POINT('Ctrl Pts',(-10.618607730849,40.5681866012103,0.));
#27791=CARTESIAN_POINT('Ctrl Pts',(-10.6851782157325,40.6443819999244,0.));
#27792=CARTESIAN_POINT('Ctrl Pts',(-10.7522471109694,40.7203187831783,0.));
#27793=CARTESIAN_POINT('Ctrl Pts',(-10.8198099757795,40.795996852756,0.));
#27794=CARTESIAN_POINT('Ctrl Pts',(-10.8878623066646,40.8714161092412,0.));
#27795=CARTESIAN_POINT('Ctrl Pts',(-10.956399476781,40.9465764747798,0.));
#27796=CARTESIAN_POINT('Ctrl Pts',(-11.0254168609972,41.0214778832142,0.));
#27797=CARTESIAN_POINT('Ctrl Pts',(-11.0949099155251,41.0961202807715,0.));
#27798=CARTESIAN_POINT('Ctrl Pts',(-11.1648742640378,41.1705036228854,0.));
#27799=CARTESIAN_POINT('Ctrl Pts',(-11.2353057980338,41.2446278781981,0.));
#27800=CARTESIAN_POINT('Ctrl Pts',(-11.3062006993745,41.3184930194148,0.));
#27801=CARTESIAN_POINT('Ctrl Pts',(-11.3775553120176,41.3920989905986,0.));
#27802=CARTESIAN_POINT('Ctrl Pts',(-11.4493660393849,41.4654456796071,0.));
#27803=CARTESIAN_POINT('Ctrl Pts',(-11.5216292382388,41.5385328935506,0.));
#27804=CARTESIAN_POINT('Ctrl Pts',(-11.5943410868252,41.6113603270596,0.));
#27805=CARTESIAN_POINT('Ctrl Pts',(-11.6674975352851,41.6839275596248,0.));
#27806=CARTESIAN_POINT('Ctrl Pts',(-11.7410945211992,41.7562341395977,0.));
#27807=CARTESIAN_POINT('Ctrl Pts',(-11.81512813804,41.8282796562569,0.));
#27808=CARTESIAN_POINT('Ctrl Pts',(-11.8895948153349,41.9000638152266,0.));
#27809=CARTESIAN_POINT('Ctrl Pts',(-11.9644914999263,41.9715865222182,0.));
#27810=CARTESIAN_POINT('Ctrl Pts',(-12.054880669507,42.0571002269437,0.));
#27811=CARTESIAN_POINT('Ctrl Pts',(-12.1307372881904,42.1280354231517,0.));
#27812=CARTESIAN_POINT('Ctrl Pts',(-12.1917619768791,42.18457517013,0.));
#27813=CARTESIAN_POINT('Ctrl Pts',(-12.2377212115623,42.2268628664988,0.));
#27814=CARTESIAN_POINT('Ctrl Pts',(-12.2684454652018,42.2550026135057,0.));
#27815=CARTESIAN_POINT('Ctrl Pts',(-8.22897839625061,36.6758703925241,15.));
#27816=CARTESIAN_POINT('Ctrl Pts',(-8.23313075335376,36.6943771018148,15.));
#27817=CARTESIAN_POINT('Ctrl Pts',(-8.24192165947367,36.7312504697652,15.));
#27818=CARTESIAN_POINT('Ctrl Pts',(-8.2565665745182,36.7861403757604,15.));
#27819=CARTESIAN_POINT('Ctrl Pts',(-8.27886599440784,36.8585291300917,15.));
#27820=CARTESIAN_POINT('Ctrl Pts',(-8.31052547794591,36.9479311729484,15.));
#27821=CARTESIAN_POINT('Ctrl Pts',(-8.34490818952639,37.0365602155148,15.));
#27822=CARTESIAN_POINT('Ctrl Pts',(-8.38096706211447,37.1247207489179,15.));
#27823=CARTESIAN_POINT('Ctrl Pts',(-8.4179308831326,37.2126332013933,15.));
#27824=CARTESIAN_POINT('Ctrl Pts',(-8.45550849433959,37.3003733151561,15.));
#27825=CARTESIAN_POINT('Ctrl Pts',(-8.49372546467075,37.3879218093514,15.));
#27826=CARTESIAN_POINT('Ctrl Pts',(-8.53279758643784,37.4752030152968,15.));
#27827=CARTESIAN_POINT('Ctrl Pts',(-8.57299698459465,37.5621256752108,15.));
#27828=CARTESIAN_POINT('Ctrl Pts',(-8.61450621749155,37.6486274754754,15.));
#27829=CARTESIAN_POINT('Ctrl Pts',(-8.65732553894524,37.7347032383719,15.));
#27830=CARTESIAN_POINT('Ctrl Pts',(-8.70134776631143,37.8203816669031,15.));
#27831=CARTESIAN_POINT('Ctrl Pts',(-8.74640499479002,37.9057107230066,15.));
#27832=CARTESIAN_POINT('Ctrl Pts',(-8.79232279131092,37.9907407304174,15.));
#27833=CARTESIAN_POINT('Ctrl Pts',(-8.83897959763348,38.0755058326913,15.));
#27834=CARTESIAN_POINT('Ctrl Pts',(-8.88633535238434,38.1600150482528,15.));
#27835=CARTESIAN_POINT('Ctrl Pts',(-8.93439830996339,38.2442625706309,15.));
#27836=CARTESIAN_POINT('Ctrl Pts',(-8.98320483785759,38.3282340281403,15.));
#27837=CARTESIAN_POINT('Ctrl Pts',(-9.0327957936019,38.4119138099805,15.));
#27838=CARTESIAN_POINT('Ctrl Pts',(-9.08319014288085,38.4952932486131,15.));
#27839=CARTESIAN_POINT('Ctrl Pts',(-9.13437512010585,38.5783736628826,15.));
#27840=CARTESIAN_POINT('Ctrl Pts',(-9.18632019394329,38.6611620045193,15.));
#27841=CARTESIAN_POINT('Ctrl Pts',(-9.23898539199331,38.7436682576832,15.));
#27842=CARTESIAN_POINT('Ctrl Pts',(-9.29233110570902,38.8259023794241,15.));
#27843=CARTESIAN_POINT('Ctrl Pts',(-9.34632917154636,38.9078708427078,15.));
#27844=CARTESIAN_POINT('Ctrl Pts',(-9.40096600877643,38.9895756526779,15.));
#27845=CARTESIAN_POINT('Ctrl Pts',(-9.45623664577431,39.0710161994951,15.));
#27846=CARTESIAN_POINT('Ctrl Pts',(-9.5121410453562,39.1521903958955,15.));
#27847=CARTESIAN_POINT('Ctrl Pts',(-9.56867984233622,39.2330959982788,15.));
#27848=CARTESIAN_POINT('Ctrl Pts',(-9.62584947846543,39.3137321153686,15.));
#27849=CARTESIAN_POINT('Ctrl Pts',(-9.68364100883826,39.3940995760289,15.));
#27850=CARTESIAN_POINT('Ctrl Pts',(-9.74204258152663,39.4742001555227,15.));
#27851=CARTESIAN_POINT('Ctrl Pts',(-9.80104095251613,39.5540361022309,15.));
#27852=CARTESIAN_POINT('Ctrl Pts',(-9.86062324242559,39.6336095893767,15.));
#27853=CARTESIAN_POINT('Ctrl Pts',(-9.92077894513191,39.712922089547,15.));
#27854=CARTESIAN_POINT('Ctrl Pts',(-9.98150036150822,39.7919742367922,15.));
#27855=CARTESIAN_POINT('Ctrl Pts',(-10.0427815229883,39.8707661565233,15.));
#27856=CARTESIAN_POINT('Ctrl Pts',(-10.1046175096878,39.9492976736738,15.));
#27857=CARTESIAN_POINT('Ctrl Pts',(-10.1670036683795,40.0275685525923,15.));
#27858=CARTESIAN_POINT('Ctrl Pts',(-10.2299347125857,40.1055787732578,15.));
#27859=CARTESIAN_POINT('Ctrl Pts',(-10.2934044990237,40.1833286010098,15.));
#27860=CARTESIAN_POINT('Ctrl Pts',(-10.3574064830678,40.2608184485326,15.));
#27861=CARTESIAN_POINT('Ctrl Pts',(-10.421933993295,40.3380487942952,15.));
#27862=CARTESIAN_POINT('Ctrl Pts',(-10.48698054978,40.4150200869536,15.));
#27863=CARTESIAN_POINT('Ctrl Pts',(-10.5525402237951,40.4917326404439,15.));
#27864=CARTESIAN_POINT('Ctrl Pts',(-10.618607730849,40.5681866012103,15.));
#27865=CARTESIAN_POINT('Ctrl Pts',(-10.6851782157325,40.6443819999244,15.));
#27866=CARTESIAN_POINT('Ctrl Pts',(-10.7522471109694,40.7203187831783,15.));
#27867=CARTESIAN_POINT('Ctrl Pts',(-10.8198099757795,40.795996852756,15.));
#27868=CARTESIAN_POINT('Ctrl Pts',(-10.8878623066646,40.8714161092412,15.));
#27869=CARTESIAN_POINT('Ctrl Pts',(-10.956399476781,40.9465764747798,15.));
#27870=CARTESIAN_POINT('Ctrl Pts',(-11.0254168609972,41.0214778832142,15.));
#27871=CARTESIAN_POINT('Ctrl Pts',(-11.0949099155251,41.0961202807715,15.));
#27872=CARTESIAN_POINT('Ctrl Pts',(-11.1648742640378,41.1705036228854,15.));
#27873=CARTESIAN_POINT('Ctrl Pts',(-11.2353057980338,41.2446278781981,15.));
#27874=CARTESIAN_POINT('Ctrl Pts',(-11.3062006993745,41.3184930194148,15.));
#27875=CARTESIAN_POINT('Ctrl Pts',(-11.3775553120176,41.3920989905986,15.));
#27876=CARTESIAN_POINT('Ctrl Pts',(-11.4493660393849,41.4654456796071,15.));
#27877=CARTESIAN_POINT('Ctrl Pts',(-11.5216292382388,41.5385328935506,15.));
#27878=CARTESIAN_POINT('Ctrl Pts',(-11.5943410868252,41.6113603270596,15.));
#27879=CARTESIAN_POINT('Ctrl Pts',(-11.6674975352851,41.6839275596248,15.));
#27880=CARTESIAN_POINT('Ctrl Pts',(-11.7410945211992,41.7562341395977,15.));
#27881=CARTESIAN_POINT('Ctrl Pts',(-11.81512813804,41.8282796562569,15.));
#27882=CARTESIAN_POINT('Ctrl Pts',(-11.8895948153349,41.9000638152266,15.));
#27883=CARTESIAN_POINT('Ctrl Pts',(-11.9644914999263,41.9715865222182,15.));
#27884=CARTESIAN_POINT('Ctrl Pts',(-12.054880669507,42.0571002269437,15.));
#27885=CARTESIAN_POINT('Ctrl Pts',(-12.1307372881904,42.1280354231517,15.));
#27886=CARTESIAN_POINT('Ctrl Pts',(-12.1917619768791,42.18457517013,15.));
#27887=CARTESIAN_POINT('Ctrl Pts',(-12.2377212115623,42.2268628664988,15.));
#27888=CARTESIAN_POINT('Ctrl Pts',(-12.2684454652018,42.2550026135057,15.));
#27889=CARTESIAN_POINT('Ctrl Pts',(-1.38952890043916,43.9780537249529,0.));
#27890=CARTESIAN_POINT('Ctrl Pts',(-1.38952890043916,43.9780537249529,18.));
#27891=CARTESIAN_POINT('Ctrl Pts',(-1.39979132121931,43.9599253218252,0.));
#27892=CARTESIAN_POINT('Ctrl Pts',(-1.39979132121931,43.9599253218252,18.));
#27893=CARTESIAN_POINT('Ctrl Pts',(-1.42026781296156,43.9236568607623,0.));
#27894=CARTESIAN_POINT('Ctrl Pts',(-1.42026781296156,43.9236568607623,18.));
#27895=CARTESIAN_POINT('Ctrl Pts',(-1.45083750111682,43.8692192047561,0.));
#27896=CARTESIAN_POINT('Ctrl Pts',(-1.45083750111682,43.8692192047561,18.));
#27897=CARTESIAN_POINT('Ctrl Pts',(-1.49130689006066,43.7965657112708,0.));
#27898=CARTESIAN_POINT('Ctrl Pts',(-1.49130689006066,43.7965657112708,18.));
#27899=CARTESIAN_POINT('Ctrl Pts',(-1.54140922714765,43.7056321934163,0.));
#27900=CARTESIAN_POINT('Ctrl Pts',(-1.54140922714765,43.7056321934163,18.));
#27901=CARTESIAN_POINT('Ctrl Pts',(-1.59102591108103,43.6145820637333,0.));
#27902=CARTESIAN_POINT('Ctrl Pts',(-1.59102591108103,43.6145820637333,18.));
#27903=CARTESIAN_POINT('Ctrl Pts',(-1.64015515906648,43.5234155788248,0.));
#27904=CARTESIAN_POINT('Ctrl Pts',(-1.64015515906648,43.5234155788248,18.));
#27905=CARTESIAN_POINT('Ctrl Pts',(-1.68879465270608,43.4321333178711,0.));
#27906=CARTESIAN_POINT('Ctrl Pts',(-1.68879465270608,43.4321333178711,18.));
#27907=CARTESIAN_POINT('Ctrl Pts',(-1.73694151741124,43.3407363140236,0.));
#27908=CARTESIAN_POINT('Ctrl Pts',(-1.73694151741124,43.3407363140236,18.));
#27909=CARTESIAN_POINT('Ctrl Pts',(-1.78459244842769,43.2492259505872,0.));
#27910=CARTESIAN_POINT('Ctrl Pts',(-1.78459244842769,43.2492259505872,18.));
#27911=CARTESIAN_POINT('Ctrl Pts',(-1.83174385734711,43.1576038253643,0.));
#27912=CARTESIAN_POINT('Ctrl Pts',(-1.83174385734711,43.1576038253643,18.));
#27913=CARTESIAN_POINT('Ctrl Pts',(-1.87839202014609,43.065871623255,0.));
#27914=CARTESIAN_POINT('Ctrl Pts',(-1.87839202014609,43.065871623255,18.));
#27915=CARTESIAN_POINT('Ctrl Pts',(-1.92453321512436,42.9740309956624,0.));
#27916=CARTESIAN_POINT('Ctrl Pts',(-1.92453321512436,42.9740309956624,18.));
#27917=CARTESIAN_POINT('Ctrl Pts',(-1.97016390194216,42.8820834139973,0.));
#27918=CARTESIAN_POINT('Ctrl Pts',(-1.97016390194216,42.8820834139973,18.));
#27919=CARTESIAN_POINT('Ctrl Pts',(-2.01528067528089,42.7900301875309,0.));
#27920=CARTESIAN_POINT('Ctrl Pts',(-2.01528067528089,42.7900301875309,18.));
#27921=CARTESIAN_POINT('Ctrl Pts',(-2.05988014924519,42.6978725343209,0.));
#27922=CARTESIAN_POINT('Ctrl Pts',(-2.05988014924519,42.6978725343209,18.));
#27923=CARTESIAN_POINT('Ctrl Pts',(-2.10395886401771,42.6056116373456,0.));
#27924=CARTESIAN_POINT('Ctrl Pts',(-2.10395886401771,42.6056116373456,18.));
#27925=CARTESIAN_POINT('Ctrl Pts',(-2.14751319676745,42.5132487024335,0.));
#27926=CARTESIAN_POINT('Ctrl Pts',(-2.14751319676745,42.5132487024335,18.));
#27927=CARTESIAN_POINT('Ctrl Pts',(-2.19053924976737,42.4207850290047,0.));
#27928=CARTESIAN_POINT('Ctrl Pts',(-2.19053924976737,42.4207850290047,18.));
#27929=CARTESIAN_POINT('Ctrl Pts',(-2.233032874655,42.3282220118033,0.));
#27930=CARTESIAN_POINT('Ctrl Pts',(-2.233032874655,42.3282220118033,18.));
#27931=CARTESIAN_POINT('Ctrl Pts',(-2.27498976664774,42.2355611060784,0.));
#27932=CARTESIAN_POINT('Ctrl Pts',(-2.27498976664774,42.2355611060784,18.));
#27933=CARTESIAN_POINT('Ctrl Pts',(-2.31640554742808,42.1428038039937,0.));
#27934=CARTESIAN_POINT('Ctrl Pts',(-2.31640554742808,42.1428038039937,18.));
#27935=CARTESIAN_POINT('Ctrl Pts',(-2.35727584066429,42.0499516093661,0.));
#27936=CARTESIAN_POINT('Ctrl Pts',(-2.35727584066429,42.0499516093661,18.));
#27937=CARTESIAN_POINT('Ctrl Pts',(-2.39759639399648,41.9570060084039,0.));
#27938=CARTESIAN_POINT('Ctrl Pts',(-2.39759639399648,41.9570060084039,18.));
#27939=CARTESIAN_POINT('Ctrl Pts',(-2.437363014342,41.8639684667923,0.));
#27940=CARTESIAN_POINT('Ctrl Pts',(-2.437363014342,41.8639684667923,18.));
#27941=CARTESIAN_POINT('Ctrl Pts',(-2.47657137427693,41.7708404467533,0.));
#27942=CARTESIAN_POINT('Ctrl Pts',(-2.47657137427693,41.7708404467533,18.));
#27943=CARTESIAN_POINT('Ctrl Pts',(-2.51521684674477,41.6776234194583,0.));
#27944=CARTESIAN_POINT('Ctrl Pts',(-2.51521684674477,41.6776234194583,18.));
#27945=CARTESIAN_POINT('Ctrl Pts',(-2.55329436064184,41.5843188786284,0.));
#27946=CARTESIAN_POINT('Ctrl Pts',(-2.55329436064184,41.5843188786284,18.));
#27947=CARTESIAN_POINT('Ctrl Pts',(-2.59079818040171,41.4909283577703,0.));
#27948=CARTESIAN_POINT('Ctrl Pts',(-2.59079818040171,41.4909283577703,18.));
#27949=CARTESIAN_POINT('Ctrl Pts',(-2.62772200460656,41.3974534325936,0.));
#27950=CARTESIAN_POINT('Ctrl Pts',(-2.62772200460656,41.3974534325936,18.));
#27951=CARTESIAN_POINT('Ctrl Pts',(-2.66405934050118,41.3038957096306,0.));
#27952=CARTESIAN_POINT('Ctrl Pts',(-2.66405934050118,41.3038957096306,18.));
#27953=CARTESIAN_POINT('Ctrl Pts',(-2.69980383625015,41.2102568187956,0.));
#27954=CARTESIAN_POINT('Ctrl Pts',(-2.69980383625015,41.2102568187956,18.));
#27955=CARTESIAN_POINT('Ctrl Pts',(-2.73494956725005,41.1165384061145,0.));
#27956=CARTESIAN_POINT('Ctrl Pts',(-2.73494956725005,41.1165384061145,18.));
#27957=CARTESIAN_POINT('Ctrl Pts',(-2.76949151194863,41.0227421242398,0.));
#27958=CARTESIAN_POINT('Ctrl Pts',(-2.76949151194863,41.0227421242398,18.));
#27959=CARTESIAN_POINT('Ctrl Pts',(-2.80342531768405,40.9288696352159,0.));
#27960=CARTESIAN_POINT('Ctrl Pts',(-2.80342531768405,40.9288696352159,18.));
#27961=CARTESIAN_POINT('Ctrl Pts',(-2.83674635946679,40.8349226258683,0.));
#27962=CARTESIAN_POINT('Ctrl Pts',(-2.83674635946679,40.8349226258683,18.));
#27963=CARTESIAN_POINT('Ctrl Pts',(-2.86944892209898,40.7409028213129,0.));
#27964=CARTESIAN_POINT('Ctrl Pts',(-2.86944892209898,40.7409028213129,18.));
#27965=CARTESIAN_POINT('Ctrl Pts',(-2.90152548734343,40.6468119976928,0.));
#27966=CARTESIAN_POINT('Ctrl Pts',(-2.90152548734343,40.6468119976928,18.));
#27967=CARTESIAN_POINT('Ctrl Pts',(-2.93296560822893,40.5526520010651,0.));
#27968=CARTESIAN_POINT('Ctrl Pts',(-2.93296560822893,40.5526520010651,18.));
#27969=CARTESIAN_POINT('Ctrl Pts',(-2.96375636417322,40.4584247445196,0.));
#27970=CARTESIAN_POINT('Ctrl Pts',(-2.96375636417322,40.4584247445196,18.));
#27971=CARTESIAN_POINT('Ctrl Pts',(-2.99388446458219,40.3641321823444,0.));
#27972=CARTESIAN_POINT('Ctrl Pts',(-2.99388446458219,40.3641321823444,18.));
#27973=CARTESIAN_POINT('Ctrl Pts',(-3.02333808901595,40.2697762886113,0.));
#27974=CARTESIAN_POINT('Ctrl Pts',(-3.02333808901595,40.2697762886113,18.));
#27975=CARTESIAN_POINT('Ctrl Pts',(-3.0521084742307,40.1753590391515,0.));
#27976=CARTESIAN_POINT('Ctrl Pts',(-3.0521084742307,40.1753590391515,18.));
#27977=CARTESIAN_POINT('Ctrl Pts',(-3.08019251155015,40.0808823811787,0.));
#27978=CARTESIAN_POINT('Ctrl Pts',(-3.08019251155015,40.0808823811787,18.));
#27979=CARTESIAN_POINT('Ctrl Pts',(-3.10759149802908,39.9863482523153,0.));
#27980=CARTESIAN_POINT('Ctrl Pts',(-3.10759149802908,39.9863482523153,18.));
#27981=CARTESIAN_POINT('Ctrl Pts',(-3.13430604330356,39.8917586491576,0.));
#27982=CARTESIAN_POINT('Ctrl Pts',(-3.13430604330356,39.8917586491576,18.));
#27983=CARTESIAN_POINT('Ctrl Pts',(-3.16033160752804,39.7971156880138,0.));
#27984=CARTESIAN_POINT('Ctrl Pts',(-3.16033160752804,39.7971156880138,18.));
#27985=CARTESIAN_POINT('Ctrl Pts',(-3.18565465503835,39.7024216585552,0.));
#27986=CARTESIAN_POINT('Ctrl Pts',(-3.18565465503835,39.7024216585552,18.));
#27987=CARTESIAN_POINT('Ctrl Pts',(-3.21024640045595,39.607679107639,0.));
#27988=CARTESIAN_POINT('Ctrl Pts',(-3.21024640045595,39.607679107639,18.));
#27989=CARTESIAN_POINT('Ctrl Pts',(-3.23406609691661,39.5128908052622,0.));
#27990=CARTESIAN_POINT('Ctrl Pts',(-3.23406609691661,39.5128908052622,18.));
#27991=CARTESIAN_POINT('Ctrl Pts',(-3.25707264313388,39.4180596080755,0.));
#27992=CARTESIAN_POINT('Ctrl Pts',(-3.25707264313388,39.4180596080755,18.));
#27993=CARTESIAN_POINT('Ctrl Pts',(-3.27923485388117,39.3231883392913,0.));
#27994=CARTESIAN_POINT('Ctrl Pts',(-3.27923485388117,39.3231883392913,18.));
#27995=CARTESIAN_POINT('Ctrl Pts',(-3.30054018081687,39.2282796893977,0.));
#27996=CARTESIAN_POINT('Ctrl Pts',(-3.30054018081687,39.2282796893977,18.));
#27997=CARTESIAN_POINT('Ctrl Pts',(-3.32100933979557,39.1333360409949,0.));
#27998=CARTESIAN_POINT('Ctrl Pts',(-3.32100933979557,39.1333360409949,18.));
#27999=CARTESIAN_POINT('Ctrl Pts',(-3.34068601264472,39.0383596151636,0.));
#28000=CARTESIAN_POINT('Ctrl Pts',(-3.34068601264472,39.0383596151636,18.));
#28001=CARTESIAN_POINT('Ctrl Pts',(-3.35960922799481,38.9433528420174,0.));
#28002=CARTESIAN_POINT('Ctrl Pts',(-3.35960922799481,38.9433528420174,18.));
#28003=CARTESIAN_POINT('Ctrl Pts',(-3.37778863054482,38.8483186930884,0.));
#28004=CARTESIAN_POINT('Ctrl Pts',(-3.37778863054482,38.8483186930884,18.));
#28005=CARTESIAN_POINT('Ctrl Pts',(-3.39518333281818,38.7532609709905,0.));
#28006=CARTESIAN_POINT('Ctrl Pts',(-3.39518333281818,38.7532609709905,18.));
#28007=CARTESIAN_POINT('Ctrl Pts',(-3.41166717511901,38.6581847668347,0.));
#28008=CARTESIAN_POINT('Ctrl Pts',(-3.41166717511901,38.6581847668347,18.));
#28009=CARTESIAN_POINT('Ctrl Pts',(-3.42705871084997,38.5630961226878,0.));
#28010=CARTESIAN_POINT('Ctrl Pts',(-3.42705871084997,38.5630961226878,18.));
#28011=CARTESIAN_POINT('Ctrl Pts',(-3.44118343200303,38.4680013094732,0.));
#28012=CARTESIAN_POINT('Ctrl Pts',(-3.44118343200303,38.4680013094732,18.));
#28013=CARTESIAN_POINT('Ctrl Pts',(-3.45393053211023,38.3729061502716,0.));
#28014=CARTESIAN_POINT('Ctrl Pts',(-3.45393053211023,38.3729061502716,18.));
#28015=CARTESIAN_POINT('Ctrl Pts',(-3.46530185256872,38.2778154909527,0.));
#28016=CARTESIAN_POINT('Ctrl Pts',(-3.46530185256872,38.2778154909527,18.));
#28017=CARTESIAN_POINT('Ctrl Pts',(-3.47549027265411,38.1827321816559,0.));
#28018=CARTESIAN_POINT('Ctrl Pts',(-3.47549027265411,38.1827321816559,18.));
#28019=CARTESIAN_POINT('Ctrl Pts',(-3.48478279878233,38.0876589224537,0.));
#28020=CARTESIAN_POINT('Ctrl Pts',(-3.48478279878233,38.0876589224537,18.));
#28021=CARTESIAN_POINT('Ctrl Pts',(-3.49340804454645,37.9926009950482,0.));
#28022=CARTESIAN_POINT('Ctrl Pts',(-3.49340804454645,37.9926009950482,18.));
#28023=CARTESIAN_POINT('Ctrl Pts',(-3.50139628556083,37.8975688353863,0.));
#28024=CARTESIAN_POINT('Ctrl Pts',(-3.50139628556083,37.8975688353863,18.));
#28025=CARTESIAN_POINT('Ctrl Pts',(-3.50844720825128,37.8025803811856,0.));
#28026=CARTESIAN_POINT('Ctrl Pts',(-3.50844720825128,37.8025803811856,18.));
#28027=CARTESIAN_POINT('Ctrl Pts',(-3.51375922979957,37.7076643105286,0.));
#28028=CARTESIAN_POINT('Ctrl Pts',(-3.51375922979957,37.7076643105286,18.));
#28029=CARTESIAN_POINT('Ctrl Pts',(-3.51624243734645,37.6128545966533,0.));
#28030=CARTESIAN_POINT('Ctrl Pts',(-3.51624243734645,37.6128545966533,18.));
#28031=CARTESIAN_POINT('Ctrl Pts',(-3.51508109065209,37.5371179004295,0.));
#28032=CARTESIAN_POINT('Ctrl Pts',(-3.51508109065209,37.5371179004295,18.));
#28033=CARTESIAN_POINT('Ctrl Pts',(-3.51204731876361,37.4803889700239,0.));
#28034=CARTESIAN_POINT('Ctrl Pts',(-3.51204731876361,37.4803889700239,18.));
#28035=CARTESIAN_POINT('Ctrl Pts',(-3.50901346997657,37.4426037737699,0.));
#28036=CARTESIAN_POINT('Ctrl Pts',(-3.50901346997657,37.4426037737699,18.));
#28037=CARTESIAN_POINT('Ctrl Pts',(-3.50724370857673,37.4237196983922,0.));
#28038=CARTESIAN_POINT('Ctrl Pts',(-3.50724370857673,37.4237196983922,18.));
#28039=CARTESIAN_POINT('',(-1.38952890043929,43.9780537249529,0.));
#28040=CARTESIAN_POINT('Ctrl Pts',(-3.50724370857673,37.4237196983922,0.));
#28041=CARTESIAN_POINT('Ctrl Pts',(-3.50901346997657,37.4426037737699,0.));
#28042=CARTESIAN_POINT('Ctrl Pts',(-3.51204731876361,37.4803889700239,0.));
#28043=CARTESIAN_POINT('Ctrl Pts',(-3.51508109065209,37.5371179004295,0.));
#28044=CARTESIAN_POINT('Ctrl Pts',(-3.51624243734645,37.6128545966533,0.));
#28045=CARTESIAN_POINT('Ctrl Pts',(-3.51375922979957,37.7076643105286,0.));
#28046=CARTESIAN_POINT('Ctrl Pts',(-3.50844720825128,37.8025803811856,0.));
#28047=CARTESIAN_POINT('Ctrl Pts',(-3.50139628556083,37.8975688353863,0.));
#28048=CARTESIAN_POINT('Ctrl Pts',(-3.49340804454645,37.9926009950482,0.));
#28049=CARTESIAN_POINT('Ctrl Pts',(-3.48478279878233,38.0876589224537,0.));
#28050=CARTESIAN_POINT('Ctrl Pts',(-3.47549027265411,38.1827321816559,0.));
#28051=CARTESIAN_POINT('Ctrl Pts',(-3.46530185256872,38.2778154909527,0.));
#28052=CARTESIAN_POINT('Ctrl Pts',(-3.45393053211023,38.3729061502716,0.));
#28053=CARTESIAN_POINT('Ctrl Pts',(-3.44118343200303,38.4680013094732,0.));
#28054=CARTESIAN_POINT('Ctrl Pts',(-3.42705871084997,38.5630961226878,0.));
#28055=CARTESIAN_POINT('Ctrl Pts',(-3.41166717511901,38.6581847668347,0.));
#28056=CARTESIAN_POINT('Ctrl Pts',(-3.39518333281818,38.7532609709905,0.));
#28057=CARTESIAN_POINT('Ctrl Pts',(-3.37778863054482,38.8483186930884,0.));
#28058=CARTESIAN_POINT('Ctrl Pts',(-3.35960922799481,38.9433528420174,0.));
#28059=CARTESIAN_POINT('Ctrl Pts',(-3.34068601264472,39.0383596151636,0.));
#28060=CARTESIAN_POINT('Ctrl Pts',(-3.32100933979557,39.1333360409949,0.));
#28061=CARTESIAN_POINT('Ctrl Pts',(-3.30054018081687,39.2282796893977,0.));
#28062=CARTESIAN_POINT('Ctrl Pts',(-3.27923485388117,39.3231883392913,0.));
#28063=CARTESIAN_POINT('Ctrl Pts',(-3.25707264313388,39.4180596080755,0.));
#28064=CARTESIAN_POINT('Ctrl Pts',(-3.23406609691661,39.5128908052622,0.));
#28065=CARTESIAN_POINT('Ctrl Pts',(-3.21024640045595,39.607679107639,0.));
#28066=CARTESIAN_POINT('Ctrl Pts',(-3.18565465503835,39.7024216585552,0.));
#28067=CARTESIAN_POINT('Ctrl Pts',(-3.16033160752804,39.7971156880138,0.));
#28068=CARTESIAN_POINT('Ctrl Pts',(-3.13430604330356,39.8917586491576,0.));
#28069=CARTESIAN_POINT('Ctrl Pts',(-3.10759149802908,39.9863482523153,0.));
#28070=CARTESIAN_POINT('Ctrl Pts',(-3.08019251155015,40.0808823811787,0.));
#28071=CARTESIAN_POINT('Ctrl Pts',(-3.0521084742307,40.1753590391515,0.));
#28072=CARTESIAN_POINT('Ctrl Pts',(-3.02333808901595,40.2697762886113,0.));
#28073=CARTESIAN_POINT('Ctrl Pts',(-2.99388446458219,40.3641321823444,0.));
#28074=CARTESIAN_POINT('Ctrl Pts',(-2.96375636417322,40.4584247445196,0.));
#28075=CARTESIAN_POINT('Ctrl Pts',(-2.93296560822893,40.5526520010651,0.));
#28076=CARTESIAN_POINT('Ctrl Pts',(-2.90152548734343,40.6468119976928,0.));
#28077=CARTESIAN_POINT('Ctrl Pts',(-2.86944892209898,40.7409028213129,0.));
#28078=CARTESIAN_POINT('Ctrl Pts',(-2.83674635946679,40.8349226258683,0.));
#28079=CARTESIAN_POINT('Ctrl Pts',(-2.80342531768405,40.9288696352159,0.));
#28080=CARTESIAN_POINT('Ctrl Pts',(-2.76949151194863,41.0227421242398,0.));
#28081=CARTESIAN_POINT('Ctrl Pts',(-2.73494956725005,41.1165384061145,0.));
#28082=CARTESIAN_POINT('Ctrl Pts',(-2.69980383625015,41.2102568187956,0.));
#28083=CARTESIAN_POINT('Ctrl Pts',(-2.66405934050118,41.3038957096306,0.));
#28084=CARTESIAN_POINT('Ctrl Pts',(-2.62772200460656,41.3974534325936,0.));
#28085=CARTESIAN_POINT('Ctrl Pts',(-2.59079818040171,41.4909283577703,0.));
#28086=CARTESIAN_POINT('Ctrl Pts',(-2.55329436064184,41.5843188786284,0.));
#28087=CARTESIAN_POINT('Ctrl Pts',(-2.51521684674477,41.6776234194583,0.));
#28088=CARTESIAN_POINT('Ctrl Pts',(-2.47657137427693,41.7708404467533,0.));
#28089=CARTESIAN_POINT('Ctrl Pts',(-2.437363014342,41.8639684667923,0.));
#28090=CARTESIAN_POINT('Ctrl Pts',(-2.39759639399648,41.9570060084039,0.));
#28091=CARTESIAN_POINT('Ctrl Pts',(-2.35727584066429,42.0499516093661,0.));
#28092=CARTESIAN_POINT('Ctrl Pts',(-2.31640554742808,42.1428038039937,0.));
#28093=CARTESIAN_POINT('Ctrl Pts',(-2.27498976664774,42.2355611060784,0.));
#28094=CARTESIAN_POINT('Ctrl Pts',(-2.233032874655,42.3282220118033,0.));
#28095=CARTESIAN_POINT('Ctrl Pts',(-2.19053924976737,42.4207850290047,0.));
#28096=CARTESIAN_POINT('Ctrl Pts',(-2.14751319676745,42.5132487024335,0.));
#28097=CARTESIAN_POINT('Ctrl Pts',(-2.10395886401771,42.6056116373456,0.));
#28098=CARTESIAN_POINT('Ctrl Pts',(-2.05988014924519,42.6978725343209,0.));
#28099=CARTESIAN_POINT('Ctrl Pts',(-2.01528067528089,42.7900301875309,0.));
#28100=CARTESIAN_POINT('Ctrl Pts',(-1.97016390194216,42.8820834139973,0.));
#28101=CARTESIAN_POINT('Ctrl Pts',(-1.92453321512436,42.9740309956624,0.));
#28102=CARTESIAN_POINT('Ctrl Pts',(-1.87839202014609,43.065871623255,0.));
#28103=CARTESIAN_POINT('Ctrl Pts',(-1.83174385734711,43.1576038253643,0.));
#28104=CARTESIAN_POINT('Ctrl Pts',(-1.78459244842769,43.2492259505872,0.));
#28105=CARTESIAN_POINT('Ctrl Pts',(-1.73694151741124,43.3407363140236,0.));
#28106=CARTESIAN_POINT('Ctrl Pts',(-1.68879465270608,43.4321333178711,0.));
#28107=CARTESIAN_POINT('Ctrl Pts',(-1.64015515906648,43.5234155788248,0.));
#28108=CARTESIAN_POINT('Ctrl Pts',(-1.59102591108103,43.6145820637333,0.));
#28109=CARTESIAN_POINT('Ctrl Pts',(-1.53148589036097,43.7238422193529,0.));
#28110=CARTESIAN_POINT('Ctrl Pts',(-1.48126213998558,43.8147465842503,0.));
#28111=CARTESIAN_POINT('Ctrl Pts',(-1.44069595482723,43.8873767449247,0.));
#28112=CARTESIAN_POINT('Ctrl Pts',(-1.41005374202872,43.9417969186811,0.));
#28113=CARTESIAN_POINT('Ctrl Pts',(-1.38952890043916,43.9780537249529,0.));
#28114=CARTESIAN_POINT('',(-1.38952890043929,43.9780537249529,15.));
#28115=CARTESIAN_POINT('Ctrl Pts',(-1.38952890043916,43.9780537249529,15.));
#28116=CARTESIAN_POINT('Ctrl Pts',(-1.39979132121931,43.9599253218252,15.));
#28117=CARTESIAN_POINT('Ctrl Pts',(-1.42026781296156,43.9236568607623,15.));
#28118=CARTESIAN_POINT('Ctrl Pts',(-1.45083750111682,43.8692192047561,15.));
#28119=CARTESIAN_POINT('Ctrl Pts',(-1.49130689006066,43.7965657112708,15.));
#28120=CARTESIAN_POINT('Ctrl Pts',(-1.54140922714765,43.7056321934163,15.));
#28121=CARTESIAN_POINT('Ctrl Pts',(-1.59102591108103,43.6145820637333,15.));
#28122=CARTESIAN_POINT('Ctrl Pts',(-1.64015515906648,43.5234155788248,15.));
#28123=CARTESIAN_POINT('Ctrl Pts',(-1.68879465270608,43.4321333178711,15.));
#28124=CARTESIAN_POINT('Ctrl Pts',(-1.73694151741124,43.3407363140236,15.));
#28125=CARTESIAN_POINT('Ctrl Pts',(-1.78459244842769,43.2492259505872,15.));
#28126=CARTESIAN_POINT('Ctrl Pts',(-1.83174385734711,43.1576038253643,15.));
#28127=CARTESIAN_POINT('Ctrl Pts',(-1.87839202014609,43.065871623255,15.));
#28128=CARTESIAN_POINT('Ctrl Pts',(-1.92453321512436,42.9740309956624,15.));
#28129=CARTESIAN_POINT('Ctrl Pts',(-1.97016390194216,42.8820834139973,15.));
#28130=CARTESIAN_POINT('Ctrl Pts',(-2.01528067528089,42.7900301875309,15.));
#28131=CARTESIAN_POINT('Ctrl Pts',(-2.05988014924519,42.6978725343209,15.));
#28132=CARTESIAN_POINT('Ctrl Pts',(-2.10395886401771,42.6056116373456,15.));
#28133=CARTESIAN_POINT('Ctrl Pts',(-2.14751319676745,42.5132487024335,15.));
#28134=CARTESIAN_POINT('Ctrl Pts',(-2.19053924976737,42.4207850290047,15.));
#28135=CARTESIAN_POINT('Ctrl Pts',(-2.233032874655,42.3282220118033,15.));
#28136=CARTESIAN_POINT('Ctrl Pts',(-2.27498976664774,42.2355611060784,15.));
#28137=CARTESIAN_POINT('Ctrl Pts',(-2.31640554742808,42.1428038039937,15.));
#28138=CARTESIAN_POINT('Ctrl Pts',(-2.35727584066429,42.0499516093661,15.));
#28139=CARTESIAN_POINT('Ctrl Pts',(-2.39759639399648,41.9570060084039,15.));
#28140=CARTESIAN_POINT('Ctrl Pts',(-2.437363014342,41.8639684667923,15.));
#28141=CARTESIAN_POINT('Ctrl Pts',(-2.47657137427693,41.7708404467533,15.));
#28142=CARTESIAN_POINT('Ctrl Pts',(-2.51521684674477,41.6776234194583,15.));
#28143=CARTESIAN_POINT('Ctrl Pts',(-2.55329436064184,41.5843188786284,15.));
#28144=CARTESIAN_POINT('Ctrl Pts',(-2.59079818040171,41.4909283577703,15.));
#28145=CARTESIAN_POINT('Ctrl Pts',(-2.62772200460656,41.3974534325936,15.));
#28146=CARTESIAN_POINT('Ctrl Pts',(-2.66405934050118,41.3038957096306,15.));
#28147=CARTESIAN_POINT('Ctrl Pts',(-2.69980383625015,41.2102568187956,15.));
#28148=CARTESIAN_POINT('Ctrl Pts',(-2.73494956725005,41.1165384061145,15.));
#28149=CARTESIAN_POINT('Ctrl Pts',(-2.76949151194863,41.0227421242398,15.));
#28150=CARTESIAN_POINT('Ctrl Pts',(-2.80342531768405,40.9288696352159,15.));
#28151=CARTESIAN_POINT('Ctrl Pts',(-2.83674635946679,40.8349226258683,15.));
#28152=CARTESIAN_POINT('Ctrl Pts',(-2.86944892209898,40.7409028213129,15.));
#28153=CARTESIAN_POINT('Ctrl Pts',(-2.90152548734343,40.6468119976928,15.));
#28154=CARTESIAN_POINT('Ctrl Pts',(-2.93296560822893,40.5526520010651,15.));
#28155=CARTESIAN_POINT('Ctrl Pts',(-2.96375636417322,40.4584247445196,15.));
#28156=CARTESIAN_POINT('Ctrl Pts',(-2.99388446458219,40.3641321823444,15.));
#28157=CARTESIAN_POINT('Ctrl Pts',(-3.02333808901595,40.2697762886113,15.));
#28158=CARTESIAN_POINT('Ctrl Pts',(-3.0521084742307,40.1753590391515,15.));
#28159=CARTESIAN_POINT('Ctrl Pts',(-3.08019251155015,40.0808823811787,15.));
#28160=CARTESIAN_POINT('Ctrl Pts',(-3.10759149802908,39.9863482523153,15.));
#28161=CARTESIAN_POINT('Ctrl Pts',(-3.13430604330356,39.8917586491576,15.));
#28162=CARTESIAN_POINT('Ctrl Pts',(-3.16033160752804,39.7971156880138,15.));
#28163=CARTESIAN_POINT('Ctrl Pts',(-3.18565465503835,39.7024216585552,15.));
#28164=CARTESIAN_POINT('Ctrl Pts',(-3.21024640045595,39.607679107639,15.));
#28165=CARTESIAN_POINT('Ctrl Pts',(-3.23406609691661,39.5128908052622,15.));
#28166=CARTESIAN_POINT('Ctrl Pts',(-3.25707264313388,39.4180596080755,15.));
#28167=CARTESIAN_POINT('Ctrl Pts',(-3.27923485388117,39.3231883392913,15.));
#28168=CARTESIAN_POINT('Ctrl Pts',(-3.30054018081687,39.2282796893977,15.));
#28169=CARTESIAN_POINT('Ctrl Pts',(-3.32100933979557,39.1333360409949,15.));
#28170=CARTESIAN_POINT('Ctrl Pts',(-3.34068601264472,39.0383596151636,15.));
#28171=CARTESIAN_POINT('Ctrl Pts',(-3.35960922799481,38.9433528420174,15.));
#28172=CARTESIAN_POINT('Ctrl Pts',(-3.37778863054482,38.8483186930884,15.));
#28173=CARTESIAN_POINT('Ctrl Pts',(-3.39518333281818,38.7532609709905,15.));
#28174=CARTESIAN_POINT('Ctrl Pts',(-3.41166717511901,38.6581847668347,15.));
#28175=CARTESIAN_POINT('Ctrl Pts',(-3.42705871084997,38.5630961226878,15.));
#28176=CARTESIAN_POINT('Ctrl Pts',(-3.44118343200303,38.4680013094732,15.));
#28177=CARTESIAN_POINT('Ctrl Pts',(-3.45393053211023,38.3729061502716,15.));
#28178=CARTESIAN_POINT('Ctrl Pts',(-3.46530185256872,38.2778154909527,15.));
#28179=CARTESIAN_POINT('Ctrl Pts',(-3.47549027265411,38.1827321816559,15.));
#28180=CARTESIAN_POINT('Ctrl Pts',(-3.48478279878233,38.0876589224537,15.));
#28181=CARTESIAN_POINT('Ctrl Pts',(-3.49340804454645,37.9926009950482,15.));
#28182=CARTESIAN_POINT('Ctrl Pts',(-3.50139628556083,37.8975688353863,15.));
#28183=CARTESIAN_POINT('Ctrl Pts',(-3.50844720825128,37.8025803811856,15.));
#28184=CARTESIAN_POINT('Ctrl Pts',(-3.51375922979957,37.7076643105286,15.));
#28185=CARTESIAN_POINT('Ctrl Pts',(-3.51624243734645,37.6128545966533,15.));
#28186=CARTESIAN_POINT('Ctrl Pts',(-3.51508109065209,37.5371179004295,15.));
#28187=CARTESIAN_POINT('Ctrl Pts',(-3.51204731876361,37.4803889700239,15.));
#28188=CARTESIAN_POINT('Ctrl Pts',(-3.50901346997657,37.4426037737699,15.));
#28189=CARTESIAN_POINT('Ctrl Pts',(-3.50724370857673,37.4237196983922,15.));
#28190=CARTESIAN_POINT('',(-1.38952890043929,43.9780537249529,0.));
#28191=CARTESIAN_POINT('Origin',(0.,1.13331566353736E-11,0.));
#28192=CARTESIAN_POINT('',(1.38952890043917,43.9780537249529,0.));
#28193=CARTESIAN_POINT('Origin',(0.,1.13331566353736E-11,0.));
#28194=CARTESIAN_POINT('',(1.38952890043917,43.9780537249529,15.));
#28195=CARTESIAN_POINT('Origin',(0.,1.13331566353736E-11,15.));
#28196=CARTESIAN_POINT('',(1.38952890043917,43.9780537249529,0.));
#28197=CARTESIAN_POINT('Ctrl Pts',(3.50724370857673,37.4237196983923,0.));
#28198=CARTESIAN_POINT('Ctrl Pts',(3.50724370857673,37.4237196983923,18.));
#28199=CARTESIAN_POINT('Ctrl Pts',(3.50901346997657,37.4426037737699,0.));
#28200=CARTESIAN_POINT('Ctrl Pts',(3.50901346997657,37.4426037737699,18.));
#28201=CARTESIAN_POINT('Ctrl Pts',(3.51204731876361,37.4803889700239,0.));
#28202=CARTESIAN_POINT('Ctrl Pts',(3.51204731876361,37.4803889700239,18.));
#28203=CARTESIAN_POINT('Ctrl Pts',(3.5150810906521,37.5371179004295,0.));
#28204=CARTESIAN_POINT('Ctrl Pts',(3.5150810906521,37.5371179004295,18.));
#28205=CARTESIAN_POINT('Ctrl Pts',(3.51624243734645,37.6128545966533,0.));
#28206=CARTESIAN_POINT('Ctrl Pts',(3.51624243734645,37.6128545966533,18.));
#28207=CARTESIAN_POINT('Ctrl Pts',(3.51375922979958,37.7076643105286,0.));
#28208=CARTESIAN_POINT('Ctrl Pts',(3.51375922979958,37.7076643105286,18.));
#28209=CARTESIAN_POINT('Ctrl Pts',(3.50844720825128,37.8025803811856,0.));
#28210=CARTESIAN_POINT('Ctrl Pts',(3.50844720825128,37.8025803811856,18.));
#28211=CARTESIAN_POINT('Ctrl Pts',(3.50139628556084,37.8975688353863,0.));
#28212=CARTESIAN_POINT('Ctrl Pts',(3.50139628556084,37.8975688353863,18.));
#28213=CARTESIAN_POINT('Ctrl Pts',(3.49340804454646,37.9926009950482,0.));
#28214=CARTESIAN_POINT('Ctrl Pts',(3.49340804454646,37.9926009950482,18.));
#28215=CARTESIAN_POINT('Ctrl Pts',(3.48478279878234,38.0876589224537,0.));
#28216=CARTESIAN_POINT('Ctrl Pts',(3.48478279878234,38.0876589224537,18.));
#28217=CARTESIAN_POINT('Ctrl Pts',(3.47549027265412,38.1827321816559,0.));
#28218=CARTESIAN_POINT('Ctrl Pts',(3.47549027265412,38.1827321816559,18.));
#28219=CARTESIAN_POINT('Ctrl Pts',(3.46530185256873,38.2778154909527,0.));
#28220=CARTESIAN_POINT('Ctrl Pts',(3.46530185256873,38.2778154909527,18.));
#28221=CARTESIAN_POINT('Ctrl Pts',(3.45393053211023,38.3729061502716,0.));
#28222=CARTESIAN_POINT('Ctrl Pts',(3.45393053211023,38.3729061502716,18.));
#28223=CARTESIAN_POINT('Ctrl Pts',(3.44118343200303,38.4680013094732,0.));
#28224=CARTESIAN_POINT('Ctrl Pts',(3.44118343200303,38.4680013094732,18.));
#28225=CARTESIAN_POINT('Ctrl Pts',(3.42705871084997,38.5630961226878,0.));
#28226=CARTESIAN_POINT('Ctrl Pts',(3.42705871084997,38.5630961226878,18.));
#28227=CARTESIAN_POINT('Ctrl Pts',(3.41166717511901,38.6581847668347,0.));
#28228=CARTESIAN_POINT('Ctrl Pts',(3.41166717511901,38.6581847668347,18.));
#28229=CARTESIAN_POINT('Ctrl Pts',(3.39518333281818,38.7532609709905,0.));
#28230=CARTESIAN_POINT('Ctrl Pts',(3.39518333281818,38.7532609709905,18.));
#28231=CARTESIAN_POINT('Ctrl Pts',(3.37778863054482,38.8483186930884,0.));
#28232=CARTESIAN_POINT('Ctrl Pts',(3.37778863054482,38.8483186930884,18.));
#28233=CARTESIAN_POINT('Ctrl Pts',(3.35960922799481,38.9433528420174,0.));
#28234=CARTESIAN_POINT('Ctrl Pts',(3.35960922799481,38.9433528420174,18.));
#28235=CARTESIAN_POINT('Ctrl Pts',(3.34068601264472,39.0383596151636,0.));
#28236=CARTESIAN_POINT('Ctrl Pts',(3.34068601264472,39.0383596151636,18.));
#28237=CARTESIAN_POINT('Ctrl Pts',(3.32100933979558,39.1333360409949,0.));
#28238=CARTESIAN_POINT('Ctrl Pts',(3.32100933979558,39.1333360409949,18.));
#28239=CARTESIAN_POINT('Ctrl Pts',(3.30054018081688,39.2282796893977,0.));
#28240=CARTESIAN_POINT('Ctrl Pts',(3.30054018081688,39.2282796893977,18.));
#28241=CARTESIAN_POINT('Ctrl Pts',(3.27923485388118,39.3231883392913,0.));
#28242=CARTESIAN_POINT('Ctrl Pts',(3.27923485388118,39.3231883392913,18.));
#28243=CARTESIAN_POINT('Ctrl Pts',(3.25707264313388,39.4180596080755,0.));
#28244=CARTESIAN_POINT('Ctrl Pts',(3.25707264313388,39.4180596080755,18.));
#28245=CARTESIAN_POINT('Ctrl Pts',(3.23406609691661,39.5128908052622,0.));
#28246=CARTESIAN_POINT('Ctrl Pts',(3.23406609691661,39.5128908052622,18.));
#28247=CARTESIAN_POINT('Ctrl Pts',(3.21024640045595,39.607679107639,0.));
#28248=CARTESIAN_POINT('Ctrl Pts',(3.21024640045595,39.607679107639,18.));
#28249=CARTESIAN_POINT('Ctrl Pts',(3.18565465503836,39.7024216585552,0.));
#28250=CARTESIAN_POINT('Ctrl Pts',(3.18565465503836,39.7024216585552,18.));
#28251=CARTESIAN_POINT('Ctrl Pts',(3.16033160752804,39.7971156880138,0.));
#28252=CARTESIAN_POINT('Ctrl Pts',(3.16033160752804,39.7971156880138,18.));
#28253=CARTESIAN_POINT('Ctrl Pts',(3.13430604330356,39.8917586491576,0.));
#28254=CARTESIAN_POINT('Ctrl Pts',(3.13430604330356,39.8917586491576,18.));
#28255=CARTESIAN_POINT('Ctrl Pts',(3.10759149802908,39.9863482523153,0.));
#28256=CARTESIAN_POINT('Ctrl Pts',(3.10759149802908,39.9863482523153,18.));
#28257=CARTESIAN_POINT('Ctrl Pts',(3.08019251155016,40.0808823811787,0.));
#28258=CARTESIAN_POINT('Ctrl Pts',(3.08019251155016,40.0808823811787,18.));
#28259=CARTESIAN_POINT('Ctrl Pts',(3.05210847423071,40.1753590391515,0.));
#28260=CARTESIAN_POINT('Ctrl Pts',(3.05210847423071,40.1753590391515,18.));
#28261=CARTESIAN_POINT('Ctrl Pts',(3.02333808901595,40.2697762886113,0.));
#28262=CARTESIAN_POINT('Ctrl Pts',(3.02333808901595,40.2697762886113,18.));
#28263=CARTESIAN_POINT('Ctrl Pts',(2.9938844645822,40.3641321823444,0.));
#28264=CARTESIAN_POINT('Ctrl Pts',(2.9938844645822,40.3641321823444,18.));
#28265=CARTESIAN_POINT('Ctrl Pts',(2.96375636417323,40.4584247445196,0.));
#28266=CARTESIAN_POINT('Ctrl Pts',(2.96375636417323,40.4584247445196,18.));
#28267=CARTESIAN_POINT('Ctrl Pts',(2.93296560822894,40.5526520010651,0.));
#28268=CARTESIAN_POINT('Ctrl Pts',(2.93296560822894,40.5526520010651,18.));
#28269=CARTESIAN_POINT('Ctrl Pts',(2.90152548734343,40.6468119976928,0.));
#28270=CARTESIAN_POINT('Ctrl Pts',(2.90152548734343,40.6468119976928,18.));
#28271=CARTESIAN_POINT('Ctrl Pts',(2.86944892209898,40.7409028213129,0.));
#28272=CARTESIAN_POINT('Ctrl Pts',(2.86944892209898,40.7409028213129,18.));
#28273=CARTESIAN_POINT('Ctrl Pts',(2.8367463594668,40.8349226258683,0.));
#28274=CARTESIAN_POINT('Ctrl Pts',(2.8367463594668,40.8349226258683,18.));
#28275=CARTESIAN_POINT('Ctrl Pts',(2.80342531768405,40.9288696352159,0.));
#28276=CARTESIAN_POINT('Ctrl Pts',(2.80342531768405,40.9288696352159,18.));
#28277=CARTESIAN_POINT('Ctrl Pts',(2.76949151194864,41.0227421242398,0.));
#28278=CARTESIAN_POINT('Ctrl Pts',(2.76949151194864,41.0227421242398,18.));
#28279=CARTESIAN_POINT('Ctrl Pts',(2.73494956725006,41.1165384061145,0.));
#28280=CARTESIAN_POINT('Ctrl Pts',(2.73494956725006,41.1165384061145,18.));
#28281=CARTESIAN_POINT('Ctrl Pts',(2.69980383625016,41.2102568187956,0.));
#28282=CARTESIAN_POINT('Ctrl Pts',(2.69980383625016,41.2102568187956,18.));
#28283=CARTESIAN_POINT('Ctrl Pts',(2.66405934050118,41.3038957096306,0.));
#28284=CARTESIAN_POINT('Ctrl Pts',(2.66405934050118,41.3038957096306,18.));
#28285=CARTESIAN_POINT('Ctrl Pts',(2.62772200460657,41.3974534325937,0.));
#28286=CARTESIAN_POINT('Ctrl Pts',(2.62772200460657,41.3974534325937,18.));
#28287=CARTESIAN_POINT('Ctrl Pts',(2.59079818040172,41.4909283577703,0.));
#28288=CARTESIAN_POINT('Ctrl Pts',(2.59079818040172,41.4909283577703,18.));
#28289=CARTESIAN_POINT('Ctrl Pts',(2.55329436064184,41.5843188786284,0.));
#28290=CARTESIAN_POINT('Ctrl Pts',(2.55329436064184,41.5843188786284,18.));
#28291=CARTESIAN_POINT('Ctrl Pts',(2.51521684674477,41.6776234194583,0.));
#28292=CARTESIAN_POINT('Ctrl Pts',(2.51521684674477,41.6776234194583,18.));
#28293=CARTESIAN_POINT('Ctrl Pts',(2.47657137427693,41.7708404467533,0.));
#28294=CARTESIAN_POINT('Ctrl Pts',(2.47657137427693,41.7708404467533,18.));
#28295=CARTESIAN_POINT('Ctrl Pts',(2.43736301434201,41.8639684667923,0.));
#28296=CARTESIAN_POINT('Ctrl Pts',(2.43736301434201,41.8639684667923,18.));
#28297=CARTESIAN_POINT('Ctrl Pts',(2.39759639399648,41.9570060084039,0.));
#28298=CARTESIAN_POINT('Ctrl Pts',(2.39759639399648,41.9570060084039,18.));
#28299=CARTESIAN_POINT('Ctrl Pts',(2.35727584066429,42.0499516093661,0.));
#28300=CARTESIAN_POINT('Ctrl Pts',(2.35727584066429,42.0499516093661,18.));
#28301=CARTESIAN_POINT('Ctrl Pts',(2.3164055474281,42.1428038039937,0.));
#28302=CARTESIAN_POINT('Ctrl Pts',(2.3164055474281,42.1428038039937,18.));
#28303=CARTESIAN_POINT('Ctrl Pts',(2.27498976664775,42.2355611060784,0.));
#28304=CARTESIAN_POINT('Ctrl Pts',(2.27498976664775,42.2355611060784,18.));
#28305=CARTESIAN_POINT('Ctrl Pts',(2.233032874655,42.3282220118033,0.));
#28306=CARTESIAN_POINT('Ctrl Pts',(2.233032874655,42.3282220118033,18.));
#28307=CARTESIAN_POINT('Ctrl Pts',(2.19053924976738,42.4207850290047,0.));
#28308=CARTESIAN_POINT('Ctrl Pts',(2.19053924976738,42.4207850290047,18.));
#28309=CARTESIAN_POINT('Ctrl Pts',(2.14751319676746,42.5132487024335,0.));
#28310=CARTESIAN_POINT('Ctrl Pts',(2.14751319676746,42.5132487024335,18.));
#28311=CARTESIAN_POINT('Ctrl Pts',(2.10395886401771,42.6056116373456,0.));
#28312=CARTESIAN_POINT('Ctrl Pts',(2.10395886401771,42.6056116373456,18.));
#28313=CARTESIAN_POINT('Ctrl Pts',(2.05988014924519,42.6978725343209,0.));
#28314=CARTESIAN_POINT('Ctrl Pts',(2.05988014924519,42.6978725343209,18.));
#28315=CARTESIAN_POINT('Ctrl Pts',(2.01528067528089,42.7900301875309,0.));
#28316=CARTESIAN_POINT('Ctrl Pts',(2.01528067528089,42.7900301875309,18.));
#28317=CARTESIAN_POINT('Ctrl Pts',(1.97016390194216,42.8820834139973,0.));
#28318=CARTESIAN_POINT('Ctrl Pts',(1.97016390194216,42.8820834139973,18.));
#28319=CARTESIAN_POINT('Ctrl Pts',(1.92453321512436,42.9740309956624,0.));
#28320=CARTESIAN_POINT('Ctrl Pts',(1.92453321512436,42.9740309956624,18.));
#28321=CARTESIAN_POINT('Ctrl Pts',(1.87839202014609,43.065871623255,0.));
#28322=CARTESIAN_POINT('Ctrl Pts',(1.87839202014609,43.065871623255,18.));
#28323=CARTESIAN_POINT('Ctrl Pts',(1.83174385734712,43.1576038253643,0.));
#28324=CARTESIAN_POINT('Ctrl Pts',(1.83174385734712,43.1576038253643,18.));
#28325=CARTESIAN_POINT('Ctrl Pts',(1.7845924484277,43.2492259505872,0.));
#28326=CARTESIAN_POINT('Ctrl Pts',(1.7845924484277,43.2492259505872,18.));
#28327=CARTESIAN_POINT('Ctrl Pts',(1.73694151741124,43.3407363140236,0.));
#28328=CARTESIAN_POINT('Ctrl Pts',(1.73694151741124,43.3407363140236,18.));
#28329=CARTESIAN_POINT('Ctrl Pts',(1.68879465270608,43.4321333178711,0.));
#28330=CARTESIAN_POINT('Ctrl Pts',(1.68879465270608,43.4321333178711,18.));
#28331=CARTESIAN_POINT('Ctrl Pts',(1.64015515906649,43.5234155788248,0.));
#28332=CARTESIAN_POINT('Ctrl Pts',(1.64015515906649,43.5234155788248,18.));
#28333=CARTESIAN_POINT('Ctrl Pts',(1.59102591108104,43.6145820637333,0.));
#28334=CARTESIAN_POINT('Ctrl Pts',(1.59102591108104,43.6145820637333,18.));
#28335=CARTESIAN_POINT('Ctrl Pts',(1.54140922714765,43.7056321934163,0.));
#28336=CARTESIAN_POINT('Ctrl Pts',(1.54140922714765,43.7056321934163,18.));
#28337=CARTESIAN_POINT('Ctrl Pts',(1.49130689006067,43.7965657112708,0.));
#28338=CARTESIAN_POINT('Ctrl Pts',(1.49130689006067,43.7965657112708,18.));
#28339=CARTESIAN_POINT('Ctrl Pts',(1.45083750111682,43.8692192047561,0.));
#28340=CARTESIAN_POINT('Ctrl Pts',(1.45083750111682,43.8692192047561,18.));
#28341=CARTESIAN_POINT('Ctrl Pts',(1.42026781296157,43.9236568607623,0.));
#28342=CARTESIAN_POINT('Ctrl Pts',(1.42026781296157,43.9236568607623,18.));
#28343=CARTESIAN_POINT('Ctrl Pts',(1.39979132121931,43.9599253218251,0.));
#28344=CARTESIAN_POINT('Ctrl Pts',(1.39979132121931,43.9599253218251,18.));
#28345=CARTESIAN_POINT('Ctrl Pts',(1.38952890043916,43.9780537249529,0.));
#28346=CARTESIAN_POINT('Ctrl Pts',(1.38952890043916,43.9780537249529,18.));
#28347=CARTESIAN_POINT('Ctrl Pts',(3.50724370857673,37.4237196983923,0.));
#28348=CARTESIAN_POINT('Ctrl Pts',(3.50901346997657,37.4426037737699,0.));
#28349=CARTESIAN_POINT('Ctrl Pts',(3.51204731876361,37.4803889700239,0.));
#28350=CARTESIAN_POINT('Ctrl Pts',(3.5150810906521,37.5371179004295,0.));
#28351=CARTESIAN_POINT('Ctrl Pts',(3.51624243734645,37.6128545966533,0.));
#28352=CARTESIAN_POINT('Ctrl Pts',(3.51375922979958,37.7076643105286,0.));
#28353=CARTESIAN_POINT('Ctrl Pts',(3.50844720825128,37.8025803811856,0.));
#28354=CARTESIAN_POINT('Ctrl Pts',(3.50139628556084,37.8975688353863,0.));
#28355=CARTESIAN_POINT('Ctrl Pts',(3.49340804454646,37.9926009950482,0.));
#28356=CARTESIAN_POINT('Ctrl Pts',(3.48478279878234,38.0876589224537,0.));
#28357=CARTESIAN_POINT('Ctrl Pts',(3.47549027265412,38.1827321816559,0.));
#28358=CARTESIAN_POINT('Ctrl Pts',(3.46530185256873,38.2778154909527,0.));
#28359=CARTESIAN_POINT('Ctrl Pts',(3.45393053211023,38.3729061502716,0.));
#28360=CARTESIAN_POINT('Ctrl Pts',(3.44118343200303,38.4680013094732,0.));
#28361=CARTESIAN_POINT('Ctrl Pts',(3.42705871084997,38.5630961226878,0.));
#28362=CARTESIAN_POINT('Ctrl Pts',(3.41166717511901,38.6581847668347,0.));
#28363=CARTESIAN_POINT('Ctrl Pts',(3.39518333281818,38.7532609709905,0.));
#28364=CARTESIAN_POINT('Ctrl Pts',(3.37778863054482,38.8483186930884,0.));
#28365=CARTESIAN_POINT('Ctrl Pts',(3.35960922799481,38.9433528420174,0.));
#28366=CARTESIAN_POINT('Ctrl Pts',(3.34068601264472,39.0383596151636,0.));
#28367=CARTESIAN_POINT('Ctrl Pts',(3.32100933979558,39.1333360409949,0.));
#28368=CARTESIAN_POINT('Ctrl Pts',(3.30054018081688,39.2282796893977,0.));
#28369=CARTESIAN_POINT('Ctrl Pts',(3.27923485388118,39.3231883392913,0.));
#28370=CARTESIAN_POINT('Ctrl Pts',(3.25707264313388,39.4180596080755,0.));
#28371=CARTESIAN_POINT('Ctrl Pts',(3.23406609691661,39.5128908052622,0.));
#28372=CARTESIAN_POINT('Ctrl Pts',(3.21024640045595,39.607679107639,0.));
#28373=CARTESIAN_POINT('Ctrl Pts',(3.18565465503836,39.7024216585552,0.));
#28374=CARTESIAN_POINT('Ctrl Pts',(3.16033160752804,39.7971156880138,0.));
#28375=CARTESIAN_POINT('Ctrl Pts',(3.13430604330356,39.8917586491576,0.));
#28376=CARTESIAN_POINT('Ctrl Pts',(3.10759149802908,39.9863482523153,0.));
#28377=CARTESIAN_POINT('Ctrl Pts',(3.08019251155016,40.0808823811787,0.));
#28378=CARTESIAN_POINT('Ctrl Pts',(3.05210847423071,40.1753590391515,0.));
#28379=CARTESIAN_POINT('Ctrl Pts',(3.02333808901595,40.2697762886113,0.));
#28380=CARTESIAN_POINT('Ctrl Pts',(2.9938844645822,40.3641321823444,0.));
#28381=CARTESIAN_POINT('Ctrl Pts',(2.96375636417323,40.4584247445196,0.));
#28382=CARTESIAN_POINT('Ctrl Pts',(2.93296560822894,40.5526520010651,0.));
#28383=CARTESIAN_POINT('Ctrl Pts',(2.90152548734343,40.6468119976928,0.));
#28384=CARTESIAN_POINT('Ctrl Pts',(2.86944892209898,40.7409028213129,0.));
#28385=CARTESIAN_POINT('Ctrl Pts',(2.8367463594668,40.8349226258683,0.));
#28386=CARTESIAN_POINT('Ctrl Pts',(2.80342531768405,40.9288696352159,0.));
#28387=CARTESIAN_POINT('Ctrl Pts',(2.76949151194864,41.0227421242398,0.));
#28388=CARTESIAN_POINT('Ctrl Pts',(2.73494956725006,41.1165384061145,0.));
#28389=CARTESIAN_POINT('Ctrl Pts',(2.69980383625016,41.2102568187956,0.));
#28390=CARTESIAN_POINT('Ctrl Pts',(2.66405934050118,41.3038957096306,0.));
#28391=CARTESIAN_POINT('Ctrl Pts',(2.62772200460657,41.3974534325937,0.));
#28392=CARTESIAN_POINT('Ctrl Pts',(2.59079818040172,41.4909283577703,0.));
#28393=CARTESIAN_POINT('Ctrl Pts',(2.55329436064184,41.5843188786284,0.));
#28394=CARTESIAN_POINT('Ctrl Pts',(2.51521684674477,41.6776234194583,0.));
#28395=CARTESIAN_POINT('Ctrl Pts',(2.47657137427693,41.7708404467533,0.));
#28396=CARTESIAN_POINT('Ctrl Pts',(2.43736301434201,41.8639684667923,0.));
#28397=CARTESIAN_POINT('Ctrl Pts',(2.39759639399648,41.9570060084039,0.));
#28398=CARTESIAN_POINT('Ctrl Pts',(2.35727584066429,42.0499516093661,0.));
#28399=CARTESIAN_POINT('Ctrl Pts',(2.3164055474281,42.1428038039937,0.));
#28400=CARTESIAN_POINT('Ctrl Pts',(2.27498976664775,42.2355611060784,0.));
#28401=CARTESIAN_POINT('Ctrl Pts',(2.233032874655,42.3282220118033,0.));
#28402=CARTESIAN_POINT('Ctrl Pts',(2.19053924976738,42.4207850290047,0.));
#28403=CARTESIAN_POINT('Ctrl Pts',(2.14751319676746,42.5132487024335,0.));
#28404=CARTESIAN_POINT('Ctrl Pts',(2.10395886401771,42.6056116373456,0.));
#28405=CARTESIAN_POINT('Ctrl Pts',(2.05988014924519,42.6978725343209,0.));
#28406=CARTESIAN_POINT('Ctrl Pts',(2.01528067528089,42.7900301875309,0.));
#28407=CARTESIAN_POINT('Ctrl Pts',(1.97016390194216,42.8820834139973,0.));
#28408=CARTESIAN_POINT('Ctrl Pts',(1.92453321512436,42.9740309956624,0.));
#28409=CARTESIAN_POINT('Ctrl Pts',(1.87839202014609,43.065871623255,0.));
#28410=CARTESIAN_POINT('Ctrl Pts',(1.83174385734712,43.1576038253643,0.));
#28411=CARTESIAN_POINT('Ctrl Pts',(1.7845924484277,43.2492259505872,0.));
#28412=CARTESIAN_POINT('Ctrl Pts',(1.73694151741124,43.3407363140236,0.));
#28413=CARTESIAN_POINT('Ctrl Pts',(1.68879465270608,43.4321333178711,0.));
#28414=CARTESIAN_POINT('Ctrl Pts',(1.64015515906649,43.5234155788248,0.));
#28415=CARTESIAN_POINT('Ctrl Pts',(1.59102591108104,43.6145820637333,0.));
#28416=CARTESIAN_POINT('Ctrl Pts',(1.53148589036097,43.7238422193529,0.));
#28417=CARTESIAN_POINT('Ctrl Pts',(1.48126213998559,43.8147465842503,0.));
#28418=CARTESIAN_POINT('Ctrl Pts',(1.44069595482723,43.8873767449247,0.));
#28419=CARTESIAN_POINT('Ctrl Pts',(1.41005374202874,43.9417969186811,0.));
#28420=CARTESIAN_POINT('Ctrl Pts',(1.38952890043916,43.9780537249529,0.));
#28421=CARTESIAN_POINT('Ctrl Pts',(3.50724370857673,37.4237196983923,15.));
#28422=CARTESIAN_POINT('Ctrl Pts',(3.50901346997657,37.4426037737699,15.));
#28423=CARTESIAN_POINT('Ctrl Pts',(3.51204731876361,37.4803889700239,15.));
#28424=CARTESIAN_POINT('Ctrl Pts',(3.5150810906521,37.5371179004295,15.));
#28425=CARTESIAN_POINT('Ctrl Pts',(3.51624243734645,37.6128545966533,15.));
#28426=CARTESIAN_POINT('Ctrl Pts',(3.51375922979958,37.7076643105286,15.));
#28427=CARTESIAN_POINT('Ctrl Pts',(3.50844720825128,37.8025803811856,15.));
#28428=CARTESIAN_POINT('Ctrl Pts',(3.50139628556084,37.8975688353863,15.));
#28429=CARTESIAN_POINT('Ctrl Pts',(3.49340804454646,37.9926009950482,15.));
#28430=CARTESIAN_POINT('Ctrl Pts',(3.48478279878234,38.0876589224537,15.));
#28431=CARTESIAN_POINT('Ctrl Pts',(3.47549027265412,38.1827321816559,15.));
#28432=CARTESIAN_POINT('Ctrl Pts',(3.46530185256873,38.2778154909527,15.));
#28433=CARTESIAN_POINT('Ctrl Pts',(3.45393053211023,38.3729061502716,15.));
#28434=CARTESIAN_POINT('Ctrl Pts',(3.44118343200303,38.4680013094732,15.));
#28435=CARTESIAN_POINT('Ctrl Pts',(3.42705871084997,38.5630961226878,15.));
#28436=CARTESIAN_POINT('Ctrl Pts',(3.41166717511901,38.6581847668347,15.));
#28437=CARTESIAN_POINT('Ctrl Pts',(3.39518333281818,38.7532609709905,15.));
#28438=CARTESIAN_POINT('Ctrl Pts',(3.37778863054482,38.8483186930884,15.));
#28439=CARTESIAN_POINT('Ctrl Pts',(3.35960922799481,38.9433528420174,15.));
#28440=CARTESIAN_POINT('Ctrl Pts',(3.34068601264472,39.0383596151636,15.));
#28441=CARTESIAN_POINT('Ctrl Pts',(3.32100933979558,39.1333360409949,15.));
#28442=CARTESIAN_POINT('Ctrl Pts',(3.30054018081688,39.2282796893977,15.));
#28443=CARTESIAN_POINT('Ctrl Pts',(3.27923485388118,39.3231883392913,15.));
#28444=CARTESIAN_POINT('Ctrl Pts',(3.25707264313388,39.4180596080755,15.));
#28445=CARTESIAN_POINT('Ctrl Pts',(3.23406609691661,39.5128908052622,15.));
#28446=CARTESIAN_POINT('Ctrl Pts',(3.21024640045595,39.607679107639,15.));
#28447=CARTESIAN_POINT('Ctrl Pts',(3.18565465503836,39.7024216585552,15.));
#28448=CARTESIAN_POINT('Ctrl Pts',(3.16033160752804,39.7971156880138,15.));
#28449=CARTESIAN_POINT('Ctrl Pts',(3.13430604330356,39.8917586491576,15.));
#28450=CARTESIAN_POINT('Ctrl Pts',(3.10759149802908,39.9863482523153,15.));
#28451=CARTESIAN_POINT('Ctrl Pts',(3.08019251155016,40.0808823811787,15.));
#28452=CARTESIAN_POINT('Ctrl Pts',(3.05210847423071,40.1753590391515,15.));
#28453=CARTESIAN_POINT('Ctrl Pts',(3.02333808901595,40.2697762886113,15.));
#28454=CARTESIAN_POINT('Ctrl Pts',(2.9938844645822,40.3641321823444,15.));
#28455=CARTESIAN_POINT('Ctrl Pts',(2.96375636417323,40.4584247445196,15.));
#28456=CARTESIAN_POINT('Ctrl Pts',(2.93296560822894,40.5526520010651,15.));
#28457=CARTESIAN_POINT('Ctrl Pts',(2.90152548734343,40.6468119976928,15.));
#28458=CARTESIAN_POINT('Ctrl Pts',(2.86944892209898,40.7409028213129,15.));
#28459=CARTESIAN_POINT('Ctrl Pts',(2.8367463594668,40.8349226258683,15.));
#28460=CARTESIAN_POINT('Ctrl Pts',(2.80342531768405,40.9288696352159,15.));
#28461=CARTESIAN_POINT('Ctrl Pts',(2.76949151194864,41.0227421242398,15.));
#28462=CARTESIAN_POINT('Ctrl Pts',(2.73494956725006,41.1165384061145,15.));
#28463=CARTESIAN_POINT('Ctrl Pts',(2.69980383625016,41.2102568187956,15.));
#28464=CARTESIAN_POINT('Ctrl Pts',(2.66405934050118,41.3038957096306,15.));
#28465=CARTESIAN_POINT('Ctrl Pts',(2.62772200460657,41.3974534325937,15.));
#28466=CARTESIAN_POINT('Ctrl Pts',(2.59079818040172,41.4909283577703,15.));
#28467=CARTESIAN_POINT('Ctrl Pts',(2.55329436064184,41.5843188786284,15.));
#28468=CARTESIAN_POINT('Ctrl Pts',(2.51521684674477,41.6776234194583,15.));
#28469=CARTESIAN_POINT('Ctrl Pts',(2.47657137427693,41.7708404467533,15.));
#28470=CARTESIAN_POINT('Ctrl Pts',(2.43736301434201,41.8639684667923,15.));
#28471=CARTESIAN_POINT('Ctrl Pts',(2.39759639399648,41.9570060084039,15.));
#28472=CARTESIAN_POINT('Ctrl Pts',(2.35727584066429,42.0499516093661,15.));
#28473=CARTESIAN_POINT('Ctrl Pts',(2.3164055474281,42.1428038039937,15.));
#28474=CARTESIAN_POINT('Ctrl Pts',(2.27498976664775,42.2355611060784,15.));
#28475=CARTESIAN_POINT('Ctrl Pts',(2.233032874655,42.3282220118033,15.));
#28476=CARTESIAN_POINT('Ctrl Pts',(2.19053924976738,42.4207850290047,15.));
#28477=CARTESIAN_POINT('Ctrl Pts',(2.14751319676746,42.5132487024335,15.));
#28478=CARTESIAN_POINT('Ctrl Pts',(2.10395886401771,42.6056116373456,15.));
#28479=CARTESIAN_POINT('Ctrl Pts',(2.05988014924519,42.6978725343209,15.));
#28480=CARTESIAN_POINT('Ctrl Pts',(2.01528067528089,42.7900301875309,15.));
#28481=CARTESIAN_POINT('Ctrl Pts',(1.97016390194216,42.8820834139973,15.));
#28482=CARTESIAN_POINT('Ctrl Pts',(1.92453321512436,42.9740309956624,15.));
#28483=CARTESIAN_POINT('Ctrl Pts',(1.87839202014609,43.065871623255,15.));
#28484=CARTESIAN_POINT('Ctrl Pts',(1.83174385734712,43.1576038253643,15.));
#28485=CARTESIAN_POINT('Ctrl Pts',(1.7845924484277,43.2492259505872,15.));
#28486=CARTESIAN_POINT('Ctrl Pts',(1.73694151741124,43.3407363140236,15.));
#28487=CARTESIAN_POINT('Ctrl Pts',(1.68879465270608,43.4321333178711,15.));
#28488=CARTESIAN_POINT('Ctrl Pts',(1.64015515906649,43.5234155788248,15.));
#28489=CARTESIAN_POINT('Ctrl Pts',(1.59102591108104,43.6145820637333,15.));
#28490=CARTESIAN_POINT('Ctrl Pts',(1.53148589036097,43.7238422193529,15.));
#28491=CARTESIAN_POINT('Ctrl Pts',(1.48126213998559,43.8147465842503,15.));
#28492=CARTESIAN_POINT('Ctrl Pts',(1.44069595482723,43.8873767449247,15.));
#28493=CARTESIAN_POINT('Ctrl Pts',(1.41005374202874,43.9417969186811,15.));
#28494=CARTESIAN_POINT('Ctrl Pts',(1.38952890043916,43.9780537249529,15.));
#28495=CARTESIAN_POINT('Ctrl Pts',(12.2684454652018,42.2550026135057,0.));
#28496=CARTESIAN_POINT('Ctrl Pts',(12.2684454652018,42.2550026135057,18.));
#28497=CARTESIAN_POINT('Ctrl Pts',(12.2530833383985,42.2409327400055,0.));
#28498=CARTESIAN_POINT('Ctrl Pts',(12.2530833383985,42.2409327400055,18.));
#28499=CARTESIAN_POINT('Ctrl Pts',(12.222401466668,42.2127669677092,0.));
#28500=CARTESIAN_POINT('Ctrl Pts',(12.222401466668,42.2127669677092,18.));
#28501=CARTESIAN_POINT('Ctrl Pts',(12.1765058047069,42.1704402333854,0.));
#28502=CARTESIAN_POINT('Ctrl Pts',(12.1765058047069,42.1704402333854,18.));
#28503=CARTESIAN_POINT('Ctrl Pts',(12.1155659644537,42.1138483839101,0.));
#28504=CARTESIAN_POINT('Ctrl Pts',(12.1155659644537,42.1138483839101,18.));
#28505=CARTESIAN_POINT('Ctrl Pts',(12.0398158079102,42.0428479428228,0.));
#28506=CARTESIAN_POINT('Ctrl Pts',(12.0398158079102,42.0428479428228,18.));
#28507=CARTESIAN_POINT('Ctrl Pts',(11.9644914999263,41.9715865222182,0.));
#28508=CARTESIAN_POINT('Ctrl Pts',(11.9644914999263,41.9715865222182,18.));
#28509=CARTESIAN_POINT('Ctrl Pts',(11.8895948153349,41.9000638152266,0.));
#28510=CARTESIAN_POINT('Ctrl Pts',(11.8895948153349,41.9000638152266,18.));
#28511=CARTESIAN_POINT('Ctrl Pts',(11.81512813804,41.8282796562569,0.));
#28512=CARTESIAN_POINT('Ctrl Pts',(11.81512813804,41.8282796562569,18.));
#28513=CARTESIAN_POINT('Ctrl Pts',(11.7410945211992,41.7562341395977,0.));
#28514=CARTESIAN_POINT('Ctrl Pts',(11.7410945211992,41.7562341395977,18.));
#28515=CARTESIAN_POINT('Ctrl Pts',(11.6674975352852,41.6839275596248,0.));
#28516=CARTESIAN_POINT('Ctrl Pts',(11.6674975352852,41.6839275596248,18.));
#28517=CARTESIAN_POINT('Ctrl Pts',(11.5943410868252,41.6113603270596,0.));
#28518=CARTESIAN_POINT('Ctrl Pts',(11.5943410868252,41.6113603270596,18.));
#28519=CARTESIAN_POINT('Ctrl Pts',(11.5216292382388,41.5385328935506,0.));
#28520=CARTESIAN_POINT('Ctrl Pts',(11.5216292382388,41.5385328935506,18.));
#28521=CARTESIAN_POINT('Ctrl Pts',(11.4493660393849,41.4654456796071,0.));
#28522=CARTESIAN_POINT('Ctrl Pts',(11.4493660393849,41.4654456796071,18.));
#28523=CARTESIAN_POINT('Ctrl Pts',(11.3775553120176,41.3920989905986,0.));
#28524=CARTESIAN_POINT('Ctrl Pts',(11.3775553120176,41.3920989905986,18.));
#28525=CARTESIAN_POINT('Ctrl Pts',(11.3062006993745,41.3184930194148,0.));
#28526=CARTESIAN_POINT('Ctrl Pts',(11.3062006993745,41.3184930194148,18.));
#28527=CARTESIAN_POINT('Ctrl Pts',(11.2353057980338,41.2446278781981,0.));
#28528=CARTESIAN_POINT('Ctrl Pts',(11.2353057980338,41.2446278781981,18.));
#28529=CARTESIAN_POINT('Ctrl Pts',(11.1648742640378,41.1705036228854,0.));
#28530=CARTESIAN_POINT('Ctrl Pts',(11.1648742640378,41.1705036228854,18.));
#28531=CARTESIAN_POINT('Ctrl Pts',(11.0949099155251,41.0961202807715,0.));
#28532=CARTESIAN_POINT('Ctrl Pts',(11.0949099155251,41.0961202807715,18.));
#28533=CARTESIAN_POINT('Ctrl Pts',(11.0254168609972,41.0214778832142,0.));
#28534=CARTESIAN_POINT('Ctrl Pts',(11.0254168609972,41.0214778832142,18.));
#28535=CARTESIAN_POINT('Ctrl Pts',(10.956399476781,40.9465764747798,0.));
#28536=CARTESIAN_POINT('Ctrl Pts',(10.956399476781,40.9465764747798,18.));
#28537=CARTESIAN_POINT('Ctrl Pts',(10.8878623066646,40.8714161092412,0.));
#28538=CARTESIAN_POINT('Ctrl Pts',(10.8878623066646,40.8714161092412,18.));
#28539=CARTESIAN_POINT('Ctrl Pts',(10.8198099757795,40.7959968527561,0.));
#28540=CARTESIAN_POINT('Ctrl Pts',(10.8198099757795,40.7959968527561,18.));
#28541=CARTESIAN_POINT('Ctrl Pts',(10.7522471109694,40.7203187831783,0.));
#28542=CARTESIAN_POINT('Ctrl Pts',(10.7522471109694,40.7203187831783,18.));
#28543=CARTESIAN_POINT('Ctrl Pts',(10.6851782157325,40.6443819999244,0.));
#28544=CARTESIAN_POINT('Ctrl Pts',(10.6851782157325,40.6443819999244,18.));
#28545=CARTESIAN_POINT('Ctrl Pts',(10.618607730849,40.5681866012103,0.));
#28546=CARTESIAN_POINT('Ctrl Pts',(10.618607730849,40.5681866012103,18.));
#28547=CARTESIAN_POINT('Ctrl Pts',(10.5525402237951,40.4917326404439,0.));
#28548=CARTESIAN_POINT('Ctrl Pts',(10.5525402237951,40.4917326404439,18.));
#28549=CARTESIAN_POINT('Ctrl Pts',(10.48698054978,40.4150200869536,0.));
#28550=CARTESIAN_POINT('Ctrl Pts',(10.48698054978,40.4150200869536,18.));
#28551=CARTESIAN_POINT('Ctrl Pts',(10.4219339932951,40.3380487942952,0.));
#28552=CARTESIAN_POINT('Ctrl Pts',(10.4219339932951,40.3380487942952,18.));
#28553=CARTESIAN_POINT('Ctrl Pts',(10.3574064830678,40.2608184485326,0.));
#28554=CARTESIAN_POINT('Ctrl Pts',(10.3574064830678,40.2608184485326,18.));
#28555=CARTESIAN_POINT('Ctrl Pts',(10.2934044990237,40.1833286010098,0.));
#28556=CARTESIAN_POINT('Ctrl Pts',(10.2934044990237,40.1833286010098,18.));
#28557=CARTESIAN_POINT('Ctrl Pts',(10.2299347125857,40.1055787732578,0.));
#28558=CARTESIAN_POINT('Ctrl Pts',(10.2299347125857,40.1055787732578,18.));
#28559=CARTESIAN_POINT('Ctrl Pts',(10.1670036683795,40.0275685525923,0.));
#28560=CARTESIAN_POINT('Ctrl Pts',(10.1670036683795,40.0275685525923,18.));
#28561=CARTESIAN_POINT('Ctrl Pts',(10.1046175096878,39.9492976736738,0.));
#28562=CARTESIAN_POINT('Ctrl Pts',(10.1046175096878,39.9492976736738,18.));
#28563=CARTESIAN_POINT('Ctrl Pts',(10.0427815229883,39.8707661565233,0.));
#28564=CARTESIAN_POINT('Ctrl Pts',(10.0427815229883,39.8707661565233,18.));
#28565=CARTESIAN_POINT('Ctrl Pts',(9.98150036150824,39.7919742367922,0.));
#28566=CARTESIAN_POINT('Ctrl Pts',(9.98150036150824,39.7919742367922,18.));
#28567=CARTESIAN_POINT('Ctrl Pts',(9.92077894513192,39.712922089547,0.));
#28568=CARTESIAN_POINT('Ctrl Pts',(9.92077894513192,39.712922089547,18.));
#28569=CARTESIAN_POINT('Ctrl Pts',(9.8606232424256,39.6336095893767,0.));
#28570=CARTESIAN_POINT('Ctrl Pts',(9.8606232424256,39.6336095893767,18.));
#28571=CARTESIAN_POINT('Ctrl Pts',(9.80104095251614,39.5540361022309,0.));
#28572=CARTESIAN_POINT('Ctrl Pts',(9.80104095251614,39.5540361022309,18.));
#28573=CARTESIAN_POINT('Ctrl Pts',(9.74204258152664,39.4742001555227,0.));
#28574=CARTESIAN_POINT('Ctrl Pts',(9.74204258152664,39.4742001555227,18.));
#28575=CARTESIAN_POINT('Ctrl Pts',(9.68364100883828,39.3940995760289,0.));
#28576=CARTESIAN_POINT('Ctrl Pts',(9.68364100883828,39.3940995760289,18.));
#28577=CARTESIAN_POINT('Ctrl Pts',(9.62584947846544,39.3137321153686,0.));
#28578=CARTESIAN_POINT('Ctrl Pts',(9.62584947846544,39.3137321153686,18.));
#28579=CARTESIAN_POINT('Ctrl Pts',(9.56867984233624,39.2330959982788,0.));
#28580=CARTESIAN_POINT('Ctrl Pts',(9.56867984233624,39.2330959982788,18.));
#28581=CARTESIAN_POINT('Ctrl Pts',(9.51214104535621,39.1521903958956,0.));
#28582=CARTESIAN_POINT('Ctrl Pts',(9.51214104535621,39.1521903958956,18.));
#28583=CARTESIAN_POINT('Ctrl Pts',(9.45623664577432,39.0710161994951,0.));
#28584=CARTESIAN_POINT('Ctrl Pts',(9.45623664577432,39.0710161994951,18.));
#28585=CARTESIAN_POINT('Ctrl Pts',(9.40096600877644,38.9895756526779,0.));
#28586=CARTESIAN_POINT('Ctrl Pts',(9.40096600877644,38.9895756526779,18.));
#28587=CARTESIAN_POINT('Ctrl Pts',(9.34632917154637,38.9078708427078,0.));
#28588=CARTESIAN_POINT('Ctrl Pts',(9.34632917154637,38.9078708427078,18.));
#28589=CARTESIAN_POINT('Ctrl Pts',(9.29233110570903,38.8259023794241,0.));
#28590=CARTESIAN_POINT('Ctrl Pts',(9.29233110570903,38.8259023794241,18.));
#28591=CARTESIAN_POINT('Ctrl Pts',(9.23898539199332,38.7436682576832,0.));
#28592=CARTESIAN_POINT('Ctrl Pts',(9.23898539199332,38.7436682576832,18.));
#28593=CARTESIAN_POINT('Ctrl Pts',(9.1863201939433,38.6611620045193,0.));
#28594=CARTESIAN_POINT('Ctrl Pts',(9.1863201939433,38.6611620045193,18.));
#28595=CARTESIAN_POINT('Ctrl Pts',(9.13437512010586,38.5783736628826,0.));
#28596=CARTESIAN_POINT('Ctrl Pts',(9.13437512010586,38.5783736628826,18.));
#28597=CARTESIAN_POINT('Ctrl Pts',(9.08319014288086,38.4952932486131,0.));
#28598=CARTESIAN_POINT('Ctrl Pts',(9.08319014288086,38.4952932486131,18.));
#28599=CARTESIAN_POINT('Ctrl Pts',(9.03279579360191,38.4119138099805,0.));
#28600=CARTESIAN_POINT('Ctrl Pts',(9.03279579360191,38.4119138099805,18.));
#28601=CARTESIAN_POINT('Ctrl Pts',(8.9832048378576,38.3282340281403,0.));
#28602=CARTESIAN_POINT('Ctrl Pts',(8.9832048378576,38.3282340281403,18.));
#28603=CARTESIAN_POINT('Ctrl Pts',(8.93439830996339,38.2442625706309,0.));
#28604=CARTESIAN_POINT('Ctrl Pts',(8.93439830996339,38.2442625706309,18.));
#28605=CARTESIAN_POINT('Ctrl Pts',(8.88633535238435,38.1600150482528,0.));
#28606=CARTESIAN_POINT('Ctrl Pts',(8.88633535238435,38.1600150482528,18.));
#28607=CARTESIAN_POINT('Ctrl Pts',(8.8389795976335,38.0755058326913,0.));
#28608=CARTESIAN_POINT('Ctrl Pts',(8.8389795976335,38.0755058326913,18.));
#28609=CARTESIAN_POINT('Ctrl Pts',(8.79232279131092,37.9907407304174,0.));
#28610=CARTESIAN_POINT('Ctrl Pts',(8.79232279131092,37.9907407304174,18.));
#28611=CARTESIAN_POINT('Ctrl Pts',(8.74640499479003,37.9057107230066,0.));
#28612=CARTESIAN_POINT('Ctrl Pts',(8.74640499479003,37.9057107230066,18.));
#28613=CARTESIAN_POINT('Ctrl Pts',(8.70134776631144,37.8203816669032,0.));
#28614=CARTESIAN_POINT('Ctrl Pts',(8.70134776631144,37.8203816669032,18.));
#28615=CARTESIAN_POINT('Ctrl Pts',(8.65732553894525,37.7347032383719,0.));
#28616=CARTESIAN_POINT('Ctrl Pts',(8.65732553894525,37.7347032383719,18.));
#28617=CARTESIAN_POINT('Ctrl Pts',(8.61450621749155,37.6486274754754,0.));
#28618=CARTESIAN_POINT('Ctrl Pts',(8.61450621749155,37.6486274754754,18.));
#28619=CARTESIAN_POINT('Ctrl Pts',(8.57299698459466,37.5621256752108,0.));
#28620=CARTESIAN_POINT('Ctrl Pts',(8.57299698459466,37.5621256752108,18.));
#28621=CARTESIAN_POINT('Ctrl Pts',(8.53279758643785,37.4752030152968,0.));
#28622=CARTESIAN_POINT('Ctrl Pts',(8.53279758643785,37.4752030152968,18.));
#28623=CARTESIAN_POINT('Ctrl Pts',(8.49372546467076,37.3879218093514,0.));
#28624=CARTESIAN_POINT('Ctrl Pts',(8.49372546467076,37.3879218093514,18.));
#28625=CARTESIAN_POINT('Ctrl Pts',(8.4555084943396,37.3003733151561,0.));
#28626=CARTESIAN_POINT('Ctrl Pts',(8.4555084943396,37.3003733151561,18.));
#28627=CARTESIAN_POINT('Ctrl Pts',(8.41793088313261,37.2126332013933,0.));
#28628=CARTESIAN_POINT('Ctrl Pts',(8.41793088313261,37.2126332013933,18.));
#28629=CARTESIAN_POINT('Ctrl Pts',(8.38096706211448,37.1247207489179,0.));
#28630=CARTESIAN_POINT('Ctrl Pts',(8.38096706211448,37.1247207489179,18.));
#28631=CARTESIAN_POINT('Ctrl Pts',(8.3449081895264,37.0365602155149,0.));
#28632=CARTESIAN_POINT('Ctrl Pts',(8.3449081895264,37.0365602155149,18.));
#28633=CARTESIAN_POINT('Ctrl Pts',(8.31052547794592,36.9479311729484,0.));
#28634=CARTESIAN_POINT('Ctrl Pts',(8.31052547794592,36.9479311729484,18.));
#28635=CARTESIAN_POINT('Ctrl Pts',(8.27886599440786,36.8585291300917,0.));
#28636=CARTESIAN_POINT('Ctrl Pts',(8.27886599440786,36.8585291300917,18.));
#28637=CARTESIAN_POINT('Ctrl Pts',(8.25656657451821,36.7861403757605,0.));
#28638=CARTESIAN_POINT('Ctrl Pts',(8.25656657451821,36.7861403757605,18.));
#28639=CARTESIAN_POINT('Ctrl Pts',(8.24192165947368,36.7312504697652,0.));
#28640=CARTESIAN_POINT('Ctrl Pts',(8.24192165947368,36.7312504697652,18.));
#28641=CARTESIAN_POINT('Ctrl Pts',(8.23313075335377,36.6943771018148,0.));
#28642=CARTESIAN_POINT('Ctrl Pts',(8.23313075335377,36.6943771018148,18.));
#28643=CARTESIAN_POINT('Ctrl Pts',(8.22897839625062,36.6758703925241,0.));
#28644=CARTESIAN_POINT('Ctrl Pts',(8.22897839625062,36.6758703925241,18.));
#28645=CARTESIAN_POINT('',(12.2684454652017,42.2550026135057,0.));
#28646=CARTESIAN_POINT('Ctrl Pts',(8.22897839625062,36.6758703925241,0.));
#28647=CARTESIAN_POINT('Ctrl Pts',(8.23313075335377,36.6943771018148,0.));
#28648=CARTESIAN_POINT('Ctrl Pts',(8.24192165947368,36.7312504697652,0.));
#28649=CARTESIAN_POINT('Ctrl Pts',(8.25656657451821,36.7861403757605,0.));
#28650=CARTESIAN_POINT('Ctrl Pts',(8.27886599440786,36.8585291300917,0.));
#28651=CARTESIAN_POINT('Ctrl Pts',(8.31052547794592,36.9479311729484,0.));
#28652=CARTESIAN_POINT('Ctrl Pts',(8.3449081895264,37.0365602155149,0.));
#28653=CARTESIAN_POINT('Ctrl Pts',(8.38096706211448,37.1247207489179,0.));
#28654=CARTESIAN_POINT('Ctrl Pts',(8.41793088313261,37.2126332013933,0.));
#28655=CARTESIAN_POINT('Ctrl Pts',(8.4555084943396,37.3003733151561,0.));
#28656=CARTESIAN_POINT('Ctrl Pts',(8.49372546467076,37.3879218093514,0.));
#28657=CARTESIAN_POINT('Ctrl Pts',(8.53279758643785,37.4752030152968,0.));
#28658=CARTESIAN_POINT('Ctrl Pts',(8.57299698459466,37.5621256752108,0.));
#28659=CARTESIAN_POINT('Ctrl Pts',(8.61450621749155,37.6486274754754,0.));
#28660=CARTESIAN_POINT('Ctrl Pts',(8.65732553894525,37.7347032383719,0.));
#28661=CARTESIAN_POINT('Ctrl Pts',(8.70134776631144,37.8203816669032,0.));
#28662=CARTESIAN_POINT('Ctrl Pts',(8.74640499479003,37.9057107230066,0.));
#28663=CARTESIAN_POINT('Ctrl Pts',(8.79232279131092,37.9907407304174,0.));
#28664=CARTESIAN_POINT('Ctrl Pts',(8.8389795976335,38.0755058326913,0.));
#28665=CARTESIAN_POINT('Ctrl Pts',(8.88633535238435,38.1600150482528,0.));
#28666=CARTESIAN_POINT('Ctrl Pts',(8.93439830996339,38.2442625706309,0.));
#28667=CARTESIAN_POINT('Ctrl Pts',(8.9832048378576,38.3282340281403,0.));
#28668=CARTESIAN_POINT('Ctrl Pts',(9.03279579360191,38.4119138099805,0.));
#28669=CARTESIAN_POINT('Ctrl Pts',(9.08319014288086,38.4952932486131,0.));
#28670=CARTESIAN_POINT('Ctrl Pts',(9.13437512010586,38.5783736628826,0.));
#28671=CARTESIAN_POINT('Ctrl Pts',(9.1863201939433,38.6611620045193,0.));
#28672=CARTESIAN_POINT('Ctrl Pts',(9.23898539199332,38.7436682576832,0.));
#28673=CARTESIAN_POINT('Ctrl Pts',(9.29233110570903,38.8259023794241,0.));
#28674=CARTESIAN_POINT('Ctrl Pts',(9.34632917154637,38.9078708427078,0.));
#28675=CARTESIAN_POINT('Ctrl Pts',(9.40096600877644,38.9895756526779,0.));
#28676=CARTESIAN_POINT('Ctrl Pts',(9.45623664577432,39.0710161994951,0.));
#28677=CARTESIAN_POINT('Ctrl Pts',(9.51214104535621,39.1521903958956,0.));
#28678=CARTESIAN_POINT('Ctrl Pts',(9.56867984233624,39.2330959982788,0.));
#28679=CARTESIAN_POINT('Ctrl Pts',(9.62584947846544,39.3137321153686,0.));
#28680=CARTESIAN_POINT('Ctrl Pts',(9.68364100883828,39.3940995760289,0.));
#28681=CARTESIAN_POINT('Ctrl Pts',(9.74204258152664,39.4742001555227,0.));
#28682=CARTESIAN_POINT('Ctrl Pts',(9.80104095251614,39.5540361022309,0.));
#28683=CARTESIAN_POINT('Ctrl Pts',(9.8606232424256,39.6336095893767,0.));
#28684=CARTESIAN_POINT('Ctrl Pts',(9.92077894513192,39.712922089547,0.));
#28685=CARTESIAN_POINT('Ctrl Pts',(9.98150036150824,39.7919742367922,0.));
#28686=CARTESIAN_POINT('Ctrl Pts',(10.0427815229883,39.8707661565233,0.));
#28687=CARTESIAN_POINT('Ctrl Pts',(10.1046175096878,39.9492976736738,0.));
#28688=CARTESIAN_POINT('Ctrl Pts',(10.1670036683795,40.0275685525923,0.));
#28689=CARTESIAN_POINT('Ctrl Pts',(10.2299347125857,40.1055787732578,0.));
#28690=CARTESIAN_POINT('Ctrl Pts',(10.2934044990237,40.1833286010098,0.));
#28691=CARTESIAN_POINT('Ctrl Pts',(10.3574064830678,40.2608184485326,0.));
#28692=CARTESIAN_POINT('Ctrl Pts',(10.4219339932951,40.3380487942952,0.));
#28693=CARTESIAN_POINT('Ctrl Pts',(10.48698054978,40.4150200869536,0.));
#28694=CARTESIAN_POINT('Ctrl Pts',(10.5525402237951,40.4917326404439,0.));
#28695=CARTESIAN_POINT('Ctrl Pts',(10.618607730849,40.5681866012103,0.));
#28696=CARTESIAN_POINT('Ctrl Pts',(10.6851782157325,40.6443819999244,0.));
#28697=CARTESIAN_POINT('Ctrl Pts',(10.7522471109694,40.7203187831783,0.));
#28698=CARTESIAN_POINT('Ctrl Pts',(10.8198099757795,40.7959968527561,0.));
#28699=CARTESIAN_POINT('Ctrl Pts',(10.8878623066646,40.8714161092412,0.));
#28700=CARTESIAN_POINT('Ctrl Pts',(10.956399476781,40.9465764747798,0.));
#28701=CARTESIAN_POINT('Ctrl Pts',(11.0254168609972,41.0214778832142,0.));
#28702=CARTESIAN_POINT('Ctrl Pts',(11.0949099155251,41.0961202807715,0.));
#28703=CARTESIAN_POINT('Ctrl Pts',(11.1648742640378,41.1705036228854,0.));
#28704=CARTESIAN_POINT('Ctrl Pts',(11.2353057980338,41.2446278781981,0.));
#28705=CARTESIAN_POINT('Ctrl Pts',(11.3062006993745,41.3184930194148,0.));
#28706=CARTESIAN_POINT('Ctrl Pts',(11.3775553120176,41.3920989905986,0.));
#28707=CARTESIAN_POINT('Ctrl Pts',(11.4493660393849,41.4654456796071,0.));
#28708=CARTESIAN_POINT('Ctrl Pts',(11.5216292382388,41.5385328935506,0.));
#28709=CARTESIAN_POINT('Ctrl Pts',(11.5943410868252,41.6113603270596,0.));
#28710=CARTESIAN_POINT('Ctrl Pts',(11.6674975352852,41.6839275596248,0.));
#28711=CARTESIAN_POINT('Ctrl Pts',(11.7410945211992,41.7562341395977,0.));
#28712=CARTESIAN_POINT('Ctrl Pts',(11.81512813804,41.8282796562569,0.));
#28713=CARTESIAN_POINT('Ctrl Pts',(11.8895948153349,41.9000638152266,0.));
#28714=CARTESIAN_POINT('Ctrl Pts',(11.9644914999263,41.9715865222182,0.));
#28715=CARTESIAN_POINT('Ctrl Pts',(12.054880669507,42.0571002269437,0.));
#28716=CARTESIAN_POINT('Ctrl Pts',(12.1307372881904,42.1280354231517,0.));
#28717=CARTESIAN_POINT('Ctrl Pts',(12.1917619768791,42.18457517013,0.));
#28718=CARTESIAN_POINT('Ctrl Pts',(12.2377212115625,42.2268628664988,0.));
#28719=CARTESIAN_POINT('Ctrl Pts',(12.2684454652018,42.2550026135057,0.));
#28720=CARTESIAN_POINT('',(12.2684454652017,42.2550026135057,15.));
#28721=CARTESIAN_POINT('Ctrl Pts',(12.2684454652018,42.2550026135057,15.));
#28722=CARTESIAN_POINT('Ctrl Pts',(12.2530833383985,42.2409327400055,15.));
#28723=CARTESIAN_POINT('Ctrl Pts',(12.222401466668,42.2127669677092,15.));
#28724=CARTESIAN_POINT('Ctrl Pts',(12.1765058047069,42.1704402333854,15.));
#28725=CARTESIAN_POINT('Ctrl Pts',(12.1155659644537,42.1138483839101,15.));
#28726=CARTESIAN_POINT('Ctrl Pts',(12.0398158079102,42.0428479428228,15.));
#28727=CARTESIAN_POINT('Ctrl Pts',(11.9644914999263,41.9715865222182,15.));
#28728=CARTESIAN_POINT('Ctrl Pts',(11.8895948153349,41.9000638152266,15.));
#28729=CARTESIAN_POINT('Ctrl Pts',(11.81512813804,41.8282796562569,15.));
#28730=CARTESIAN_POINT('Ctrl Pts',(11.7410945211992,41.7562341395977,15.));
#28731=CARTESIAN_POINT('Ctrl Pts',(11.6674975352852,41.6839275596248,15.));
#28732=CARTESIAN_POINT('Ctrl Pts',(11.5943410868252,41.6113603270596,15.));
#28733=CARTESIAN_POINT('Ctrl Pts',(11.5216292382388,41.5385328935506,15.));
#28734=CARTESIAN_POINT('Ctrl Pts',(11.4493660393849,41.4654456796071,15.));
#28735=CARTESIAN_POINT('Ctrl Pts',(11.3775553120176,41.3920989905986,15.));
#28736=CARTESIAN_POINT('Ctrl Pts',(11.3062006993745,41.3184930194148,15.));
#28737=CARTESIAN_POINT('Ctrl Pts',(11.2353057980338,41.2446278781981,15.));
#28738=CARTESIAN_POINT('Ctrl Pts',(11.1648742640378,41.1705036228854,15.));
#28739=CARTESIAN_POINT('Ctrl Pts',(11.0949099155251,41.0961202807715,15.));
#28740=CARTESIAN_POINT('Ctrl Pts',(11.0254168609972,41.0214778832142,15.));
#28741=CARTESIAN_POINT('Ctrl Pts',(10.956399476781,40.9465764747798,15.));
#28742=CARTESIAN_POINT('Ctrl Pts',(10.8878623066646,40.8714161092412,15.));
#28743=CARTESIAN_POINT('Ctrl Pts',(10.8198099757795,40.7959968527561,15.));
#28744=CARTESIAN_POINT('Ctrl Pts',(10.7522471109694,40.7203187831783,15.));
#28745=CARTESIAN_POINT('Ctrl Pts',(10.6851782157325,40.6443819999244,15.));
#28746=CARTESIAN_POINT('Ctrl Pts',(10.618607730849,40.5681866012103,15.));
#28747=CARTESIAN_POINT('Ctrl Pts',(10.5525402237951,40.4917326404439,15.));
#28748=CARTESIAN_POINT('Ctrl Pts',(10.48698054978,40.4150200869536,15.));
#28749=CARTESIAN_POINT('Ctrl Pts',(10.4219339932951,40.3380487942952,15.));
#28750=CARTESIAN_POINT('Ctrl Pts',(10.3574064830678,40.2608184485326,15.));
#28751=CARTESIAN_POINT('Ctrl Pts',(10.2934044990237,40.1833286010098,15.));
#28752=CARTESIAN_POINT('Ctrl Pts',(10.2299347125857,40.1055787732578,15.));
#28753=CARTESIAN_POINT('Ctrl Pts',(10.1670036683795,40.0275685525923,15.));
#28754=CARTESIAN_POINT('Ctrl Pts',(10.1046175096878,39.9492976736738,15.));
#28755=CARTESIAN_POINT('Ctrl Pts',(10.0427815229883,39.8707661565233,15.));
#28756=CARTESIAN_POINT('Ctrl Pts',(9.98150036150824,39.7919742367922,15.));
#28757=CARTESIAN_POINT('Ctrl Pts',(9.92077894513192,39.712922089547,15.));
#28758=CARTESIAN_POINT('Ctrl Pts',(9.8606232424256,39.6336095893767,15.));
#28759=CARTESIAN_POINT('Ctrl Pts',(9.80104095251614,39.5540361022309,15.));
#28760=CARTESIAN_POINT('Ctrl Pts',(9.74204258152664,39.4742001555227,15.));
#28761=CARTESIAN_POINT('Ctrl Pts',(9.68364100883828,39.3940995760289,15.));
#28762=CARTESIAN_POINT('Ctrl Pts',(9.62584947846544,39.3137321153686,15.));
#28763=CARTESIAN_POINT('Ctrl Pts',(9.56867984233624,39.2330959982788,15.));
#28764=CARTESIAN_POINT('Ctrl Pts',(9.51214104535621,39.1521903958956,15.));
#28765=CARTESIAN_POINT('Ctrl Pts',(9.45623664577432,39.0710161994951,15.));
#28766=CARTESIAN_POINT('Ctrl Pts',(9.40096600877644,38.9895756526779,15.));
#28767=CARTESIAN_POINT('Ctrl Pts',(9.34632917154637,38.9078708427078,15.));
#28768=CARTESIAN_POINT('Ctrl Pts',(9.29233110570903,38.8259023794241,15.));
#28769=CARTESIAN_POINT('Ctrl Pts',(9.23898539199332,38.7436682576832,15.));
#28770=CARTESIAN_POINT('Ctrl Pts',(9.1863201939433,38.6611620045193,15.));
#28771=CARTESIAN_POINT('Ctrl Pts',(9.13437512010586,38.5783736628826,15.));
#28772=CARTESIAN_POINT('Ctrl Pts',(9.08319014288086,38.4952932486131,15.));
#28773=CARTESIAN_POINT('Ctrl Pts',(9.03279579360191,38.4119138099805,15.));
#28774=CARTESIAN_POINT('Ctrl Pts',(8.9832048378576,38.3282340281403,15.));
#28775=CARTESIAN_POINT('Ctrl Pts',(8.93439830996339,38.2442625706309,15.));
#28776=CARTESIAN_POINT('Ctrl Pts',(8.88633535238435,38.1600150482528,15.));
#28777=CARTESIAN_POINT('Ctrl Pts',(8.8389795976335,38.0755058326913,15.));
#28778=CARTESIAN_POINT('Ctrl Pts',(8.79232279131092,37.9907407304174,15.));
#28779=CARTESIAN_POINT('Ctrl Pts',(8.74640499479003,37.9057107230066,15.));
#28780=CARTESIAN_POINT('Ctrl Pts',(8.70134776631144,37.8203816669032,15.));
#28781=CARTESIAN_POINT('Ctrl Pts',(8.65732553894525,37.7347032383719,15.));
#28782=CARTESIAN_POINT('Ctrl Pts',(8.61450621749155,37.6486274754754,15.));
#28783=CARTESIAN_POINT('Ctrl Pts',(8.57299698459466,37.5621256752108,15.));
#28784=CARTESIAN_POINT('Ctrl Pts',(8.53279758643785,37.4752030152968,15.));
#28785=CARTESIAN_POINT('Ctrl Pts',(8.49372546467076,37.3879218093514,15.));
#28786=CARTESIAN_POINT('Ctrl Pts',(8.4555084943396,37.3003733151561,15.));
#28787=CARTESIAN_POINT('Ctrl Pts',(8.41793088313261,37.2126332013933,15.));
#28788=CARTESIAN_POINT('Ctrl Pts',(8.38096706211448,37.1247207489179,15.));
#28789=CARTESIAN_POINT('Ctrl Pts',(8.3449081895264,37.0365602155149,15.));
#28790=CARTESIAN_POINT('Ctrl Pts',(8.31052547794592,36.9479311729484,15.));
#28791=CARTESIAN_POINT('Ctrl Pts',(8.27886599440786,36.8585291300917,15.));
#28792=CARTESIAN_POINT('Ctrl Pts',(8.25656657451821,36.7861403757605,15.));
#28793=CARTESIAN_POINT('Ctrl Pts',(8.24192165947368,36.7312504697652,15.));
#28794=CARTESIAN_POINT('Ctrl Pts',(8.23313075335377,36.6943771018148,15.));
#28795=CARTESIAN_POINT('Ctrl Pts',(8.22897839625062,36.6758703925241,15.));
#28796=CARTESIAN_POINT('',(12.2684454652017,42.2550026135057,0.));
#28797=CARTESIAN_POINT('Origin',(3.50213800024364E-12,1.07784724682657E-11,
0.));
#28798=CARTESIAN_POINT('',(14.911486495888,41.396226524684,0.));
#28799=CARTESIAN_POINT('Origin',(3.50213800024364E-12,1.07784724682657E-11,
0.));
#28800=CARTESIAN_POINT('',(14.911486495888,41.396226524684,15.));
#28801=CARTESIAN_POINT('Origin',(3.50213800024364E-12,1.07784724682657E-11,
15.));
#28802=CARTESIAN_POINT('',(14.911486495888,41.396226524684,0.));
#28803=CARTESIAN_POINT('Ctrl Pts',(14.9001523628048,34.5082745737944,0.));
#28804=CARTESIAN_POINT('Ctrl Pts',(14.9001523628048,34.5082745737944,18.));
#28805=CARTESIAN_POINT('Ctrl Pts',(14.9076710061311,34.525687510388,0.));
#28806=CARTESIAN_POINT('Ctrl Pts',(14.9076710061311,34.525687510388,18.));
#28807=CARTESIAN_POINT('Ctrl Pts',(14.9222326355678,34.5606858566713,0.));
#28808=CARTESIAN_POINT('Ctrl Pts',(14.9222326355678,34.5606858566713,18.));
#28809=CARTESIAN_POINT('Ctrl Pts',(14.9426481276593,34.6137007885254,0.));
#28810=CARTESIAN_POINT('Ctrl Pts',(14.9426481276593,34.6137007885254,18.));
#28811=CARTESIAN_POINT('Ctrl Pts',(14.9671565602316,34.6853717911269,0.));
#28812=CARTESIAN_POINT('Ctrl Pts',(14.9671565602316,34.6853717911269,18.));
#28813=CARTESIAN_POINT('Ctrl Pts',(14.9940927023322,34.7763085406486,0.));
#28814=CARTESIAN_POINT('Ctrl Pts',(14.9940927023322,34.7763085406486,18.));
#28815=CARTESIAN_POINT('Ctrl Pts',(15.0183713484962,34.8682205930809,0.));
#28816=CARTESIAN_POINT('Ctrl Pts',(15.0183713484962,34.8682205930809,18.));
#28817=CARTESIAN_POINT('Ctrl Pts',(15.041018569143,34.9607388363587,0.));
#28818=CARTESIAN_POINT('Ctrl Pts',(15.041018569143,34.9607388363587,18.));
#28819=CARTESIAN_POINT('Ctrl Pts',(15.0627878528202,35.0535882932913,0.));
#28820=CARTESIAN_POINT('Ctrl Pts',(15.0627878528202,35.0535882932913,18.));
#28821=CARTESIAN_POINT('Ctrl Pts',(15.08395927165,35.1466591020976,0.));
#28822=CARTESIAN_POINT('Ctrl Pts',(15.08395927165,35.1466591020976,18.));
#28823=CARTESIAN_POINT('Ctrl Pts',(15.104500806927,35.2399506932815,0.));
#28824=CARTESIAN_POINT('Ctrl Pts',(15.104500806927,35.2399506932815,18.));
#28825=CARTESIAN_POINT('Ctrl Pts',(15.1241934020682,35.3335286891314,0.));
#28826=CARTESIAN_POINT('Ctrl Pts',(15.1241934020682,35.3335286891314,18.));
#28827=CARTESIAN_POINT('Ctrl Pts',(15.1427632633831,35.4274792115857,0.));
#28828=CARTESIAN_POINT('Ctrl Pts',(15.1427632633831,35.4274792115857,18.));
#28829=CARTESIAN_POINT('Ctrl Pts',(15.1600260710384,35.5218591529746,0.));
#28830=CARTESIAN_POINT('Ctrl Pts',(15.1600260710384,35.5218591529746,18.));
#28831=CARTESIAN_POINT('Ctrl Pts',(15.1759785763051,35.6166644736253,0.));
#28832=CARTESIAN_POINT('Ctrl Pts',(15.1759785763051,35.6166644736253,18.));
#28833=CARTESIAN_POINT('Ctrl Pts',(15.1907243629659,35.7118553943773,0.));
#28834=CARTESIAN_POINT('Ctrl Pts',(15.1907243629659,35.7118553943773,18.));
#28835=CARTESIAN_POINT('Ctrl Pts',(15.2044274601769,35.8073720252878,0.));
#28836=CARTESIAN_POINT('Ctrl Pts',(15.2044274601769,35.8073720252878,18.));
#28837=CARTESIAN_POINT('Ctrl Pts',(15.2172585668056,35.9031525499277,0.));
#28838=CARTESIAN_POINT('Ctrl Pts',(15.2172585668056,35.9031525499277,18.));
#28839=CARTESIAN_POINT('Ctrl Pts',(15.2293360946131,35.9991531408727,0.));
#28840=CARTESIAN_POINT('Ctrl Pts',(15.2293360946131,35.9991531408727,18.));
#28841=CARTESIAN_POINT('Ctrl Pts',(15.240697754828,36.095357546697,0.));
#28842=CARTESIAN_POINT('Ctrl Pts',(15.240697754828,36.095357546697,18.));
#28843=CARTESIAN_POINT('Ctrl Pts',(15.2513334565427,36.1917659216814,0.));
#28844=CARTESIAN_POINT('Ctrl Pts',(15.2513334565427,36.1917659216814,18.));
#28845=CARTESIAN_POINT('Ctrl Pts',(15.2612053303774,36.2883880151607,0.));
#28846=CARTESIAN_POINT('Ctrl Pts',(15.2612053303774,36.2883880151607,18.));
#28847=CARTESIAN_POINT('Ctrl Pts',(15.2702711460937,36.3852352131887,0.));
#28848=CARTESIAN_POINT('Ctrl Pts',(15.2702711460937,36.3852352131887,18.));
#28849=CARTESIAN_POINT('Ctrl Pts',(15.2785104654792,36.4823116513289,0.));
#28850=CARTESIAN_POINT('Ctrl Pts',(15.2785104654792,36.4823116513289,18.));
#28851=CARTESIAN_POINT('Ctrl Pts',(15.2859343913094,36.5796108931244,0.));
#28852=CARTESIAN_POINT('Ctrl Pts',(15.2859343913094,36.5796108931244,18.));
#28853=CARTESIAN_POINT('Ctrl Pts',(15.2925717100767,36.6771206167756,0.));
#28854=CARTESIAN_POINT('Ctrl Pts',(15.2925717100767,36.6771206167756,18.));
#28855=CARTESIAN_POINT('Ctrl Pts',(15.2984606286737,36.7748254044502,0.));
#28856=CARTESIAN_POINT('Ctrl Pts',(15.2984606286737,36.7748254044502,18.));
#28857=CARTESIAN_POINT('Ctrl Pts',(15.3036390436952,36.8727100302512,0.));
#28858=CARTESIAN_POINT('Ctrl Pts',(15.3036390436952,36.8727100302512,18.));
#28859=CARTESIAN_POINT('Ctrl Pts',(15.3081335446406,36.970763176802,0.));
#28860=CARTESIAN_POINT('Ctrl Pts',(15.3081335446406,36.970763176802,18.));
#28861=CARTESIAN_POINT('Ctrl Pts',(15.3119562971444,37.0689784837457,0.));
#28862=CARTESIAN_POINT('Ctrl Pts',(15.3119562971444,37.0689784837457,18.));
#28863=CARTESIAN_POINT('Ctrl Pts',(15.3151109648809,37.1673525354642,0.));
#28864=CARTESIAN_POINT('Ctrl Pts',(15.3151109648809,37.1673525354642,18.));
#28865=CARTESIAN_POINT('Ctrl Pts',(15.3175963510698,37.2658836214694,0.));
#28866=CARTESIAN_POINT('Ctrl Pts',(15.3175963510698,37.2658836214694,18.));
#28867=CARTESIAN_POINT('Ctrl Pts',(15.3194106233801,37.3645702997848,0.));
#28868=CARTESIAN_POINT('Ctrl Pts',(15.3194106233801,37.3645702997848,18.));
#28869=CARTESIAN_POINT('Ctrl Pts',(15.3205561366169,37.4634097578665,0.));
#28870=CARTESIAN_POINT('Ctrl Pts',(15.3205561366169,37.4634097578665,18.));
#28871=CARTESIAN_POINT('Ctrl Pts',(15.3210406145546,37.562397408596,0.));
#28872=CARTESIAN_POINT('Ctrl Pts',(15.3210406145546,37.562397408596,18.));
#28873=CARTESIAN_POINT('Ctrl Pts',(15.3208746890781,37.6615277218027,0.));
#28874=CARTESIAN_POINT('Ctrl Pts',(15.3208746890781,37.6615277218027,18.));
#28875=CARTESIAN_POINT('Ctrl Pts',(15.320070396385,37.7607947318286,0.));
#28876=CARTESIAN_POINT('Ctrl Pts',(15.320070396385,37.7607947318286,18.));
#28877=CARTESIAN_POINT('Ctrl Pts',(15.3186394335023,37.8601926265378,0.));
#28878=CARTESIAN_POINT('Ctrl Pts',(15.3186394335023,37.8601926265378,18.));
#28879=CARTESIAN_POINT('Ctrl Pts',(15.3165911656268,37.959716421934,0.));
#28880=CARTESIAN_POINT('Ctrl Pts',(15.3165911656268,37.959716421934,18.));
#28881=CARTESIAN_POINT('Ctrl Pts',(15.3139321941687,38.0593621055415,0.));
#28882=CARTESIAN_POINT('Ctrl Pts',(15.3139321941687,38.0593621055415,18.));
#28883=CARTESIAN_POINT('Ctrl Pts',(15.310667421514,38.1591262705847,0.));
#28884=CARTESIAN_POINT('Ctrl Pts',(15.310667421514,38.1591262705847,18.));
#28885=CARTESIAN_POINT('Ctrl Pts',(15.3068007250314,38.2590058835965,0.));
#28886=CARTESIAN_POINT('Ctrl Pts',(15.3068007250314,38.2590058835965,18.));
#28887=CARTESIAN_POINT('Ctrl Pts',(15.3023357307483,38.3589980188324,0.));
#28888=CARTESIAN_POINT('Ctrl Pts',(15.3023357307483,38.3589980188324,18.));
#28889=CARTESIAN_POINT('Ctrl Pts',(15.297276703747,38.4590995527814,0.));
#28890=CARTESIAN_POINT('Ctrl Pts',(15.297276703747,38.4590995527814,18.));
#28891=CARTESIAN_POINT('Ctrl Pts',(15.2916287700102,38.5593070891769,0.));
#28892=CARTESIAN_POINT('Ctrl Pts',(15.2916287700102,38.5593070891769,18.));
#28893=CARTESIAN_POINT('Ctrl Pts',(15.2853974668211,38.659617115053,0.));
#28894=CARTESIAN_POINT('Ctrl Pts',(15.2853974668211,38.659617115053,18.));
#28895=CARTESIAN_POINT('Ctrl Pts',(15.2785884727112,38.7600260961351,0.));
#28896=CARTESIAN_POINT('Ctrl Pts',(15.2785884727112,38.7600260961351,18.));
#28897=CARTESIAN_POINT('Ctrl Pts',(15.2712072937639,38.860530586589,0.));
#28898=CARTESIAN_POINT('Ctrl Pts',(15.2712072937639,38.860530586589,18.));
#28899=CARTESIAN_POINT('Ctrl Pts',(15.2632589109473,38.9611273555758,0.));
#28900=CARTESIAN_POINT('Ctrl Pts',(15.2632589109473,38.9611273555758,18.));
#28901=CARTESIAN_POINT('Ctrl Pts',(15.2547476855825,39.061813415425,0.));
#28902=CARTESIAN_POINT('Ctrl Pts',(15.2547476855825,39.061813415425,18.));
#28903=CARTESIAN_POINT('Ctrl Pts',(15.2456775636447,39.1625859371304,0.));
#28904=CARTESIAN_POINT('Ctrl Pts',(15.2456775636447,39.1625859371304,18.));
#28905=CARTESIAN_POINT('Ctrl Pts',(15.2360522089072,39.2634421927888,0.));
#28906=CARTESIAN_POINT('Ctrl Pts',(15.2360522089072,39.2634421927888,18.));
#28907=CARTESIAN_POINT('Ctrl Pts',(15.225875156307,39.3643794927167,0.));
#28908=CARTESIAN_POINT('Ctrl Pts',(15.225875156307,39.3643794927167,18.));
#28909=CARTESIAN_POINT('Ctrl Pts',(15.2151499908149,39.4653951093947,0.));
#28910=CARTESIAN_POINT('Ctrl Pts',(15.2151499908149,39.4653951093947,18.));
#28911=CARTESIAN_POINT('Ctrl Pts',(15.2038804098649,39.5664862602472,0.));
#28912=CARTESIAN_POINT('Ctrl Pts',(15.2038804098649,39.5664862602472,18.));
#28913=CARTESIAN_POINT('Ctrl Pts',(15.1920701163804,39.6676501731673,0.));
#28914=CARTESIAN_POINT('Ctrl Pts',(15.1920701163804,39.6676501731673,18.));
#28915=CARTESIAN_POINT('Ctrl Pts',(15.1797227547562,39.7688841338802,0.));
#28916=CARTESIAN_POINT('Ctrl Pts',(15.1797227547562,39.7688841338802,18.));
#28917=CARTESIAN_POINT('Ctrl Pts',(15.1668418393198,39.8701855339908,0.));
#28918=CARTESIAN_POINT('Ctrl Pts',(15.1668418393198,39.8701855339908,18.));
#28919=CARTESIAN_POINT('Ctrl Pts',(15.1534306754871,39.9715519332134,0.));
#28920=CARTESIAN_POINT('Ctrl Pts',(15.1534306754871,39.9715519332134,18.));
#28921=CARTESIAN_POINT('Ctrl Pts',(15.1394923361537,40.0729810652204,0.));
#28922=CARTESIAN_POINT('Ctrl Pts',(15.1394923361537,40.0729810652204,18.));
#28923=CARTESIAN_POINT('Ctrl Pts',(15.1250297462408,40.1744707357902,0.));
#28924=CARTESIAN_POINT('Ctrl Pts',(15.1250297462408,40.1744707357902,18.));
#28925=CARTESIAN_POINT('Ctrl Pts',(15.1100457495259,40.2760187401822,0.));
#28926=CARTESIAN_POINT('Ctrl Pts',(15.1100457495259,40.2760187401822,18.));
#28927=CARTESIAN_POINT('Ctrl Pts',(15.0945431800724,40.3776227809037,0.));
#28928=CARTESIAN_POINT('Ctrl Pts',(15.0945431800724,40.3776227809037,18.));
#28929=CARTESIAN_POINT('Ctrl Pts',(15.0785249502524,40.4792803645352,0.));
#28930=CARTESIAN_POINT('Ctrl Pts',(15.0785249502524,40.4792803645352,18.));
#28931=CARTESIAN_POINT('Ctrl Pts',(15.0619940893017,40.5809887704301,0.));
#28932=CARTESIAN_POINT('Ctrl Pts',(15.0619940893017,40.5809887704301,18.));
#28933=CARTESIAN_POINT('Ctrl Pts',(15.0449536183143,40.6827452453667,0.));
#28934=CARTESIAN_POINT('Ctrl Pts',(15.0449536183143,40.6827452453667,18.));
#28935=CARTESIAN_POINT('Ctrl Pts',(15.0274064563211,40.7845471608654,0.));
#28936=CARTESIAN_POINT('Ctrl Pts',(15.0274064563211,40.7845471608654,18.));
#28937=CARTESIAN_POINT('Ctrl Pts',(15.0093553188655,40.8863921801,0.));
#28938=CARTESIAN_POINT('Ctrl Pts',(15.0093553188655,40.8863921801,18.));
#28939=CARTESIAN_POINT('Ctrl Pts',(14.9908026205824,40.9882784321884,0.));
#28940=CARTESIAN_POINT('Ctrl Pts',(14.9908026205824,40.9882784321884,18.));
#28941=CARTESIAN_POINT('Ctrl Pts',(14.9717503874227,41.0902046498729,0.));
#28942=CARTESIAN_POINT('Ctrl Pts',(14.9717503874227,41.0902046498729,18.));
#28943=CARTESIAN_POINT('Ctrl Pts',(14.9522002356298,41.1921700381957,0.));
#28944=CARTESIAN_POINT('Ctrl Pts',(14.9522002356298,41.1921700381957,18.));
#28945=CARTESIAN_POINT('Ctrl Pts',(14.936162723752,41.2737733455422,0.));
#28946=CARTESIAN_POINT('Ctrl Pts',(14.936162723752,41.2737733455422,18.));
#28947=CARTESIAN_POINT('Ctrl Pts',(14.9239113834707,41.3349931861715,0.));
#28948=CARTESIAN_POINT('Ctrl Pts',(14.9239113834707,41.3349931861715,18.));
#28949=CARTESIAN_POINT('Ctrl Pts',(14.9156446533966,41.3758141263348,0.));
#28950=CARTESIAN_POINT('Ctrl Pts',(14.9156446533966,41.3758141263348,18.));
#28951=CARTESIAN_POINT('Ctrl Pts',(14.911486495888,41.396226524684,0.));
#28952=CARTESIAN_POINT('Ctrl Pts',(14.911486495888,41.396226524684,18.));
#28953=CARTESIAN_POINT('Ctrl Pts',(14.9001523628048,34.5082745737944,0.));
#28954=CARTESIAN_POINT('Ctrl Pts',(14.9076710061311,34.525687510388,0.));
#28955=CARTESIAN_POINT('Ctrl Pts',(14.9222326355678,34.5606858566713,0.));
#28956=CARTESIAN_POINT('Ctrl Pts',(14.9426481276593,34.6137007885254,0.));
#28957=CARTESIAN_POINT('Ctrl Pts',(14.9671565602316,34.6853717911269,0.));
#28958=CARTESIAN_POINT('Ctrl Pts',(14.9940927023322,34.7763085406486,0.));
#28959=CARTESIAN_POINT('Ctrl Pts',(15.0183713484962,34.8682205930809,0.));
#28960=CARTESIAN_POINT('Ctrl Pts',(15.041018569143,34.9607388363587,0.));
#28961=CARTESIAN_POINT('Ctrl Pts',(15.0627878528202,35.0535882932913,0.));
#28962=CARTESIAN_POINT('Ctrl Pts',(15.08395927165,35.1466591020976,0.));
#28963=CARTESIAN_POINT('Ctrl Pts',(15.104500806927,35.2399506932815,0.));
#28964=CARTESIAN_POINT('Ctrl Pts',(15.1241934020682,35.3335286891314,0.));
#28965=CARTESIAN_POINT('Ctrl Pts',(15.1427632633831,35.4274792115857,0.));
#28966=CARTESIAN_POINT('Ctrl Pts',(15.1600260710384,35.5218591529746,0.));
#28967=CARTESIAN_POINT('Ctrl Pts',(15.1759785763051,35.6166644736253,0.));
#28968=CARTESIAN_POINT('Ctrl Pts',(15.1907243629659,35.7118553943773,0.));
#28969=CARTESIAN_POINT('Ctrl Pts',(15.2044274601769,35.8073720252878,0.));
#28970=CARTESIAN_POINT('Ctrl Pts',(15.2172585668056,35.9031525499277,0.));
#28971=CARTESIAN_POINT('Ctrl Pts',(15.2293360946131,35.9991531408727,0.));
#28972=CARTESIAN_POINT('Ctrl Pts',(15.240697754828,36.095357546697,0.));
#28973=CARTESIAN_POINT('Ctrl Pts',(15.2513334565427,36.1917659216814,0.));
#28974=CARTESIAN_POINT('Ctrl Pts',(15.2612053303774,36.2883880151607,0.));
#28975=CARTESIAN_POINT('Ctrl Pts',(15.2702711460937,36.3852352131887,0.));
#28976=CARTESIAN_POINT('Ctrl Pts',(15.2785104654792,36.4823116513289,0.));
#28977=CARTESIAN_POINT('Ctrl Pts',(15.2859343913094,36.5796108931244,0.));
#28978=CARTESIAN_POINT('Ctrl Pts',(15.2925717100767,36.6771206167756,0.));
#28979=CARTESIAN_POINT('Ctrl Pts',(15.2984606286737,36.7748254044502,0.));
#28980=CARTESIAN_POINT('Ctrl Pts',(15.3036390436952,36.8727100302512,0.));
#28981=CARTESIAN_POINT('Ctrl Pts',(15.3081335446406,36.970763176802,0.));
#28982=CARTESIAN_POINT('Ctrl Pts',(15.3119562971444,37.0689784837457,0.));
#28983=CARTESIAN_POINT('Ctrl Pts',(15.3151109648809,37.1673525354642,0.));
#28984=CARTESIAN_POINT('Ctrl Pts',(15.3175963510698,37.2658836214694,0.));
#28985=CARTESIAN_POINT('Ctrl Pts',(15.3194106233801,37.3645702997848,0.));
#28986=CARTESIAN_POINT('Ctrl Pts',(15.3205561366169,37.4634097578665,0.));
#28987=CARTESIAN_POINT('Ctrl Pts',(15.3210406145546,37.562397408596,0.));
#28988=CARTESIAN_POINT('Ctrl Pts',(15.3208746890781,37.6615277218027,0.));
#28989=CARTESIAN_POINT('Ctrl Pts',(15.320070396385,37.7607947318286,0.));
#28990=CARTESIAN_POINT('Ctrl Pts',(15.3186394335023,37.8601926265378,0.));
#28991=CARTESIAN_POINT('Ctrl Pts',(15.3165911656268,37.959716421934,0.));
#28992=CARTESIAN_POINT('Ctrl Pts',(15.3139321941687,38.0593621055415,0.));
#28993=CARTESIAN_POINT('Ctrl Pts',(15.310667421514,38.1591262705847,0.));
#28994=CARTESIAN_POINT('Ctrl Pts',(15.3068007250314,38.2590058835965,0.));
#28995=CARTESIAN_POINT('Ctrl Pts',(15.3023357307483,38.3589980188324,0.));
#28996=CARTESIAN_POINT('Ctrl Pts',(15.297276703747,38.4590995527814,0.));
#28997=CARTESIAN_POINT('Ctrl Pts',(15.2916287700102,38.5593070891769,0.));
#28998=CARTESIAN_POINT('Ctrl Pts',(15.2853974668211,38.659617115053,0.));
#28999=CARTESIAN_POINT('Ctrl Pts',(15.2785884727112,38.7600260961351,0.));
#29000=CARTESIAN_POINT('Ctrl Pts',(15.2712072937639,38.860530586589,0.));
#29001=CARTESIAN_POINT('Ctrl Pts',(15.2632589109473,38.9611273555758,0.));
#29002=CARTESIAN_POINT('Ctrl Pts',(15.2547476855825,39.061813415425,0.));
#29003=CARTESIAN_POINT('Ctrl Pts',(15.2456775636447,39.1625859371304,0.));
#29004=CARTESIAN_POINT('Ctrl Pts',(15.2360522089072,39.2634421927888,0.));
#29005=CARTESIAN_POINT('Ctrl Pts',(15.225875156307,39.3643794927167,0.));
#29006=CARTESIAN_POINT('Ctrl Pts',(15.2151499908149,39.4653951093947,0.));
#29007=CARTESIAN_POINT('Ctrl Pts',(15.2038804098649,39.5664862602472,0.));
#29008=CARTESIAN_POINT('Ctrl Pts',(15.1920701163804,39.6676501731673,0.));
#29009=CARTESIAN_POINT('Ctrl Pts',(15.1797227547562,39.7688841338802,0.));
#29010=CARTESIAN_POINT('Ctrl Pts',(15.1668418393198,39.8701855339908,0.));
#29011=CARTESIAN_POINT('Ctrl Pts',(15.1534306754871,39.9715519332134,0.));
#29012=CARTESIAN_POINT('Ctrl Pts',(15.1394923361537,40.0729810652204,0.));
#29013=CARTESIAN_POINT('Ctrl Pts',(15.1250297462408,40.1744707357902,0.));
#29014=CARTESIAN_POINT('Ctrl Pts',(15.1100457495259,40.2760187401822,0.));
#29015=CARTESIAN_POINT('Ctrl Pts',(15.0945431800724,40.3776227809037,0.));
#29016=CARTESIAN_POINT('Ctrl Pts',(15.0785249502524,40.4792803645352,0.));
#29017=CARTESIAN_POINT('Ctrl Pts',(15.0619940893017,40.5809887704301,0.));
#29018=CARTESIAN_POINT('Ctrl Pts',(15.0449536183143,40.6827452453667,0.));
#29019=CARTESIAN_POINT('Ctrl Pts',(15.0274064563211,40.7845471608654,0.));
#29020=CARTESIAN_POINT('Ctrl Pts',(15.0093553188655,40.8863921801,0.));
#29021=CARTESIAN_POINT('Ctrl Pts',(14.9908026205824,40.9882784321884,0.));
#29022=CARTESIAN_POINT('Ctrl Pts',(14.9679399407908,41.1105898934098,0.));
#29023=CARTESIAN_POINT('Ctrl Pts',(14.9482653093396,41.2125650743922,0.));
#29024=CARTESIAN_POINT('Ctrl Pts',(14.9321285285561,41.2941761025922,0.));
#29025=CARTESIAN_POINT('Ctrl Pts',(14.919802810928,41.3554017279611,0.));
#29026=CARTESIAN_POINT('Ctrl Pts',(14.911486495888,41.396226524684,0.));
#29027=CARTESIAN_POINT('Ctrl Pts',(14.9001523628048,34.5082745737944,15.));
#29028=CARTESIAN_POINT('Ctrl Pts',(14.9076710061311,34.525687510388,15.));
#29029=CARTESIAN_POINT('Ctrl Pts',(14.9222326355678,34.5606858566713,15.));
#29030=CARTESIAN_POINT('Ctrl Pts',(14.9426481276593,34.6137007885254,15.));
#29031=CARTESIAN_POINT('Ctrl Pts',(14.9671565602316,34.6853717911269,15.));
#29032=CARTESIAN_POINT('Ctrl Pts',(14.9940927023322,34.7763085406486,15.));
#29033=CARTESIAN_POINT('Ctrl Pts',(15.0183713484962,34.8682205930809,15.));
#29034=CARTESIAN_POINT('Ctrl Pts',(15.041018569143,34.9607388363587,15.));
#29035=CARTESIAN_POINT('Ctrl Pts',(15.0627878528202,35.0535882932913,15.));
#29036=CARTESIAN_POINT('Ctrl Pts',(15.08395927165,35.1466591020976,15.));
#29037=CARTESIAN_POINT('Ctrl Pts',(15.104500806927,35.2399506932815,15.));
#29038=CARTESIAN_POINT('Ctrl Pts',(15.1241934020682,35.3335286891314,15.));
#29039=CARTESIAN_POINT('Ctrl Pts',(15.1427632633831,35.4274792115857,15.));
#29040=CARTESIAN_POINT('Ctrl Pts',(15.1600260710384,35.5218591529746,15.));
#29041=CARTESIAN_POINT('Ctrl Pts',(15.1759785763051,35.6166644736253,15.));
#29042=CARTESIAN_POINT('Ctrl Pts',(15.1907243629659,35.7118553943773,15.));
#29043=CARTESIAN_POINT('Ctrl Pts',(15.2044274601769,35.8073720252878,15.));
#29044=CARTESIAN_POINT('Ctrl Pts',(15.2172585668056,35.9031525499277,15.));
#29045=CARTESIAN_POINT('Ctrl Pts',(15.2293360946131,35.9991531408727,15.));
#29046=CARTESIAN_POINT('Ctrl Pts',(15.240697754828,36.095357546697,15.));
#29047=CARTESIAN_POINT('Ctrl Pts',(15.2513334565427,36.1917659216814,15.));
#29048=CARTESIAN_POINT('Ctrl Pts',(15.2612053303774,36.2883880151607,15.));
#29049=CARTESIAN_POINT('Ctrl Pts',(15.2702711460937,36.3852352131887,15.));
#29050=CARTESIAN_POINT('Ctrl Pts',(15.2785104654792,36.4823116513289,15.));
#29051=CARTESIAN_POINT('Ctrl Pts',(15.2859343913094,36.5796108931244,15.));
#29052=CARTESIAN_POINT('Ctrl Pts',(15.2925717100767,36.6771206167756,15.));
#29053=CARTESIAN_POINT('Ctrl Pts',(15.2984606286737,36.7748254044502,15.));
#29054=CARTESIAN_POINT('Ctrl Pts',(15.3036390436952,36.8727100302512,15.));
#29055=CARTESIAN_POINT('Ctrl Pts',(15.3081335446406,36.970763176802,15.));
#29056=CARTESIAN_POINT('Ctrl Pts',(15.3119562971444,37.0689784837457,15.));
#29057=CARTESIAN_POINT('Ctrl Pts',(15.3151109648809,37.1673525354642,15.));
#29058=CARTESIAN_POINT('Ctrl Pts',(15.3175963510698,37.2658836214694,15.));
#29059=CARTESIAN_POINT('Ctrl Pts',(15.3194106233801,37.3645702997848,15.));
#29060=CARTESIAN_POINT('Ctrl Pts',(15.3205561366169,37.4634097578665,15.));
#29061=CARTESIAN_POINT('Ctrl Pts',(15.3210406145546,37.562397408596,15.));
#29062=CARTESIAN_POINT('Ctrl Pts',(15.3208746890781,37.6615277218027,15.));
#29063=CARTESIAN_POINT('Ctrl Pts',(15.320070396385,37.7607947318286,15.));
#29064=CARTESIAN_POINT('Ctrl Pts',(15.3186394335023,37.8601926265378,15.));
#29065=CARTESIAN_POINT('Ctrl Pts',(15.3165911656268,37.959716421934,15.));
#29066=CARTESIAN_POINT('Ctrl Pts',(15.3139321941687,38.0593621055415,15.));
#29067=CARTESIAN_POINT('Ctrl Pts',(15.310667421514,38.1591262705847,15.));
#29068=CARTESIAN_POINT('Ctrl Pts',(15.3068007250314,38.2590058835965,15.));
#29069=CARTESIAN_POINT('Ctrl Pts',(15.3023357307483,38.3589980188324,15.));
#29070=CARTESIAN_POINT('Ctrl Pts',(15.297276703747,38.4590995527814,15.));
#29071=CARTESIAN_POINT('Ctrl Pts',(15.2916287700102,38.5593070891769,15.));
#29072=CARTESIAN_POINT('Ctrl Pts',(15.2853974668211,38.659617115053,15.));
#29073=CARTESIAN_POINT('Ctrl Pts',(15.2785884727112,38.7600260961351,15.));
#29074=CARTESIAN_POINT('Ctrl Pts',(15.2712072937639,38.860530586589,15.));
#29075=CARTESIAN_POINT('Ctrl Pts',(15.2632589109473,38.9611273555758,15.));
#29076=CARTESIAN_POINT('Ctrl Pts',(15.2547476855825,39.061813415425,15.));
#29077=CARTESIAN_POINT('Ctrl Pts',(15.2456775636447,39.1625859371304,15.));
#29078=CARTESIAN_POINT('Ctrl Pts',(15.2360522089072,39.2634421927888,15.));
#29079=CARTESIAN_POINT('Ctrl Pts',(15.225875156307,39.3643794927167,15.));
#29080=CARTESIAN_POINT('Ctrl Pts',(15.2151499908149,39.4653951093947,15.));
#29081=CARTESIAN_POINT('Ctrl Pts',(15.2038804098649,39.5664862602472,15.));
#29082=CARTESIAN_POINT('Ctrl Pts',(15.1920701163804,39.6676501731673,15.));
#29083=CARTESIAN_POINT('Ctrl Pts',(15.1797227547562,39.7688841338802,15.));
#29084=CARTESIAN_POINT('Ctrl Pts',(15.1668418393198,39.8701855339908,15.));
#29085=CARTESIAN_POINT('Ctrl Pts',(15.1534306754871,39.9715519332134,15.));
#29086=CARTESIAN_POINT('Ctrl Pts',(15.1394923361537,40.0729810652204,15.));
#29087=CARTESIAN_POINT('Ctrl Pts',(15.1250297462408,40.1744707357902,15.));
#29088=CARTESIAN_POINT('Ctrl Pts',(15.1100457495259,40.2760187401822,15.));
#29089=CARTESIAN_POINT('Ctrl Pts',(15.0945431800724,40.3776227809037,15.));
#29090=CARTESIAN_POINT('Ctrl Pts',(15.0785249502524,40.4792803645352,15.));
#29091=CARTESIAN_POINT('Ctrl Pts',(15.0619940893017,40.5809887704301,15.));
#29092=CARTESIAN_POINT('Ctrl Pts',(15.0449536183143,40.6827452453667,15.));
#29093=CARTESIAN_POINT('Ctrl Pts',(15.0274064563211,40.7845471608654,15.));
#29094=CARTESIAN_POINT('Ctrl Pts',(15.0093553188655,40.8863921801,15.));
#29095=CARTESIAN_POINT('Ctrl Pts',(14.9908026205824,40.9882784321884,15.));
#29096=CARTESIAN_POINT('Ctrl Pts',(14.9679399407908,41.1105898934098,15.));
#29097=CARTESIAN_POINT('Ctrl Pts',(14.9482653093396,41.2125650743922,15.));
#29098=CARTESIAN_POINT('Ctrl Pts',(14.9321285285561,41.2941761025922,15.));
#29099=CARTESIAN_POINT('Ctrl Pts',(14.919802810928,41.3554017279611,15.));
#29100=CARTESIAN_POINT('Ctrl Pts',(14.911486495888,41.396226524684,15.));
#29101=CARTESIAN_POINT('Ctrl Pts',(24.725498909423,36.3957374383337,0.));
#29102=CARTESIAN_POINT('Ctrl Pts',(24.725498909423,36.3957374383337,18.));
#29103=CARTESIAN_POINT('Ctrl Pts',(24.7065408286023,36.3871033517098,0.));
#29104=CARTESIAN_POINT('Ctrl Pts',(24.7065408286023,36.3871033517098,18.));
#29105=CARTESIAN_POINT('Ctrl Pts',(24.6686569322616,36.369797330215,0.));
#29106=CARTESIAN_POINT('Ctrl Pts',(24.6686569322616,36.369797330215,18.));
#29107=CARTESIAN_POINT('Ctrl Pts',(24.6119278836614,36.3437247532368,0.));
#29108=CARTESIAN_POINT('Ctrl Pts',(24.6119278836614,36.3437247532368,18.));
#29109=CARTESIAN_POINT('Ctrl Pts',(24.5364828082556,36.3087341522969,0.));
#29110=CARTESIAN_POINT('Ctrl Pts',(24.5364828082556,36.3087341522969,18.));
#29111=CARTESIAN_POINT('Ctrl Pts',(24.4424997853604,36.2646168058395,0.));
#29112=CARTESIAN_POINT('Ctrl Pts',(24.4424997853604,36.2646168058395,18.));
#29113=CARTESIAN_POINT('Ctrl Pts',(24.3488411214068,36.2201196586696,0.));
#29114=CARTESIAN_POINT('Ctrl Pts',(24.3488411214068,36.2201196586696,18.));
#29115=CARTESIAN_POINT('Ctrl Pts',(24.2555084095332,36.1752418704833,0.));
#29116=CARTESIAN_POINT('Ctrl Pts',(24.2555084095332,36.1752418704833,18.));
#29117=CARTESIAN_POINT('Ctrl Pts',(24.1625038657964,36.1299825471271,0.));
#29118=CARTESIAN_POINT('Ctrl Pts',(24.1625038657964,36.1299825471271,18.));
#29119=CARTESIAN_POINT('Ctrl Pts',(24.0698304230588,36.0843408347974,0.));
#29120=CARTESIAN_POINT('Ctrl Pts',(24.0698304230588,36.0843408347974,18.));
#29121=CARTESIAN_POINT('Ctrl Pts',(23.9774915680089,36.0383159101253,0.));
#29122=CARTESIAN_POINT('Ctrl Pts',(23.9774915680089,36.0383159101253,18.));
#29123=CARTESIAN_POINT('Ctrl Pts',(23.8854911428946,35.9919069565469,0.));
#29124=CARTESIAN_POINT('Ctrl Pts',(23.8854911428946,35.9919069565469,18.));
#29125=CARTESIAN_POINT('Ctrl Pts',(23.7938331508737,35.9451131482488,0.));
#29126=CARTESIAN_POINT('Ctrl Pts',(23.7938331508737,35.9451131482488,18.));
#29127=CARTESIAN_POINT('Ctrl Pts',(23.7025215735353,35.8979336336837,0.));
#29128=CARTESIAN_POINT('Ctrl Pts',(23.7025215735353,35.8979336336837,18.));
#29129=CARTESIAN_POINT('Ctrl Pts',(23.611560139948,35.8503675222885,0.));
#29130=CARTESIAN_POINT('Ctrl Pts',(23.611560139948,35.8503675222885,18.));
#29131=CARTESIAN_POINT('Ctrl Pts',(23.5209523746427,35.8024138716897,0.));
#29132=CARTESIAN_POINT('Ctrl Pts',(23.5209523746427,35.8024138716897,18.));
#29133=CARTESIAN_POINT('Ctrl Pts',(23.4307017328227,35.7540716771372,0.));
#29134=CARTESIAN_POINT('Ctrl Pts',(23.4307017328227,35.7540716771372,18.));
#29135=CARTESIAN_POINT('Ctrl Pts',(23.3408117088761,35.7053398620512,0.));
#29136=CARTESIAN_POINT('Ctrl Pts',(23.3408117088761,35.7053398620512,18.));
#29137=CARTESIAN_POINT('Ctrl Pts',(23.2512859425032,35.6562172725207,0.));
#29138=CARTESIAN_POINT('Ctrl Pts',(23.2512859425032,35.6562172725207,18.));
#29139=CARTESIAN_POINT('Ctrl Pts',(23.1621283508111,35.6067026687722,0.));
#29140=CARTESIAN_POINT('Ctrl Pts',(23.1621283508111,35.6067026687722,18.));
#29141=CARTESIAN_POINT('Ctrl Pts',(23.0733431097058,35.5567947408311,0.));
#29142=CARTESIAN_POINT('Ctrl Pts',(23.0733431097058,35.5567947408311,18.));
#29143=CARTESIAN_POINT('Ctrl Pts',(22.9849345572033,35.5064921357308,0.));
#29144=CARTESIAN_POINT('Ctrl Pts',(22.9849345572033,35.5064921357308,18.));
#29145=CARTESIAN_POINT('Ctrl Pts',(22.8969071125089,35.4557934871468,0.));
#29146=CARTESIAN_POINT('Ctrl Pts',(22.8969071125089,35.4557934871468,18.));
#29147=CARTESIAN_POINT('Ctrl Pts',(22.8092652000706,35.4046974393492,0.));
#29148=CARTESIAN_POINT('Ctrl Pts',(22.8092652000706,35.4046974393492,18.));
#29149=CARTESIAN_POINT('Ctrl Pts',(22.7220131336912,35.3532026952313,0.));
#29150=CARTESIAN_POINT('Ctrl Pts',(22.7220131336912,35.3532026952313,18.));
#29151=CARTESIAN_POINT('Ctrl Pts',(22.635155167154,35.3013079759252,0.));
#29152=CARTESIAN_POINT('Ctrl Pts',(22.635155167154,35.3013079759252,18.));
#29153=CARTESIAN_POINT('Ctrl Pts',(22.5486956608909,35.2490119207975,0.));
#29154=CARTESIAN_POINT('Ctrl Pts',(22.5486956608909,35.2490119207975,18.));
#29155=CARTESIAN_POINT('Ctrl Pts',(22.4626392230023,35.1963130003352,0.));
#29156=CARTESIAN_POINT('Ctrl Pts',(22.4626392230023,35.1963130003352,18.));
#29157=CARTESIAN_POINT('Ctrl Pts',(22.3769908340843,35.1432094422642,0.));
#29158=CARTESIAN_POINT('Ctrl Pts',(22.3769908340843,35.1432094422642,18.));
#29159=CARTESIAN_POINT('Ctrl Pts',(22.2917560356803,35.0896991159359,0.));
#29160=CARTESIAN_POINT('Ctrl Pts',(22.2917560356803,35.0896991159359,18.));
#29161=CARTESIAN_POINT('Ctrl Pts',(22.2069408519232,35.0357795922459,0.));
#29162=CARTESIAN_POINT('Ctrl Pts',(22.2069408519232,35.0357795922459,18.));
#29163=CARTESIAN_POINT('Ctrl Pts',(22.1225514798584,34.9814483545602,0.));
#29164=CARTESIAN_POINT('Ctrl Pts',(22.1225514798584,34.9814483545602,18.));
#29165=CARTESIAN_POINT('Ctrl Pts',(22.0385940162683,34.9267029879922,0.));
#29166=CARTESIAN_POINT('Ctrl Pts',(22.0385940162683,34.9267029879922,18.));
#29167=CARTESIAN_POINT('Ctrl Pts',(21.9550742217675,34.8715413418101,0.));
#29168=CARTESIAN_POINT('Ctrl Pts',(21.9550742217675,34.8715413418101,18.));
#29169=CARTESIAN_POINT('Ctrl Pts',(21.8719971302817,34.8159618014436,0.));
#29170=CARTESIAN_POINT('Ctrl Pts',(21.8719971302817,34.8159618014436,18.));
#29171=CARTESIAN_POINT('Ctrl Pts',(21.7893672401137,34.7599631530844,0.));
#29172=CARTESIAN_POINT('Ctrl Pts',(21.7893672401137,34.7599631530844,18.));
#29173=CARTESIAN_POINT('Ctrl Pts',(21.7071892844497,34.7035440429025,0.));
#29174=CARTESIAN_POINT('Ctrl Pts',(21.7071892844497,34.7035440429025,18.));
#29175=CARTESIAN_POINT('Ctrl Pts',(21.6254689009796,34.6467025072367,0.));
#29176=CARTESIAN_POINT('Ctrl Pts',(21.6254689009796,34.6467025072367,18.));
#29177=CARTESIAN_POINT('Ctrl Pts',(21.5442132160757,34.5894355639082,0.));
#29178=CARTESIAN_POINT('Ctrl Pts',(21.5442132160757,34.5894355639082,18.));
#29179=CARTESIAN_POINT('Ctrl Pts',(21.4634317666005,34.5317385658329,0.));
#29180=CARTESIAN_POINT('Ctrl Pts',(21.4634317666005,34.5317385658329,18.));
#29181=CARTESIAN_POINT('Ctrl Pts',(21.3831361300104,34.4736054662052,0.));
#29182=CARTESIAN_POINT('Ctrl Pts',(21.3831361300104,34.4736054662052,18.));
#29183=CARTESIAN_POINT('Ctrl Pts',(21.3033382073239,34.4150300340623,0.));
#29184=CARTESIAN_POINT('Ctrl Pts',(21.3033382073239,34.4150300340623,18.));
#29185=CARTESIAN_POINT('Ctrl Pts',(21.2240487218079,34.3560069185815,0.));
#29186=CARTESIAN_POINT('Ctrl Pts',(21.2240487218079,34.3560069185815,18.));
#29187=CARTESIAN_POINT('Ctrl Pts',(21.1452759244399,34.2965325673384,0.));
#29188=CARTESIAN_POINT('Ctrl Pts',(21.1452759244399,34.2965325673384,18.));
#29189=CARTESIAN_POINT('Ctrl Pts',(21.0670234747355,34.2366067284279,0.));
#29190=CARTESIAN_POINT('Ctrl Pts',(21.0670234747355,34.2366067284279,18.));
#29191=CARTESIAN_POINT('Ctrl Pts',(20.9892914622612,34.176231731809,0.));
#29192=CARTESIAN_POINT('Ctrl Pts',(20.9892914622612,34.176231731809,18.));
#29193=CARTESIAN_POINT('Ctrl Pts',(20.9120805673809,34.1154095510973,0.));
#29194=CARTESIAN_POINT('Ctrl Pts',(20.9120805673809,34.1154095510973,18.));
#29195=CARTESIAN_POINT('Ctrl Pts',(20.8353957068415,34.0541392299678,0.));
#29196=CARTESIAN_POINT('Ctrl Pts',(20.8353957068415,34.0541392299678,18.));
#29197=CARTESIAN_POINT('Ctrl Pts',(20.7592491770603,33.9924146647395,0.));
#29198=CARTESIAN_POINT('Ctrl Pts',(20.7592491770603,33.9924146647395,18.));
#29199=CARTESIAN_POINT('Ctrl Pts',(20.683665762903,33.9302209962425,0.));
#29200=CARTESIAN_POINT('Ctrl Pts',(20.683665762903,33.9302209962425,18.));
#29201=CARTESIAN_POINT('Ctrl Pts',(20.6086800574386,33.8675365150454,0.));
#29202=CARTESIAN_POINT('Ctrl Pts',(20.6086800574386,33.8675365150454,18.));
#29203=CARTESIAN_POINT('Ctrl Pts',(20.5343269914034,33.8043393734971,0.));
#29204=CARTESIAN_POINT('Ctrl Pts',(20.5343269914034,33.8043393734971,18.));
#29205=CARTESIAN_POINT('Ctrl Pts',(20.4606334536183,33.7406135254082,0.));
#29206=CARTESIAN_POINT('Ctrl Pts',(20.4606334536183,33.7406135254082,18.));
#29207=CARTESIAN_POINT('Ctrl Pts',(20.3876111773341,33.6763537716992,0.));
#29208=CARTESIAN_POINT('Ctrl Pts',(20.3876111773341,33.6763537716992,18.));
#29209=CARTESIAN_POINT('Ctrl Pts',(20.3152448035298,33.6115742164079,0.));
#29210=CARTESIAN_POINT('Ctrl Pts',(20.3152448035298,33.6115742164079,18.));
#29211=CARTESIAN_POINT('Ctrl Pts',(20.243500298383,33.5463023319603,0.));
#29212=CARTESIAN_POINT('Ctrl Pts',(20.243500298383,33.5463023319603,18.));
#29213=CARTESIAN_POINT('Ctrl Pts',(20.1723475154533,33.480563024813,0.));
#29214=CARTESIAN_POINT('Ctrl Pts',(20.1723475154533,33.480563024813,18.));
#29215=CARTESIAN_POINT('Ctrl Pts',(20.1017803986381,33.4143643679979,0.));
#29216=CARTESIAN_POINT('Ctrl Pts',(20.1017803986381,33.4143643679979,18.));
#29217=CARTESIAN_POINT('Ctrl Pts',(20.0318342617212,33.3476854048385,0.));
#29218=CARTESIAN_POINT('Ctrl Pts',(20.0318342617212,33.3476854048385,18.));
#29219=CARTESIAN_POINT('Ctrl Pts',(19.9626141625205,33.2804560993213,0.));
#29220=CARTESIAN_POINT('Ctrl Pts',(19.9626141625205,33.2804560993213,18.));
#29221=CARTESIAN_POINT('Ctrl Pts',(19.8942704458546,33.2125746879471,0.));
#29222=CARTESIAN_POINT('Ctrl Pts',(19.8942704458546,33.2125746879471,18.));
#29223=CARTESIAN_POINT('Ctrl Pts',(19.8269479776239,33.1439436707661,0.));
#29224=CARTESIAN_POINT('Ctrl Pts',(19.8269479776239,33.1439436707661,18.));
#29225=CARTESIAN_POINT('Ctrl Pts',(19.7607398248651,33.0745026283418,0.));
#29226=CARTESIAN_POINT('Ctrl Pts',(19.7607398248651,33.0745026283418,18.));
#29227=CARTESIAN_POINT('Ctrl Pts',(19.6956473461873,33.004256563411,0.));
#29228=CARTESIAN_POINT('Ctrl Pts',(19.6956473461873,33.004256563411,18.));
#29229=CARTESIAN_POINT('Ctrl Pts',(19.6315161742485,32.9333211533788,0.));
#29230=CARTESIAN_POINT('Ctrl Pts',(19.6315161742485,32.9333211533788,18.));
#29231=CARTESIAN_POINT('Ctrl Pts',(19.5681157030437,32.8618672807884,0.));
#29232=CARTESIAN_POINT('Ctrl Pts',(19.5681157030437,32.8618672807884,18.));
#29233=CARTESIAN_POINT('Ctrl Pts',(19.5052640847974,32.7900335943248,0.));
#29234=CARTESIAN_POINT('Ctrl Pts',(19.5052640847974,32.7900335943248,18.));
#29235=CARTESIAN_POINT('Ctrl Pts',(19.4429429601189,32.7178463324062,0.));
#29236=CARTESIAN_POINT('Ctrl Pts',(19.4429429601189,32.7178463324062,18.));
#29237=CARTESIAN_POINT('Ctrl Pts',(19.381405831319,32.6451434870609,0.));
#29238=CARTESIAN_POINT('Ctrl Pts',(19.381405831319,32.6451434870609,18.));
#29239=CARTESIAN_POINT('Ctrl Pts',(19.3213180490743,32.5714771007861,0.));
#29240=CARTESIAN_POINT('Ctrl Pts',(19.3213180490743,32.5714771007861,18.));
#29241=CARTESIAN_POINT('Ctrl Pts',(19.2635813403783,32.4962340238036,0.));
#29242=CARTESIAN_POINT('Ctrl Pts',(19.2635813403783,32.4962340238036,18.));
#29243=CARTESIAN_POINT('Ctrl Pts',(19.2200039764927,32.4342791270009,0.));
#29244=CARTESIAN_POINT('Ctrl Pts',(19.2200039764927,32.4342791270009,18.));
#29245=CARTESIAN_POINT('Ctrl Pts',(19.1891139208368,32.3866012518553,0.));
#29246=CARTESIAN_POINT('Ctrl Pts',(19.1891139208368,32.3866012518553,18.));
#29247=CARTESIAN_POINT('Ctrl Pts',(19.1693587749508,32.3542491343753,0.));
#29248=CARTESIAN_POINT('Ctrl Pts',(19.1693587749508,32.3542491343753,18.));
#29249=CARTESIAN_POINT('Ctrl Pts',(19.1596907609891,32.3379313568208,0.));
#29250=CARTESIAN_POINT('Ctrl Pts',(19.1596907609891,32.3379313568208,18.));
#29251=CARTESIAN_POINT('',(24.7254989094229,36.3957374383337,0.));
#29252=CARTESIAN_POINT('Ctrl Pts',(19.1596907609891,32.3379313568208,0.));
#29253=CARTESIAN_POINT('Ctrl Pts',(19.1693587749508,32.3542491343753,0.));
#29254=CARTESIAN_POINT('Ctrl Pts',(19.1891139208368,32.3866012518553,0.));
#29255=CARTESIAN_POINT('Ctrl Pts',(19.2200039764927,32.4342791270009,0.));
#29256=CARTESIAN_POINT('Ctrl Pts',(19.2635813403783,32.4962340238036,0.));
#29257=CARTESIAN_POINT('Ctrl Pts',(19.3213180490743,32.5714771007861,0.));
#29258=CARTESIAN_POINT('Ctrl Pts',(19.381405831319,32.6451434870609,0.));
#29259=CARTESIAN_POINT('Ctrl Pts',(19.4429429601189,32.7178463324062,0.));
#29260=CARTESIAN_POINT('Ctrl Pts',(19.5052640847974,32.7900335943248,0.));
#29261=CARTESIAN_POINT('Ctrl Pts',(19.5681157030437,32.8618672807884,0.));
#29262=CARTESIAN_POINT('Ctrl Pts',(19.6315161742485,32.9333211533788,0.));
#29263=CARTESIAN_POINT('Ctrl Pts',(19.6956473461873,33.004256563411,0.));
#29264=CARTESIAN_POINT('Ctrl Pts',(19.7607398248651,33.0745026283418,0.));
#29265=CARTESIAN_POINT('Ctrl Pts',(19.8269479776239,33.1439436707661,0.));
#29266=CARTESIAN_POINT('Ctrl Pts',(19.8942704458546,33.2125746879471,0.));
#29267=CARTESIAN_POINT('Ctrl Pts',(19.9626141625205,33.2804560993213,0.));
#29268=CARTESIAN_POINT('Ctrl Pts',(20.0318342617212,33.3476854048385,0.));
#29269=CARTESIAN_POINT('Ctrl Pts',(20.1017803986381,33.4143643679979,0.));
#29270=CARTESIAN_POINT('Ctrl Pts',(20.1723475154533,33.480563024813,0.));
#29271=CARTESIAN_POINT('Ctrl Pts',(20.243500298383,33.5463023319603,0.));
#29272=CARTESIAN_POINT('Ctrl Pts',(20.3152448035298,33.6115742164079,0.));
#29273=CARTESIAN_POINT('Ctrl Pts',(20.3876111773341,33.6763537716992,0.));
#29274=CARTESIAN_POINT('Ctrl Pts',(20.4606334536183,33.7406135254082,0.));
#29275=CARTESIAN_POINT('Ctrl Pts',(20.5343269914034,33.8043393734971,0.));
#29276=CARTESIAN_POINT('Ctrl Pts',(20.6086800574386,33.8675365150454,0.));
#29277=CARTESIAN_POINT('Ctrl Pts',(20.683665762903,33.9302209962425,0.));
#29278=CARTESIAN_POINT('Ctrl Pts',(20.7592491770603,33.9924146647395,0.));
#29279=CARTESIAN_POINT('Ctrl Pts',(20.8353957068415,34.0541392299678,0.));
#29280=CARTESIAN_POINT('Ctrl Pts',(20.9120805673809,34.1154095510973,0.));
#29281=CARTESIAN_POINT('Ctrl Pts',(20.9892914622612,34.176231731809,0.));
#29282=CARTESIAN_POINT('Ctrl Pts',(21.0670234747355,34.2366067284279,0.));
#29283=CARTESIAN_POINT('Ctrl Pts',(21.1452759244399,34.2965325673384,0.));
#29284=CARTESIAN_POINT('Ctrl Pts',(21.2240487218079,34.3560069185815,0.));
#29285=CARTESIAN_POINT('Ctrl Pts',(21.3033382073239,34.4150300340623,0.));
#29286=CARTESIAN_POINT('Ctrl Pts',(21.3831361300104,34.4736054662052,0.));
#29287=CARTESIAN_POINT('Ctrl Pts',(21.4634317666005,34.5317385658329,0.));
#29288=CARTESIAN_POINT('Ctrl Pts',(21.5442132160757,34.5894355639082,0.));
#29289=CARTESIAN_POINT('Ctrl Pts',(21.6254689009796,34.6467025072367,0.));
#29290=CARTESIAN_POINT('Ctrl Pts',(21.7071892844497,34.7035440429025,0.));
#29291=CARTESIAN_POINT('Ctrl Pts',(21.7893672401137,34.7599631530844,0.));
#29292=CARTESIAN_POINT('Ctrl Pts',(21.8719971302817,34.8159618014436,0.));
#29293=CARTESIAN_POINT('Ctrl Pts',(21.9550742217675,34.8715413418101,0.));
#29294=CARTESIAN_POINT('Ctrl Pts',(22.0385940162683,34.9267029879922,0.));
#29295=CARTESIAN_POINT('Ctrl Pts',(22.1225514798584,34.9814483545602,0.));
#29296=CARTESIAN_POINT('Ctrl Pts',(22.2069408519232,35.0357795922459,0.));
#29297=CARTESIAN_POINT('Ctrl Pts',(22.2917560356803,35.0896991159359,0.));
#29298=CARTESIAN_POINT('Ctrl Pts',(22.3769908340843,35.1432094422642,0.));
#29299=CARTESIAN_POINT('Ctrl Pts',(22.4626392230023,35.1963130003352,0.));
#29300=CARTESIAN_POINT('Ctrl Pts',(22.5486956608909,35.2490119207975,0.));
#29301=CARTESIAN_POINT('Ctrl Pts',(22.635155167154,35.3013079759252,0.));
#29302=CARTESIAN_POINT('Ctrl Pts',(22.7220131336912,35.3532026952313,0.));
#29303=CARTESIAN_POINT('Ctrl Pts',(22.8092652000706,35.4046974393492,0.));
#29304=CARTESIAN_POINT('Ctrl Pts',(22.8969071125089,35.4557934871468,0.));
#29305=CARTESIAN_POINT('Ctrl Pts',(22.9849345572033,35.5064921357308,0.));
#29306=CARTESIAN_POINT('Ctrl Pts',(23.0733431097058,35.5567947408311,0.));
#29307=CARTESIAN_POINT('Ctrl Pts',(23.1621283508111,35.6067026687722,0.));
#29308=CARTESIAN_POINT('Ctrl Pts',(23.2512859425032,35.6562172725207,0.));
#29309=CARTESIAN_POINT('Ctrl Pts',(23.3408117088761,35.7053398620512,0.));
#29310=CARTESIAN_POINT('Ctrl Pts',(23.4307017328227,35.7540716771372,0.));
#29311=CARTESIAN_POINT('Ctrl Pts',(23.5209523746427,35.8024138716897,0.));
#29312=CARTESIAN_POINT('Ctrl Pts',(23.611560139948,35.8503675222885,0.));
#29313=CARTESIAN_POINT('Ctrl Pts',(23.7025215735353,35.8979336336837,0.));
#29314=CARTESIAN_POINT('Ctrl Pts',(23.7938331508737,35.9451131482488,0.));
#29315=CARTESIAN_POINT('Ctrl Pts',(23.8854911428946,35.9919069565469,0.));
#29316=CARTESIAN_POINT('Ctrl Pts',(23.9774915680089,36.0383159101253,0.));
#29317=CARTESIAN_POINT('Ctrl Pts',(24.0698304230588,36.0843408347974,0.));
#29318=CARTESIAN_POINT('Ctrl Pts',(24.1625038657964,36.1299825471271,0.));
#29319=CARTESIAN_POINT('Ctrl Pts',(24.2555084095332,36.1752418704833,0.));
#29320=CARTESIAN_POINT('Ctrl Pts',(24.3488411214068,36.2201196586696,0.));
#29321=CARTESIAN_POINT('Ctrl Pts',(24.4612315181511,36.2735162352735,0.));
#29322=CARTESIAN_POINT('Ctrl Pts',(24.5552956307817,36.3175386315528,0.));
#29323=CARTESIAN_POINT('Ctrl Pts',(24.630805301288,36.3524534604648,0.));
#29324=CARTESIAN_POINT('Ctrl Pts',(24.6875827477484,36.3784692650901,0.));
#29325=CARTESIAN_POINT('Ctrl Pts',(24.725498909423,36.3957374383337,0.));
#29326=CARTESIAN_POINT('',(24.7254989094229,36.3957374383337,15.));
#29327=CARTESIAN_POINT('Ctrl Pts',(24.725498909423,36.3957374383337,15.));
#29328=CARTESIAN_POINT('Ctrl Pts',(24.7065408286023,36.3871033517098,15.));
#29329=CARTESIAN_POINT('Ctrl Pts',(24.6686569322616,36.369797330215,15.));
#29330=CARTESIAN_POINT('Ctrl Pts',(24.6119278836614,36.3437247532368,15.));
#29331=CARTESIAN_POINT('Ctrl Pts',(24.5364828082556,36.3087341522969,15.));
#29332=CARTESIAN_POINT('Ctrl Pts',(24.4424997853604,36.2646168058395,15.));
#29333=CARTESIAN_POINT('Ctrl Pts',(24.3488411214068,36.2201196586696,15.));
#29334=CARTESIAN_POINT('Ctrl Pts',(24.2555084095332,36.1752418704833,15.));
#29335=CARTESIAN_POINT('Ctrl Pts',(24.1625038657964,36.1299825471271,15.));
#29336=CARTESIAN_POINT('Ctrl Pts',(24.0698304230588,36.0843408347974,15.));
#29337=CARTESIAN_POINT('Ctrl Pts',(23.9774915680089,36.0383159101253,15.));
#29338=CARTESIAN_POINT('Ctrl Pts',(23.8854911428946,35.9919069565469,15.));
#29339=CARTESIAN_POINT('Ctrl Pts',(23.7938331508737,35.9451131482488,15.));
#29340=CARTESIAN_POINT('Ctrl Pts',(23.7025215735353,35.8979336336837,15.));
#29341=CARTESIAN_POINT('Ctrl Pts',(23.611560139948,35.8503675222885,15.));
#29342=CARTESIAN_POINT('Ctrl Pts',(23.5209523746427,35.8024138716897,15.));
#29343=CARTESIAN_POINT('Ctrl Pts',(23.4307017328227,35.7540716771372,15.));
#29344=CARTESIAN_POINT('Ctrl Pts',(23.3408117088761,35.7053398620512,15.));
#29345=CARTESIAN_POINT('Ctrl Pts',(23.2512859425032,35.6562172725207,15.));
#29346=CARTESIAN_POINT('Ctrl Pts',(23.1621283508111,35.6067026687722,15.));
#29347=CARTESIAN_POINT('Ctrl Pts',(23.0733431097058,35.5567947408311,15.));
#29348=CARTESIAN_POINT('Ctrl Pts',(22.9849345572033,35.5064921357308,15.));
#29349=CARTESIAN_POINT('Ctrl Pts',(22.8969071125089,35.4557934871468,15.));
#29350=CARTESIAN_POINT('Ctrl Pts',(22.8092652000706,35.4046974393492,15.));
#29351=CARTESIAN_POINT('Ctrl Pts',(22.7220131336912,35.3532026952313,15.));
#29352=CARTESIAN_POINT('Ctrl Pts',(22.635155167154,35.3013079759252,15.));
#29353=CARTESIAN_POINT('Ctrl Pts',(22.5486956608909,35.2490119207975,15.));
#29354=CARTESIAN_POINT('Ctrl Pts',(22.4626392230023,35.1963130003352,15.));
#29355=CARTESIAN_POINT('Ctrl Pts',(22.3769908340843,35.1432094422642,15.));
#29356=CARTESIAN_POINT('Ctrl Pts',(22.2917560356803,35.0896991159359,15.));
#29357=CARTESIAN_POINT('Ctrl Pts',(22.2069408519232,35.0357795922459,15.));
#29358=CARTESIAN_POINT('Ctrl Pts',(22.1225514798584,34.9814483545602,15.));
#29359=CARTESIAN_POINT('Ctrl Pts',(22.0385940162683,34.9267029879922,15.));
#29360=CARTESIAN_POINT('Ctrl Pts',(21.9550742217675,34.8715413418101,15.));
#29361=CARTESIAN_POINT('Ctrl Pts',(21.8719971302817,34.8159618014436,15.));
#29362=CARTESIAN_POINT('Ctrl Pts',(21.7893672401137,34.7599631530844,15.));
#29363=CARTESIAN_POINT('Ctrl Pts',(21.7071892844497,34.7035440429025,15.));
#29364=CARTESIAN_POINT('Ctrl Pts',(21.6254689009796,34.6467025072367,15.));
#29365=CARTESIAN_POINT('Ctrl Pts',(21.5442132160757,34.5894355639082,15.));
#29366=CARTESIAN_POINT('Ctrl Pts',(21.4634317666005,34.5317385658329,15.));
#29367=CARTESIAN_POINT('Ctrl Pts',(21.3831361300104,34.4736054662052,15.));
#29368=CARTESIAN_POINT('Ctrl Pts',(21.3033382073239,34.4150300340623,15.));
#29369=CARTESIAN_POINT('Ctrl Pts',(21.2240487218079,34.3560069185815,15.));
#29370=CARTESIAN_POINT('Ctrl Pts',(21.1452759244399,34.2965325673384,15.));
#29371=CARTESIAN_POINT('Ctrl Pts',(21.0670234747355,34.2366067284279,15.));
#29372=CARTESIAN_POINT('Ctrl Pts',(20.9892914622612,34.176231731809,15.));
#29373=CARTESIAN_POINT('Ctrl Pts',(20.9120805673809,34.1154095510973,15.));
#29374=CARTESIAN_POINT('Ctrl Pts',(20.8353957068415,34.0541392299678,15.));
#29375=CARTESIAN_POINT('Ctrl Pts',(20.7592491770603,33.9924146647395,15.));
#29376=CARTESIAN_POINT('Ctrl Pts',(20.683665762903,33.9302209962425,15.));
#29377=CARTESIAN_POINT('Ctrl Pts',(20.6086800574386,33.8675365150454,15.));
#29378=CARTESIAN_POINT('Ctrl Pts',(20.5343269914034,33.8043393734971,15.));
#29379=CARTESIAN_POINT('Ctrl Pts',(20.4606334536183,33.7406135254082,15.));
#29380=CARTESIAN_POINT('Ctrl Pts',(20.3876111773341,33.6763537716992,15.));
#29381=CARTESIAN_POINT('Ctrl Pts',(20.3152448035298,33.6115742164079,15.));
#29382=CARTESIAN_POINT('Ctrl Pts',(20.243500298383,33.5463023319603,15.));
#29383=CARTESIAN_POINT('Ctrl Pts',(20.1723475154533,33.480563024813,15.));
#29384=CARTESIAN_POINT('Ctrl Pts',(20.1017803986381,33.4143643679979,15.));
#29385=CARTESIAN_POINT('Ctrl Pts',(20.0318342617212,33.3476854048385,15.));
#29386=CARTESIAN_POINT('Ctrl Pts',(19.9626141625205,33.2804560993213,15.));
#29387=CARTESIAN_POINT('Ctrl Pts',(19.8942704458546,33.2125746879471,15.));
#29388=CARTESIAN_POINT('Ctrl Pts',(19.8269479776239,33.1439436707661,15.));
#29389=CARTESIAN_POINT('Ctrl Pts',(19.7607398248651,33.0745026283418,15.));
#29390=CARTESIAN_POINT('Ctrl Pts',(19.6956473461873,33.004256563411,15.));
#29391=CARTESIAN_POINT('Ctrl Pts',(19.6315161742485,32.9333211533788,15.));
#29392=CARTESIAN_POINT('Ctrl Pts',(19.5681157030437,32.8618672807884,15.));
#29393=CARTESIAN_POINT('Ctrl Pts',(19.5052640847974,32.7900335943248,15.));
#29394=CARTESIAN_POINT('Ctrl Pts',(19.4429429601189,32.7178463324062,15.));
#29395=CARTESIAN_POINT('Ctrl Pts',(19.381405831319,32.6451434870609,15.));
#29396=CARTESIAN_POINT('Ctrl Pts',(19.3213180490743,32.5714771007861,15.));
#29397=CARTESIAN_POINT('Ctrl Pts',(19.2635813403783,32.4962340238036,15.));
#29398=CARTESIAN_POINT('Ctrl Pts',(19.2200039764927,32.4342791270009,15.));
#29399=CARTESIAN_POINT('Ctrl Pts',(19.1891139208368,32.3866012518553,15.));
#29400=CARTESIAN_POINT('Ctrl Pts',(19.1693587749508,32.3542491343753,15.));
#29401=CARTESIAN_POINT('Ctrl Pts',(19.1596907609891,32.3379313568208,15.));
#29402=CARTESIAN_POINT('',(24.7254989094229,36.3957374383337,0.));
#29403=CARTESIAN_POINT('Origin',(6.66146233219319E-12,9.16871631793044E-12,
0.));
#29404=CARTESIAN_POINT('',(26.9738038986838,34.762248247709,0.));
#29405=CARTESIAN_POINT('Origin',(6.66146233219319E-12,9.16871631793044E-12,
0.));
#29406=CARTESIAN_POINT('',(26.9738038986838,34.762248247709,15.));
#29407=CARTESIAN_POINT('Origin',(6.66146233219319E-12,9.16871631793044E-12,
15.));
#29408=CARTESIAN_POINT('',(26.9738038986838,34.762248247709,0.));
#29409=CARTESIAN_POINT('Ctrl Pts',(24.8345302882955,28.2149191006268,0.));
#29410=CARTESIAN_POINT('Ctrl Pts',(24.8345302882955,28.2149191006268,18.));
#29411=CARTESIAN_POINT('Ctrl Pts',(24.8470618363541,28.2291563988796,0.));
#29412=CARTESIAN_POINT('Ctrl Pts',(24.8470618363541,28.2291563988796,18.));
#29413=CARTESIAN_POINT('Ctrl Pts',(24.8717258526943,28.2579420132101,0.));
#29414=CARTESIAN_POINT('Ctrl Pts',(24.8717258526943,28.2579420132101,18.));
#29415=CARTESIAN_POINT('Ctrl Pts',(24.9075246543798,28.3020534756061,0.));
#29416=CARTESIAN_POINT('Ctrl Pts',(24.9075246543798,28.3020534756061,18.));
#29417=CARTESIAN_POINT('Ctrl Pts',(24.9529811166897,28.3626431274892,0.));
#29418=CARTESIAN_POINT('Ctrl Pts',(24.9529811166897,28.3626431274892,18.));
#29419=CARTESIAN_POINT('Ctrl Pts',(25.0066999111736,28.4408053900206,0.));
#29420=CARTESIAN_POINT('Ctrl Pts',(25.0066999111736,28.4408053900206,18.));
#29421=CARTESIAN_POINT('Ctrl Pts',(25.0581926620043,28.5207164321473,0.));
#29422=CARTESIAN_POINT('Ctrl Pts',(25.0581926620043,28.5207164321473,18.));
#29423=CARTESIAN_POINT('Ctrl Pts',(25.1083211582389,28.6017081342376,0.));
#29424=CARTESIAN_POINT('Ctrl Pts',(25.1083211582389,28.6017081342376,18.));
#29425=CARTESIAN_POINT('Ctrl Pts',(25.1577170374459,28.6832861366762,0.));
#29426=CARTESIAN_POINT('Ctrl Pts',(25.1577170374459,28.6832861366762,18.));
#29427=CARTESIAN_POINT('Ctrl Pts',(25.2066127148845,28.7652594076549,0.));
#29428=CARTESIAN_POINT('Ctrl Pts',(25.2066127148845,28.7652594076549,18.));
#29429=CARTESIAN_POINT('Ctrl Pts',(25.2549775629725,28.8476372998748,0.));
#29430=CARTESIAN_POINT('Ctrl Pts',(25.2549775629725,28.8476372998748,18.));
#29431=CARTESIAN_POINT('Ctrl Pts',(25.3026235249214,28.9305499160476,0.));
#29432=CARTESIAN_POINT('Ctrl Pts',(25.3026235249214,28.9305499160476,18.));
#29433=CARTESIAN_POINT('Ctrl Pts',(25.3493168206005,29.0141637699076,0.));
#29434=CARTESIAN_POINT('Ctrl Pts',(25.3493168206005,29.0141637699076,18.));
#29435=CARTESIAN_POINT('Ctrl Pts',(25.3948997321279,29.098589927237,0.));
#29436=CARTESIAN_POINT('Ctrl Pts',(25.3948997321279,29.098589927237,18.));
#29437=CARTESIAN_POINT('Ctrl Pts',(25.4393679214513,29.183825549991,0.));
#29438=CARTESIAN_POINT('Ctrl Pts',(25.4393679214513,29.183825549991,18.));
#29439=CARTESIAN_POINT('Ctrl Pts',(25.4828076101654,29.2698007967907,0.));
#29440=CARTESIAN_POINT('Ctrl Pts',(25.4828076101654,29.2698007967907,18.));
#29441=CARTESIAN_POINT('Ctrl Pts',(25.5253562922582,29.356408021119,0.));
#29442=CARTESIAN_POINT('Ctrl Pts',(25.5253562922582,29.356408021119,18.));
#29443=CARTESIAN_POINT('Ctrl Pts',(25.5671572096726,29.443535683207,0.));
#29444=CARTESIAN_POINT('Ctrl Pts',(25.5671572096726,29.443535683207,18.));
#29445=CARTESIAN_POINT('Ctrl Pts',(25.6083094352667,29.5311055094509,0.));
#29446=CARTESIAN_POINT('Ctrl Pts',(25.6083094352667,29.5311055094509,18.));
#29447=CARTESIAN_POINT('Ctrl Pts',(25.6488438125835,29.6190903904157,0.));
#29448=CARTESIAN_POINT('Ctrl Pts',(25.6488438125835,29.6190903904157,18.));
#29449=CARTESIAN_POINT('Ctrl Pts',(25.6887507922748,29.7074935910931,0.));
#29450=CARTESIAN_POINT('Ctrl Pts',(25.6887507922748,29.7074935910931,18.));
#29451=CARTESIAN_POINT('Ctrl Pts',(25.7279973711305,29.7963360859334,0.));
#29452=CARTESIAN_POINT('Ctrl Pts',(25.7279973711305,29.7963360859334,18.));
#29453=CARTESIAN_POINT('Ctrl Pts',(25.7665469042913,29.8856417535786,0.));
#29454=CARTESIAN_POINT('Ctrl Pts',(25.7665469042913,29.8856417535786,18.));
#29455=CARTESIAN_POINT('Ctrl Pts',(25.8043812318214,29.9754208429384,0.));
#29456=CARTESIAN_POINT('Ctrl Pts',(25.8043812318214,29.9754208429384,18.));
#29457=CARTESIAN_POINT('Ctrl Pts',(25.8415089241134,30.0656638016321,0.));
#29458=CARTESIAN_POINT('Ctrl Pts',(25.8415089241134,30.0656638016321,18.));
#29459=CARTESIAN_POINT('Ctrl Pts',(25.8779535511027,30.1563500154165,0.));
#29460=CARTESIAN_POINT('Ctrl Pts',(25.8779535511027,30.1563500154165,18.));
#29461=CARTESIAN_POINT('Ctrl Pts',(25.9137466853317,30.2474530144827,0.));
#29462=CARTESIAN_POINT('Ctrl Pts',(25.9137466853317,30.2474530144827,18.));
#29463=CARTESIAN_POINT('Ctrl Pts',(25.9489196635424,30.3389466074503,0.));
#29464=CARTESIAN_POINT('Ctrl Pts',(25.9489196635424,30.3389466074503,18.));
#29465=CARTESIAN_POINT('Ctrl Pts',(25.9834942765902,30.4308118142473,0.));
#29466=CARTESIAN_POINT('Ctrl Pts',(25.9834942765902,30.4308118142473,18.));
#29467=CARTESIAN_POINT('Ctrl Pts',(26.0174801292225,30.5230388264271,0.));
#29468=CARTESIAN_POINT('Ctrl Pts',(26.0174801292225,30.5230388264271,18.));
#29469=CARTESIAN_POINT('Ctrl Pts',(26.0508796503166,30.6156232634061,0.));
#29470=CARTESIAN_POINT('Ctrl Pts',(26.0508796503166,30.6156232634061,18.));
#29471=CARTESIAN_POINT('Ctrl Pts',(26.0836911730968,30.7085638682391,0.));
#29472=CARTESIAN_POINT('Ctrl Pts',(26.0836911730968,30.7085638682391,18.));
#29473=CARTESIAN_POINT('Ctrl Pts',(26.1159125093178,30.8018598357461,0.));
#29474=CARTESIAN_POINT('Ctrl Pts',(26.1159125093178,30.8018598357461,18.));
#29475=CARTESIAN_POINT('Ctrl Pts',(26.1475450294082,30.8955077633644,0.));
#29476=CARTESIAN_POINT('Ctrl Pts',(26.1475450294082,30.8955077633644,18.));
#29477=CARTESIAN_POINT('Ctrl Pts',(26.1785946616165,30.9895009017073,0.));
#29478=CARTESIAN_POINT('Ctrl Pts',(26.1785946616165,30.9895009017073,18.));
#29479=CARTESIAN_POINT('Ctrl Pts',(26.2090698085494,31.0838307058369,0.));
#29480=CARTESIAN_POINT('Ctrl Pts',(26.2090698085494,31.0838307058369,18.));
#29481=CARTESIAN_POINT('Ctrl Pts',(26.2389800738215,31.1784877826858,0.));
#29482=CARTESIAN_POINT('Ctrl Pts',(26.2389800738215,31.1784877826858,18.));
#29483=CARTESIAN_POINT('Ctrl Pts',(26.2683347859175,31.2734629900041,0.));
#29484=CARTESIAN_POINT('Ctrl Pts',(26.2683347859175,31.2734629900041,18.));
#29485=CARTESIAN_POINT('Ctrl Pts',(26.2971413115295,31.3687486937246,0.));
#29486=CARTESIAN_POINT('Ctrl Pts',(26.2971413115295,31.3687486937246,18.));
#29487=CARTESIAN_POINT('Ctrl Pts',(26.3254046890485,31.4643390378084,0.));
#29488=CARTESIAN_POINT('Ctrl Pts',(26.3254046890485,31.4643390378084,18.));
#29489=CARTESIAN_POINT('Ctrl Pts',(26.353128528169,31.5602292672984,0.));
#29490=CARTESIAN_POINT('Ctrl Pts',(26.353128528169,31.5602292672984,18.));
#29491=CARTESIAN_POINT('Ctrl Pts',(26.3803155790949,31.6564152990236,0.));
#29492=CARTESIAN_POINT('Ctrl Pts',(26.3803155790949,31.6564152990236,18.));
#29493=CARTESIAN_POINT('Ctrl Pts',(26.4069683862784,31.7528932299312,0.));
#29494=CARTESIAN_POINT('Ctrl Pts',(26.4069683862784,31.7528932299312,18.));
#29495=CARTESIAN_POINT('Ctrl Pts',(26.433090040836,31.849658771403,0.));
#29496=CARTESIAN_POINT('Ctrl Pts',(26.433090040836,31.849658771403,18.));
#29497=CARTESIAN_POINT('Ctrl Pts',(26.4586843683627,31.9467071093816,0.));
#29498=CARTESIAN_POINT('Ctrl Pts',(26.4586843683627,31.9467071093816,18.));
#29499=CARTESIAN_POINT('Ctrl Pts',(26.4837555495616,32.0440331917233,0.));
#29500=CARTESIAN_POINT('Ctrl Pts',(26.4837555495616,32.0440331917233,18.));
#29501=CARTESIAN_POINT('Ctrl Pts',(26.5083078928862,32.1416319023705,0.));
#29502=CARTESIAN_POINT('Ctrl Pts',(26.5083078928862,32.1416319023705,18.));
#29503=CARTESIAN_POINT('Ctrl Pts',(26.5323455701117,32.2394982626669,0.));
#29504=CARTESIAN_POINT('Ctrl Pts',(26.5323455701117,32.2394982626669,18.));
#29505=CARTESIAN_POINT('Ctrl Pts',(26.5558723200361,32.3376276606981,0.));
#29506=CARTESIAN_POINT('Ctrl Pts',(26.5558723200361,32.3376276606981,18.));
#29507=CARTESIAN_POINT('Ctrl Pts',(26.5788913672813,32.4360159072985,0.));
#29508=CARTESIAN_POINT('Ctrl Pts',(26.5788913672813,32.4360159072985,18.));
#29509=CARTESIAN_POINT('Ctrl Pts',(26.6014055904817,32.5346590925498,0.));
#29510=CARTESIAN_POINT('Ctrl Pts',(26.6014055904817,32.5346590925498,18.));
#29511=CARTESIAN_POINT('Ctrl Pts',(26.6234176311245,32.6335534898935,0.));
#29512=CARTESIAN_POINT('Ctrl Pts',(26.6234176311245,32.6335534898935,18.));
#29513=CARTESIAN_POINT('Ctrl Pts',(26.6449300199763,32.7326954489334,0.));
#29514=CARTESIAN_POINT('Ctrl Pts',(26.6449300199763,32.7326954489334,18.));
#29515=CARTESIAN_POINT('Ctrl Pts',(26.6659453236976,32.8320812678271,0.));
#29516=CARTESIAN_POINT('Ctrl Pts',(26.6659453236976,32.8320812678271,18.));
#29517=CARTESIAN_POINT('Ctrl Pts',(26.6864661988935,32.9317071576181,0.));
#29518=CARTESIAN_POINT('Ctrl Pts',(26.6864661988935,32.9317071576181,18.));
#29519=CARTESIAN_POINT('Ctrl Pts',(26.7064953106254,33.03156933761,0.));
#29520=CARTESIAN_POINT('Ctrl Pts',(26.7064953106254,33.03156933761,18.));
#29521=CARTESIAN_POINT('Ctrl Pts',(26.7260352861619,33.131664100194,0.));
#29522=CARTESIAN_POINT('Ctrl Pts',(26.7260352861619,33.131664100194,18.));
#29523=CARTESIAN_POINT('Ctrl Pts',(26.7450886617884,33.2319878786519,0.));
#29524=CARTESIAN_POINT('Ctrl Pts',(26.7450886617884,33.2319878786519,18.));
#29525=CARTESIAN_POINT('Ctrl Pts',(26.7636578270526,33.3325373307046,0.));
#29526=CARTESIAN_POINT('Ctrl Pts',(26.7636578270526,33.3325373307046,18.));
#29527=CARTESIAN_POINT('Ctrl Pts',(26.7817450041181,33.4333093513694,0.));
#29528=CARTESIAN_POINT('Ctrl Pts',(26.7817450041181,33.4333093513694,18.));
#29529=CARTESIAN_POINT('Ctrl Pts',(26.7993522966985,33.5343009499673,0.));
#29530=CARTESIAN_POINT('Ctrl Pts',(26.7993522966985,33.5343009499673,18.));
#29531=CARTESIAN_POINT('Ctrl Pts',(26.8164817280846,33.6355091508895,0.));
#29532=CARTESIAN_POINT('Ctrl Pts',(26.8164817280846,33.6355091508895,18.));
#29533=CARTESIAN_POINT('Ctrl Pts',(26.8331352836667,33.7369308933173,0.));
#29534=CARTESIAN_POINT('Ctrl Pts',(26.8331352836667,33.7369308933173,18.));
#29535=CARTESIAN_POINT('Ctrl Pts',(26.8493149627661,33.838562905895,0.));
#29536=CARTESIAN_POINT('Ctrl Pts',(26.8493149627661,33.838562905895,18.));
#29537=CARTESIAN_POINT('Ctrl Pts',(26.8650228056313,33.9404016650487,0.));
#29538=CARTESIAN_POINT('Ctrl Pts',(26.8650228056313,33.9404016650487,18.));
#29539=CARTESIAN_POINT('Ctrl Pts',(26.880260834701,34.0424436187397,0.));
#29540=CARTESIAN_POINT('Ctrl Pts',(26.880260834701,34.0424436187397,18.));
#29541=CARTESIAN_POINT('Ctrl Pts',(26.8950310138939,34.1446853651051,0.));
#29542=CARTESIAN_POINT('Ctrl Pts',(26.8950310138939,34.1446853651051,18.));
#29543=CARTESIAN_POINT('Ctrl Pts',(26.9093352037262,34.2471238425419,0.));
#29544=CARTESIAN_POINT('Ctrl Pts',(26.9093352037262,34.2471238425419,18.));
#29545=CARTESIAN_POINT('Ctrl Pts',(26.9231751225177,34.3497565255724,0.));
#29546=CARTESIAN_POINT('Ctrl Pts',(26.9231751225177,34.3497565255724,18.));
#29547=CARTESIAN_POINT('Ctrl Pts',(26.9365523054581,34.4525815829097,0.));
#29548=CARTESIAN_POINT('Ctrl Pts',(26.9365523054581,34.4525815829097,18.));
#29549=CARTESIAN_POINT('Ctrl Pts',(26.9494680440307,34.5555977590573,0.));
#29550=CARTESIAN_POINT('Ctrl Pts',(26.9494680440307,34.5555977590573,18.));
#29551=CARTESIAN_POINT('Ctrl Pts',(26.9594322726214,34.6381629799782,0.));
#29552=CARTESIAN_POINT('Ctrl Pts',(26.9594322726214,34.6381629799782,18.));
#29553=CARTESIAN_POINT('Ctrl Pts',(26.9666985267608,34.700172380686,0.));
#29554=CARTESIAN_POINT('Ctrl Pts',(26.9666985267608,34.700172380686,18.));
#29555=CARTESIAN_POINT('Ctrl Pts',(26.9714507634923,34.7415499619104,0.));
#29556=CARTESIAN_POINT('Ctrl Pts',(26.9714507634923,34.7415499619104,18.));
#29557=CARTESIAN_POINT('Ctrl Pts',(26.9738038986838,34.7622482477091,0.));
#29558=CARTESIAN_POINT('Ctrl Pts',(26.9738038986838,34.7622482477091,18.));
#29559=CARTESIAN_POINT('Ctrl Pts',(24.8345302882955,28.2149191006268,0.));
#29560=CARTESIAN_POINT('Ctrl Pts',(24.8470618363541,28.2291563988796,0.));
#29561=CARTESIAN_POINT('Ctrl Pts',(24.8717258526943,28.2579420132101,0.));
#29562=CARTESIAN_POINT('Ctrl Pts',(24.9075246543798,28.3020534756061,0.));
#29563=CARTESIAN_POINT('Ctrl Pts',(24.9529811166897,28.3626431274892,0.));
#29564=CARTESIAN_POINT('Ctrl Pts',(25.0066999111736,28.4408053900206,0.));
#29565=CARTESIAN_POINT('Ctrl Pts',(25.0581926620043,28.5207164321473,0.));
#29566=CARTESIAN_POINT('Ctrl Pts',(25.1083211582389,28.6017081342376,0.));
#29567=CARTESIAN_POINT('Ctrl Pts',(25.1577170374459,28.6832861366762,0.));
#29568=CARTESIAN_POINT('Ctrl Pts',(25.2066127148845,28.7652594076549,0.));
#29569=CARTESIAN_POINT('Ctrl Pts',(25.2549775629725,28.8476372998748,0.));
#29570=CARTESIAN_POINT('Ctrl Pts',(25.3026235249214,28.9305499160476,0.));
#29571=CARTESIAN_POINT('Ctrl Pts',(25.3493168206005,29.0141637699076,0.));
#29572=CARTESIAN_POINT('Ctrl Pts',(25.3948997321279,29.098589927237,0.));
#29573=CARTESIAN_POINT('Ctrl Pts',(25.4393679214513,29.183825549991,0.));
#29574=CARTESIAN_POINT('Ctrl Pts',(25.4828076101654,29.2698007967907,0.));
#29575=CARTESIAN_POINT('Ctrl Pts',(25.5253562922582,29.356408021119,0.));
#29576=CARTESIAN_POINT('Ctrl Pts',(25.5671572096726,29.443535683207,0.));
#29577=CARTESIAN_POINT('Ctrl Pts',(25.6083094352667,29.5311055094509,0.));
#29578=CARTESIAN_POINT('Ctrl Pts',(25.6488438125835,29.6190903904157,0.));
#29579=CARTESIAN_POINT('Ctrl Pts',(25.6887507922748,29.7074935910931,0.));
#29580=CARTESIAN_POINT('Ctrl Pts',(25.7279973711305,29.7963360859334,0.));
#29581=CARTESIAN_POINT('Ctrl Pts',(25.7665469042913,29.8856417535786,0.));
#29582=CARTESIAN_POINT('Ctrl Pts',(25.8043812318214,29.9754208429384,0.));
#29583=CARTESIAN_POINT('Ctrl Pts',(25.8415089241134,30.0656638016321,0.));
#29584=CARTESIAN_POINT('Ctrl Pts',(25.8779535511027,30.1563500154165,0.));
#29585=CARTESIAN_POINT('Ctrl Pts',(25.9137466853317,30.2474530144827,0.));
#29586=CARTESIAN_POINT('Ctrl Pts',(25.9489196635424,30.3389466074503,0.));
#29587=CARTESIAN_POINT('Ctrl Pts',(25.9834942765902,30.4308118142473,0.));
#29588=CARTESIAN_POINT('Ctrl Pts',(26.0174801292225,30.5230388264271,0.));
#29589=CARTESIAN_POINT('Ctrl Pts',(26.0508796503166,30.6156232634061,0.));
#29590=CARTESIAN_POINT('Ctrl Pts',(26.0836911730968,30.7085638682391,0.));
#29591=CARTESIAN_POINT('Ctrl Pts',(26.1159125093178,30.8018598357461,0.));
#29592=CARTESIAN_POINT('Ctrl Pts',(26.1475450294082,30.8955077633644,0.));
#29593=CARTESIAN_POINT('Ctrl Pts',(26.1785946616165,30.9895009017073,0.));
#29594=CARTESIAN_POINT('Ctrl Pts',(26.2090698085494,31.0838307058369,0.));
#29595=CARTESIAN_POINT('Ctrl Pts',(26.2389800738215,31.1784877826858,0.));
#29596=CARTESIAN_POINT('Ctrl Pts',(26.2683347859175,31.2734629900041,0.));
#29597=CARTESIAN_POINT('Ctrl Pts',(26.2971413115295,31.3687486937246,0.));
#29598=CARTESIAN_POINT('Ctrl Pts',(26.3254046890485,31.4643390378084,0.));
#29599=CARTESIAN_POINT('Ctrl Pts',(26.353128528169,31.5602292672984,0.));
#29600=CARTESIAN_POINT('Ctrl Pts',(26.3803155790949,31.6564152990236,0.));
#29601=CARTESIAN_POINT('Ctrl Pts',(26.4069683862784,31.7528932299312,0.));
#29602=CARTESIAN_POINT('Ctrl Pts',(26.433090040836,31.849658771403,0.));
#29603=CARTESIAN_POINT('Ctrl Pts',(26.4586843683627,31.9467071093816,0.));
#29604=CARTESIAN_POINT('Ctrl Pts',(26.4837555495616,32.0440331917233,0.));
#29605=CARTESIAN_POINT('Ctrl Pts',(26.5083078928862,32.1416319023705,0.));
#29606=CARTESIAN_POINT('Ctrl Pts',(26.5323455701117,32.2394982626669,0.));
#29607=CARTESIAN_POINT('Ctrl Pts',(26.5558723200361,32.3376276606981,0.));
#29608=CARTESIAN_POINT('Ctrl Pts',(26.5788913672813,32.4360159072985,0.));
#29609=CARTESIAN_POINT('Ctrl Pts',(26.6014055904817,32.5346590925498,0.));
#29610=CARTESIAN_POINT('Ctrl Pts',(26.6234176311245,32.6335534898935,0.));
#29611=CARTESIAN_POINT('Ctrl Pts',(26.6449300199763,32.7326954489334,0.));
#29612=CARTESIAN_POINT('Ctrl Pts',(26.6659453236976,32.8320812678271,0.));
#29613=CARTESIAN_POINT('Ctrl Pts',(26.6864661988935,32.9317071576181,0.));
#29614=CARTESIAN_POINT('Ctrl Pts',(26.7064953106254,33.03156933761,0.));
#29615=CARTESIAN_POINT('Ctrl Pts',(26.7260352861619,33.131664100194,0.));
#29616=CARTESIAN_POINT('Ctrl Pts',(26.7450886617884,33.2319878786519,0.));
#29617=CARTESIAN_POINT('Ctrl Pts',(26.7636578270526,33.3325373307046,0.));
#29618=CARTESIAN_POINT('Ctrl Pts',(26.7817450041181,33.4333093513694,0.));
#29619=CARTESIAN_POINT('Ctrl Pts',(26.7993522966985,33.5343009499673,0.));
#29620=CARTESIAN_POINT('Ctrl Pts',(26.8164817280846,33.6355091508895,0.));
#29621=CARTESIAN_POINT('Ctrl Pts',(26.8331352836667,33.7369308933173,0.));
#29622=CARTESIAN_POINT('Ctrl Pts',(26.8493149627661,33.838562905895,0.));
#29623=CARTESIAN_POINT('Ctrl Pts',(26.8650228056313,33.9404016650487,0.));
#29624=CARTESIAN_POINT('Ctrl Pts',(26.880260834701,34.0424436187397,0.));
#29625=CARTESIAN_POINT('Ctrl Pts',(26.8950310138939,34.1446853651051,0.));
#29626=CARTESIAN_POINT('Ctrl Pts',(26.9093352037262,34.2471238425419,0.));
#29627=CARTESIAN_POINT('Ctrl Pts',(26.9231751225177,34.3497565255724,0.));
#29628=CARTESIAN_POINT('Ctrl Pts',(26.9392277420462,34.4731465943772,0.));
#29629=CARTESIAN_POINT('Ctrl Pts',(26.9520281195268,34.5762105502273,0.));
#29630=CARTESIAN_POINT('Ctrl Pts',(26.9619003236529,34.6588137898952,0.));
#29631=CARTESIAN_POINT('Ctrl Pts',(26.9690976283147,34.7208516760814,0.));
#29632=CARTESIAN_POINT('Ctrl Pts',(26.9738038986838,34.7622482477091,0.));
#29633=CARTESIAN_POINT('Ctrl Pts',(24.8345302882955,28.2149191006268,15.));
#29634=CARTESIAN_POINT('Ctrl Pts',(24.8470618363541,28.2291563988796,15.));
#29635=CARTESIAN_POINT('Ctrl Pts',(24.8717258526943,28.2579420132101,15.));
#29636=CARTESIAN_POINT('Ctrl Pts',(24.9075246543798,28.3020534756061,15.));
#29637=CARTESIAN_POINT('Ctrl Pts',(24.9529811166897,28.3626431274892,15.));
#29638=CARTESIAN_POINT('Ctrl Pts',(25.0066999111736,28.4408053900206,15.));
#29639=CARTESIAN_POINT('Ctrl Pts',(25.0581926620043,28.5207164321473,15.));
#29640=CARTESIAN_POINT('Ctrl Pts',(25.1083211582389,28.6017081342376,15.));
#29641=CARTESIAN_POINT('Ctrl Pts',(25.1577170374459,28.6832861366762,15.));
#29642=CARTESIAN_POINT('Ctrl Pts',(25.2066127148845,28.7652594076549,15.));
#29643=CARTESIAN_POINT('Ctrl Pts',(25.2549775629725,28.8476372998748,15.));
#29644=CARTESIAN_POINT('Ctrl Pts',(25.3026235249214,28.9305499160476,15.));
#29645=CARTESIAN_POINT('Ctrl Pts',(25.3493168206005,29.0141637699076,15.));
#29646=CARTESIAN_POINT('Ctrl Pts',(25.3948997321279,29.098589927237,15.));
#29647=CARTESIAN_POINT('Ctrl Pts',(25.4393679214513,29.183825549991,15.));
#29648=CARTESIAN_POINT('Ctrl Pts',(25.4828076101654,29.2698007967907,15.));
#29649=CARTESIAN_POINT('Ctrl Pts',(25.5253562922582,29.356408021119,15.));
#29650=CARTESIAN_POINT('Ctrl Pts',(25.5671572096726,29.443535683207,15.));
#29651=CARTESIAN_POINT('Ctrl Pts',(25.6083094352667,29.5311055094509,15.));
#29652=CARTESIAN_POINT('Ctrl Pts',(25.6488438125835,29.6190903904157,15.));
#29653=CARTESIAN_POINT('Ctrl Pts',(25.6887507922748,29.7074935910931,15.));
#29654=CARTESIAN_POINT('Ctrl Pts',(25.7279973711305,29.7963360859334,15.));
#29655=CARTESIAN_POINT('Ctrl Pts',(25.7665469042913,29.8856417535786,15.));
#29656=CARTESIAN_POINT('Ctrl Pts',(25.8043812318214,29.9754208429384,15.));
#29657=CARTESIAN_POINT('Ctrl Pts',(25.8415089241134,30.0656638016321,15.));
#29658=CARTESIAN_POINT('Ctrl Pts',(25.8779535511027,30.1563500154165,15.));
#29659=CARTESIAN_POINT('Ctrl Pts',(25.9137466853317,30.2474530144827,15.));
#29660=CARTESIAN_POINT('Ctrl Pts',(25.9489196635424,30.3389466074503,15.));
#29661=CARTESIAN_POINT('Ctrl Pts',(25.9834942765902,30.4308118142473,15.));
#29662=CARTESIAN_POINT('Ctrl Pts',(26.0174801292225,30.5230388264271,15.));
#29663=CARTESIAN_POINT('Ctrl Pts',(26.0508796503166,30.6156232634061,15.));
#29664=CARTESIAN_POINT('Ctrl Pts',(26.0836911730968,30.7085638682391,15.));
#29665=CARTESIAN_POINT('Ctrl Pts',(26.1159125093178,30.8018598357461,15.));
#29666=CARTESIAN_POINT('Ctrl Pts',(26.1475450294082,30.8955077633644,15.));
#29667=CARTESIAN_POINT('Ctrl Pts',(26.1785946616165,30.9895009017073,15.));
#29668=CARTESIAN_POINT('Ctrl Pts',(26.2090698085494,31.0838307058369,15.));
#29669=CARTESIAN_POINT('Ctrl Pts',(26.2389800738215,31.1784877826858,15.));
#29670=CARTESIAN_POINT('Ctrl Pts',(26.2683347859175,31.2734629900041,15.));
#29671=CARTESIAN_POINT('Ctrl Pts',(26.2971413115295,31.3687486937246,15.));
#29672=CARTESIAN_POINT('Ctrl Pts',(26.3254046890485,31.4643390378084,15.));
#29673=CARTESIAN_POINT('Ctrl Pts',(26.353128528169,31.5602292672984,15.));
#29674=CARTESIAN_POINT('Ctrl Pts',(26.3803155790949,31.6564152990236,15.));
#29675=CARTESIAN_POINT('Ctrl Pts',(26.4069683862784,31.7528932299312,15.));
#29676=CARTESIAN_POINT('Ctrl Pts',(26.433090040836,31.849658771403,15.));
#29677=CARTESIAN_POINT('Ctrl Pts',(26.4586843683627,31.9467071093816,15.));
#29678=CARTESIAN_POINT('Ctrl Pts',(26.4837555495616,32.0440331917233,15.));
#29679=CARTESIAN_POINT('Ctrl Pts',(26.5083078928862,32.1416319023705,15.));
#29680=CARTESIAN_POINT('Ctrl Pts',(26.5323455701117,32.2394982626669,15.));
#29681=CARTESIAN_POINT('Ctrl Pts',(26.5558723200361,32.3376276606981,15.));
#29682=CARTESIAN_POINT('Ctrl Pts',(26.5788913672813,32.4360159072985,15.));
#29683=CARTESIAN_POINT('Ctrl Pts',(26.6014055904817,32.5346590925498,15.));
#29684=CARTESIAN_POINT('Ctrl Pts',(26.6234176311245,32.6335534898935,15.));
#29685=CARTESIAN_POINT('Ctrl Pts',(26.6449300199763,32.7326954489334,15.));
#29686=CARTESIAN_POINT('Ctrl Pts',(26.6659453236976,32.8320812678271,15.));
#29687=CARTESIAN_POINT('Ctrl Pts',(26.6864661988935,32.9317071576181,15.));
#29688=CARTESIAN_POINT('Ctrl Pts',(26.7064953106254,33.03156933761,15.));
#29689=CARTESIAN_POINT('Ctrl Pts',(26.7260352861619,33.131664100194,15.));
#29690=CARTESIAN_POINT('Ctrl Pts',(26.7450886617884,33.2319878786519,15.));
#29691=CARTESIAN_POINT('Ctrl Pts',(26.7636578270526,33.3325373307046,15.));
#29692=CARTESIAN_POINT('Ctrl Pts',(26.7817450041181,33.4333093513694,15.));
#29693=CARTESIAN_POINT('Ctrl Pts',(26.7993522966985,33.5343009499673,15.));
#29694=CARTESIAN_POINT('Ctrl Pts',(26.8164817280846,33.6355091508895,15.));
#29695=CARTESIAN_POINT('Ctrl Pts',(26.8331352836667,33.7369308933173,15.));
#29696=CARTESIAN_POINT('Ctrl Pts',(26.8493149627661,33.838562905895,15.));
#29697=CARTESIAN_POINT('Ctrl Pts',(26.8650228056313,33.9404016650487,15.));
#29698=CARTESIAN_POINT('Ctrl Pts',(26.880260834701,34.0424436187397,15.));
#29699=CARTESIAN_POINT('Ctrl Pts',(26.8950310138939,34.1446853651051,15.));
#29700=CARTESIAN_POINT('Ctrl Pts',(26.9093352037262,34.2471238425419,15.));
#29701=CARTESIAN_POINT('Ctrl Pts',(26.9231751225177,34.3497565255724,15.));
#29702=CARTESIAN_POINT('Ctrl Pts',(26.9392277420462,34.4731465943772,15.));
#29703=CARTESIAN_POINT('Ctrl Pts',(26.9520281195268,34.5762105502273,15.));
#29704=CARTESIAN_POINT('Ctrl Pts',(26.9619003236529,34.6588137898952,15.));
#29705=CARTESIAN_POINT('Ctrl Pts',(26.9690976283147,34.7208516760814,15.));
#29706=CARTESIAN_POINT('Ctrl Pts',(26.9738038986838,34.7622482477091,15.));
#29707=CARTESIAN_POINT('Ctrl Pts',(34.7622482477091,26.9738038986838,0.));
#29708=CARTESIAN_POINT('Ctrl Pts',(34.7622482477091,26.9738038986838,18.));
#29709=CARTESIAN_POINT('Ctrl Pts',(34.7415499619104,26.9714507634923,0.));
#29710=CARTESIAN_POINT('Ctrl Pts',(34.7415499619104,26.9714507634923,18.));
#29711=CARTESIAN_POINT('Ctrl Pts',(34.700172380686,26.9666985267608,0.));
#29712=CARTESIAN_POINT('Ctrl Pts',(34.700172380686,26.9666985267608,18.));
#29713=CARTESIAN_POINT('Ctrl Pts',(34.6381629799782,26.9594322726214,0.));
#29714=CARTESIAN_POINT('Ctrl Pts',(34.6381629799782,26.9594322726214,18.));
#29715=CARTESIAN_POINT('Ctrl Pts',(34.5555977590573,26.9494680440307,0.));
#29716=CARTESIAN_POINT('Ctrl Pts',(34.5555977590573,26.9494680440307,18.));
#29717=CARTESIAN_POINT('Ctrl Pts',(34.4525815829097,26.936552305458,0.));
#29718=CARTESIAN_POINT('Ctrl Pts',(34.4525815829097,26.936552305458,18.));
#29719=CARTESIAN_POINT('Ctrl Pts',(34.3497565255724,26.9231751225177,0.));
#29720=CARTESIAN_POINT('Ctrl Pts',(34.3497565255724,26.9231751225177,18.));
#29721=CARTESIAN_POINT('Ctrl Pts',(34.2471238425419,26.9093352037262,0.));
#29722=CARTESIAN_POINT('Ctrl Pts',(34.2471238425419,26.9093352037262,18.));
#29723=CARTESIAN_POINT('Ctrl Pts',(34.1446853651051,26.8950310138939,0.));
#29724=CARTESIAN_POINT('Ctrl Pts',(34.1446853651051,26.8950310138939,18.));
#29725=CARTESIAN_POINT('Ctrl Pts',(34.0424436187397,26.880260834701,0.));
#29726=CARTESIAN_POINT('Ctrl Pts',(34.0424436187397,26.880260834701,18.));
#29727=CARTESIAN_POINT('Ctrl Pts',(33.9404016650487,26.8650228056313,0.));
#29728=CARTESIAN_POINT('Ctrl Pts',(33.9404016650487,26.8650228056313,18.));
#29729=CARTESIAN_POINT('Ctrl Pts',(33.838562905895,26.8493149627661,0.));
#29730=CARTESIAN_POINT('Ctrl Pts',(33.838562905895,26.8493149627661,18.));
#29731=CARTESIAN_POINT('Ctrl Pts',(33.7369308933173,26.8331352836666,0.));
#29732=CARTESIAN_POINT('Ctrl Pts',(33.7369308933173,26.8331352836666,18.));
#29733=CARTESIAN_POINT('Ctrl Pts',(33.6355091508895,26.8164817280846,0.));
#29734=CARTESIAN_POINT('Ctrl Pts',(33.6355091508895,26.8164817280846,18.));
#29735=CARTESIAN_POINT('Ctrl Pts',(33.5343009499673,26.7993522966985,0.));
#29736=CARTESIAN_POINT('Ctrl Pts',(33.5343009499673,26.7993522966985,18.));
#29737=CARTESIAN_POINT('Ctrl Pts',(33.4333093513694,26.7817450041181,0.));
#29738=CARTESIAN_POINT('Ctrl Pts',(33.4333093513694,26.7817450041181,18.));
#29739=CARTESIAN_POINT('Ctrl Pts',(33.3325373307046,26.7636578270526,0.));
#29740=CARTESIAN_POINT('Ctrl Pts',(33.3325373307046,26.7636578270526,18.));
#29741=CARTESIAN_POINT('Ctrl Pts',(33.2319878786519,26.7450886617884,0.));
#29742=CARTESIAN_POINT('Ctrl Pts',(33.2319878786519,26.7450886617884,18.));
#29743=CARTESIAN_POINT('Ctrl Pts',(33.131664100194,26.7260352861619,0.));
#29744=CARTESIAN_POINT('Ctrl Pts',(33.131664100194,26.7260352861619,18.));
#29745=CARTESIAN_POINT('Ctrl Pts',(33.03156933761,26.7064953106254,0.));
#29746=CARTESIAN_POINT('Ctrl Pts',(33.03156933761,26.7064953106254,18.));
#29747=CARTESIAN_POINT('Ctrl Pts',(32.9317071576181,26.6864661988935,0.));
#29748=CARTESIAN_POINT('Ctrl Pts',(32.9317071576181,26.6864661988935,18.));
#29749=CARTESIAN_POINT('Ctrl Pts',(32.8320812678271,26.6659453236976,0.));
#29750=CARTESIAN_POINT('Ctrl Pts',(32.8320812678271,26.6659453236976,18.));
#29751=CARTESIAN_POINT('Ctrl Pts',(32.7326954489334,26.6449300199763,0.));
#29752=CARTESIAN_POINT('Ctrl Pts',(32.7326954489334,26.6449300199763,18.));
#29753=CARTESIAN_POINT('Ctrl Pts',(32.6335534898935,26.6234176311244,0.));
#29754=CARTESIAN_POINT('Ctrl Pts',(32.6335534898935,26.6234176311244,18.));
#29755=CARTESIAN_POINT('Ctrl Pts',(32.5346590925498,26.6014055904817,0.));
#29756=CARTESIAN_POINT('Ctrl Pts',(32.5346590925498,26.6014055904817,18.));
#29757=CARTESIAN_POINT('Ctrl Pts',(32.4360159072985,26.5788913672813,0.));
#29758=CARTESIAN_POINT('Ctrl Pts',(32.4360159072985,26.5788913672813,18.));
#29759=CARTESIAN_POINT('Ctrl Pts',(32.3376276606981,26.5558723200361,0.));
#29760=CARTESIAN_POINT('Ctrl Pts',(32.3376276606981,26.5558723200361,18.));
#29761=CARTESIAN_POINT('Ctrl Pts',(32.2394982626669,26.5323455701117,0.));
#29762=CARTESIAN_POINT('Ctrl Pts',(32.2394982626669,26.5323455701117,18.));
#29763=CARTESIAN_POINT('Ctrl Pts',(32.1416319023705,26.5083078928862,0.));
#29764=CARTESIAN_POINT('Ctrl Pts',(32.1416319023705,26.5083078928862,18.));
#29765=CARTESIAN_POINT('Ctrl Pts',(32.0440331917233,26.4837555495616,0.));
#29766=CARTESIAN_POINT('Ctrl Pts',(32.0440331917233,26.4837555495616,18.));
#29767=CARTESIAN_POINT('Ctrl Pts',(31.9467071093816,26.4586843683627,0.));
#29768=CARTESIAN_POINT('Ctrl Pts',(31.9467071093816,26.4586843683627,18.));
#29769=CARTESIAN_POINT('Ctrl Pts',(31.849658771403,26.433090040836,0.));
#29770=CARTESIAN_POINT('Ctrl Pts',(31.849658771403,26.433090040836,18.));
#29771=CARTESIAN_POINT('Ctrl Pts',(31.7528932299312,26.4069683862784,0.));
#29772=CARTESIAN_POINT('Ctrl Pts',(31.7528932299312,26.4069683862784,18.));
#29773=CARTESIAN_POINT('Ctrl Pts',(31.6564152990236,26.3803155790949,0.));
#29774=CARTESIAN_POINT('Ctrl Pts',(31.6564152990236,26.3803155790949,18.));
#29775=CARTESIAN_POINT('Ctrl Pts',(31.5602292672984,26.353128528169,0.));
#29776=CARTESIAN_POINT('Ctrl Pts',(31.5602292672984,26.353128528169,18.));
#29777=CARTESIAN_POINT('Ctrl Pts',(31.4643390378084,26.3254046890485,0.));
#29778=CARTESIAN_POINT('Ctrl Pts',(31.4643390378084,26.3254046890485,18.));
#29779=CARTESIAN_POINT('Ctrl Pts',(31.3687486937246,26.2971413115295,0.));
#29780=CARTESIAN_POINT('Ctrl Pts',(31.3687486937246,26.2971413115295,18.));
#29781=CARTESIAN_POINT('Ctrl Pts',(31.2734629900041,26.2683347859175,0.));
#29782=CARTESIAN_POINT('Ctrl Pts',(31.2734629900041,26.2683347859175,18.));
#29783=CARTESIAN_POINT('Ctrl Pts',(31.1784877826858,26.2389800738215,0.));
#29784=CARTESIAN_POINT('Ctrl Pts',(31.1784877826858,26.2389800738215,18.));
#29785=CARTESIAN_POINT('Ctrl Pts',(31.0838307058369,26.2090698085494,0.));
#29786=CARTESIAN_POINT('Ctrl Pts',(31.0838307058369,26.2090698085494,18.));
#29787=CARTESIAN_POINT('Ctrl Pts',(30.9895009017073,26.1785946616165,0.));
#29788=CARTESIAN_POINT('Ctrl Pts',(30.9895009017073,26.1785946616165,18.));
#29789=CARTESIAN_POINT('Ctrl Pts',(30.8955077633644,26.1475450294082,0.));
#29790=CARTESIAN_POINT('Ctrl Pts',(30.8955077633644,26.1475450294082,18.));
#29791=CARTESIAN_POINT('Ctrl Pts',(30.8018598357461,26.1159125093178,0.));
#29792=CARTESIAN_POINT('Ctrl Pts',(30.8018598357461,26.1159125093178,18.));
#29793=CARTESIAN_POINT('Ctrl Pts',(30.7085638682391,26.0836911730968,0.));
#29794=CARTESIAN_POINT('Ctrl Pts',(30.7085638682391,26.0836911730968,18.));
#29795=CARTESIAN_POINT('Ctrl Pts',(30.6156232634061,26.0508796503166,0.));
#29796=CARTESIAN_POINT('Ctrl Pts',(30.6156232634061,26.0508796503166,18.));
#29797=CARTESIAN_POINT('Ctrl Pts',(30.5230388264271,26.0174801292225,0.));
#29798=CARTESIAN_POINT('Ctrl Pts',(30.5230388264271,26.0174801292225,18.));
#29799=CARTESIAN_POINT('Ctrl Pts',(30.4308118142473,25.9834942765902,0.));
#29800=CARTESIAN_POINT('Ctrl Pts',(30.4308118142473,25.9834942765902,18.));
#29801=CARTESIAN_POINT('Ctrl Pts',(30.3389466074503,25.9489196635424,0.));
#29802=CARTESIAN_POINT('Ctrl Pts',(30.3389466074503,25.9489196635424,18.));
#29803=CARTESIAN_POINT('Ctrl Pts',(30.2474530144827,25.9137466853317,0.));
#29804=CARTESIAN_POINT('Ctrl Pts',(30.2474530144827,25.9137466853317,18.));
#29805=CARTESIAN_POINT('Ctrl Pts',(30.1563500154165,25.8779535511027,0.));
#29806=CARTESIAN_POINT('Ctrl Pts',(30.1563500154165,25.8779535511027,18.));
#29807=CARTESIAN_POINT('Ctrl Pts',(30.0656638016321,25.8415089241134,0.));
#29808=CARTESIAN_POINT('Ctrl Pts',(30.0656638016321,25.8415089241134,18.));
#29809=CARTESIAN_POINT('Ctrl Pts',(29.9754208429384,25.8043812318214,0.));
#29810=CARTESIAN_POINT('Ctrl Pts',(29.9754208429384,25.8043812318214,18.));
#29811=CARTESIAN_POINT('Ctrl Pts',(29.8856417535786,25.7665469042913,0.));
#29812=CARTESIAN_POINT('Ctrl Pts',(29.8856417535786,25.7665469042913,18.));
#29813=CARTESIAN_POINT('Ctrl Pts',(29.7963360859334,25.7279973711305,0.));
#29814=CARTESIAN_POINT('Ctrl Pts',(29.7963360859334,25.7279973711305,18.));
#29815=CARTESIAN_POINT('Ctrl Pts',(29.7074935910931,25.6887507922748,0.));
#29816=CARTESIAN_POINT('Ctrl Pts',(29.7074935910931,25.6887507922748,18.));
#29817=CARTESIAN_POINT('Ctrl Pts',(29.6190903904157,25.6488438125835,0.));
#29818=CARTESIAN_POINT('Ctrl Pts',(29.6190903904157,25.6488438125835,18.));
#29819=CARTESIAN_POINT('Ctrl Pts',(29.5311055094509,25.6083094352667,0.));
#29820=CARTESIAN_POINT('Ctrl Pts',(29.5311055094509,25.6083094352667,18.));
#29821=CARTESIAN_POINT('Ctrl Pts',(29.443535683207,25.5671572096726,0.));
#29822=CARTESIAN_POINT('Ctrl Pts',(29.443535683207,25.5671572096726,18.));
#29823=CARTESIAN_POINT('Ctrl Pts',(29.356408021119,25.5253562922582,0.));
#29824=CARTESIAN_POINT('Ctrl Pts',(29.356408021119,25.5253562922582,18.));
#29825=CARTESIAN_POINT('Ctrl Pts',(29.2698007967907,25.4828076101654,0.));
#29826=CARTESIAN_POINT('Ctrl Pts',(29.2698007967907,25.4828076101654,18.));
#29827=CARTESIAN_POINT('Ctrl Pts',(29.183825549991,25.4393679214513,0.));
#29828=CARTESIAN_POINT('Ctrl Pts',(29.183825549991,25.4393679214513,18.));
#29829=CARTESIAN_POINT('Ctrl Pts',(29.098589927237,25.3948997321279,0.));
#29830=CARTESIAN_POINT('Ctrl Pts',(29.098589927237,25.3948997321279,18.));
#29831=CARTESIAN_POINT('Ctrl Pts',(29.0141637699076,25.3493168206005,0.));
#29832=CARTESIAN_POINT('Ctrl Pts',(29.0141637699076,25.3493168206005,18.));
#29833=CARTESIAN_POINT('Ctrl Pts',(28.9305499160476,25.3026235249214,0.));
#29834=CARTESIAN_POINT('Ctrl Pts',(28.9305499160476,25.3026235249214,18.));
#29835=CARTESIAN_POINT('Ctrl Pts',(28.8476372998748,25.2549775629725,0.));
#29836=CARTESIAN_POINT('Ctrl Pts',(28.8476372998748,25.2549775629725,18.));
#29837=CARTESIAN_POINT('Ctrl Pts',(28.7652594076549,25.2066127148845,0.));
#29838=CARTESIAN_POINT('Ctrl Pts',(28.7652594076549,25.2066127148845,18.));
#29839=CARTESIAN_POINT('Ctrl Pts',(28.6832861366762,25.1577170374459,0.));
#29840=CARTESIAN_POINT('Ctrl Pts',(28.6832861366762,25.1577170374459,18.));
#29841=CARTESIAN_POINT('Ctrl Pts',(28.6017081342376,25.1083211582389,0.));
#29842=CARTESIAN_POINT('Ctrl Pts',(28.6017081342376,25.1083211582389,18.));
#29843=CARTESIAN_POINT('Ctrl Pts',(28.5207164321473,25.0581926620043,0.));
#29844=CARTESIAN_POINT('Ctrl Pts',(28.5207164321473,25.0581926620043,18.));
#29845=CARTESIAN_POINT('Ctrl Pts',(28.4408053900206,25.0066999111736,0.));
#29846=CARTESIAN_POINT('Ctrl Pts',(28.4408053900206,25.0066999111736,18.));
#29847=CARTESIAN_POINT('Ctrl Pts',(28.3626431274892,24.9529811166897,0.));
#29848=CARTESIAN_POINT('Ctrl Pts',(28.3626431274892,24.9529811166897,18.));
#29849=CARTESIAN_POINT('Ctrl Pts',(28.3020534756061,24.9075246543798,0.));
#29850=CARTESIAN_POINT('Ctrl Pts',(28.3020534756061,24.9075246543798,18.));
#29851=CARTESIAN_POINT('Ctrl Pts',(28.2579420132101,24.8717258526943,0.));
#29852=CARTESIAN_POINT('Ctrl Pts',(28.2579420132101,24.8717258526943,18.));
#29853=CARTESIAN_POINT('Ctrl Pts',(28.2291563988796,24.8470618363541,0.));
#29854=CARTESIAN_POINT('Ctrl Pts',(28.2291563988796,24.8470618363541,18.));
#29855=CARTESIAN_POINT('Ctrl Pts',(28.2149191006269,24.8345302882955,0.));
#29856=CARTESIAN_POINT('Ctrl Pts',(28.2149191006269,24.8345302882955,18.));
#29857=CARTESIAN_POINT('',(34.762248247709,26.9738038986839,0.));
#29858=CARTESIAN_POINT('Ctrl Pts',(28.2149191006269,24.8345302882955,0.));
#29859=CARTESIAN_POINT('Ctrl Pts',(28.2291563988796,24.8470618363541,0.));
#29860=CARTESIAN_POINT('Ctrl Pts',(28.2579420132101,24.8717258526943,0.));
#29861=CARTESIAN_POINT('Ctrl Pts',(28.3020534756061,24.9075246543798,0.));
#29862=CARTESIAN_POINT('Ctrl Pts',(28.3626431274892,24.9529811166897,0.));
#29863=CARTESIAN_POINT('Ctrl Pts',(28.4408053900206,25.0066999111736,0.));
#29864=CARTESIAN_POINT('Ctrl Pts',(28.5207164321473,25.0581926620043,0.));
#29865=CARTESIAN_POINT('Ctrl Pts',(28.6017081342376,25.1083211582389,0.));
#29866=CARTESIAN_POINT('Ctrl Pts',(28.6832861366762,25.1577170374459,0.));
#29867=CARTESIAN_POINT('Ctrl Pts',(28.7652594076549,25.2066127148845,0.));
#29868=CARTESIAN_POINT('Ctrl Pts',(28.8476372998748,25.2549775629725,0.));
#29869=CARTESIAN_POINT('Ctrl Pts',(28.9305499160476,25.3026235249214,0.));
#29870=CARTESIAN_POINT('Ctrl Pts',(29.0141637699076,25.3493168206005,0.));
#29871=CARTESIAN_POINT('Ctrl Pts',(29.098589927237,25.3948997321279,0.));
#29872=CARTESIAN_POINT('Ctrl Pts',(29.183825549991,25.4393679214513,0.));
#29873=CARTESIAN_POINT('Ctrl Pts',(29.2698007967907,25.4828076101654,0.));
#29874=CARTESIAN_POINT('Ctrl Pts',(29.356408021119,25.5253562922582,0.));
#29875=CARTESIAN_POINT('Ctrl Pts',(29.443535683207,25.5671572096726,0.));
#29876=CARTESIAN_POINT('Ctrl Pts',(29.5311055094509,25.6083094352667,0.));
#29877=CARTESIAN_POINT('Ctrl Pts',(29.6190903904157,25.6488438125835,0.));
#29878=CARTESIAN_POINT('Ctrl Pts',(29.7074935910931,25.6887507922748,0.));
#29879=CARTESIAN_POINT('Ctrl Pts',(29.7963360859334,25.7279973711305,0.));
#29880=CARTESIAN_POINT('Ctrl Pts',(29.8856417535786,25.7665469042913,0.));
#29881=CARTESIAN_POINT('Ctrl Pts',(29.9754208429384,25.8043812318214,0.));
#29882=CARTESIAN_POINT('Ctrl Pts',(30.0656638016321,25.8415089241134,0.));
#29883=CARTESIAN_POINT('Ctrl Pts',(30.1563500154165,25.8779535511027,0.));
#29884=CARTESIAN_POINT('Ctrl Pts',(30.2474530144827,25.9137466853317,0.));
#29885=CARTESIAN_POINT('Ctrl Pts',(30.3389466074503,25.9489196635424,0.));
#29886=CARTESIAN_POINT('Ctrl Pts',(30.4308118142473,25.9834942765902,0.));
#29887=CARTESIAN_POINT('Ctrl Pts',(30.5230388264271,26.0174801292225,0.));
#29888=CARTESIAN_POINT('Ctrl Pts',(30.6156232634061,26.0508796503166,0.));
#29889=CARTESIAN_POINT('Ctrl Pts',(30.7085638682391,26.0836911730968,0.));
#29890=CARTESIAN_POINT('Ctrl Pts',(30.8018598357461,26.1159125093178,0.));
#29891=CARTESIAN_POINT('Ctrl Pts',(30.8955077633644,26.1475450294082,0.));
#29892=CARTESIAN_POINT('Ctrl Pts',(30.9895009017073,26.1785946616165,0.));
#29893=CARTESIAN_POINT('Ctrl Pts',(31.0838307058369,26.2090698085494,0.));
#29894=CARTESIAN_POINT('Ctrl Pts',(31.1784877826858,26.2389800738215,0.));
#29895=CARTESIAN_POINT('Ctrl Pts',(31.2734629900041,26.2683347859175,0.));
#29896=CARTESIAN_POINT('Ctrl Pts',(31.3687486937246,26.2971413115295,0.));
#29897=CARTESIAN_POINT('Ctrl Pts',(31.4643390378084,26.3254046890485,0.));
#29898=CARTESIAN_POINT('Ctrl Pts',(31.5602292672984,26.353128528169,0.));
#29899=CARTESIAN_POINT('Ctrl Pts',(31.6564152990236,26.3803155790949,0.));
#29900=CARTESIAN_POINT('Ctrl Pts',(31.7528932299312,26.4069683862784,0.));
#29901=CARTESIAN_POINT('Ctrl Pts',(31.849658771403,26.433090040836,0.));
#29902=CARTESIAN_POINT('Ctrl Pts',(31.9467071093816,26.4586843683627,0.));
#29903=CARTESIAN_POINT('Ctrl Pts',(32.0440331917233,26.4837555495616,0.));
#29904=CARTESIAN_POINT('Ctrl Pts',(32.1416319023705,26.5083078928862,0.));
#29905=CARTESIAN_POINT('Ctrl Pts',(32.2394982626669,26.5323455701117,0.));
#29906=CARTESIAN_POINT('Ctrl Pts',(32.3376276606981,26.5558723200361,0.));
#29907=CARTESIAN_POINT('Ctrl Pts',(32.4360159072985,26.5788913672813,0.));
#29908=CARTESIAN_POINT('Ctrl Pts',(32.5346590925498,26.6014055904817,0.));
#29909=CARTESIAN_POINT('Ctrl Pts',(32.6335534898935,26.6234176311244,0.));
#29910=CARTESIAN_POINT('Ctrl Pts',(32.7326954489334,26.6449300199763,0.));
#29911=CARTESIAN_POINT('Ctrl Pts',(32.8320812678271,26.6659453236976,0.));
#29912=CARTESIAN_POINT('Ctrl Pts',(32.9317071576181,26.6864661988935,0.));
#29913=CARTESIAN_POINT('Ctrl Pts',(33.03156933761,26.7064953106254,0.));
#29914=CARTESIAN_POINT('Ctrl Pts',(33.131664100194,26.7260352861619,0.));
#29915=CARTESIAN_POINT('Ctrl Pts',(33.2319878786519,26.7450886617884,0.));
#29916=CARTESIAN_POINT('Ctrl Pts',(33.3325373307046,26.7636578270526,0.));
#29917=CARTESIAN_POINT('Ctrl Pts',(33.4333093513694,26.7817450041181,0.));
#29918=CARTESIAN_POINT('Ctrl Pts',(33.5343009499673,26.7993522966985,0.));
#29919=CARTESIAN_POINT('Ctrl Pts',(33.6355091508895,26.8164817280846,0.));
#29920=CARTESIAN_POINT('Ctrl Pts',(33.7369308933173,26.8331352836666,0.));
#29921=CARTESIAN_POINT('Ctrl Pts',(33.838562905895,26.8493149627661,0.));
#29922=CARTESIAN_POINT('Ctrl Pts',(33.9404016650487,26.8650228056313,0.));
#29923=CARTESIAN_POINT('Ctrl Pts',(34.0424436187397,26.880260834701,0.));
#29924=CARTESIAN_POINT('Ctrl Pts',(34.1446853651051,26.8950310138939,0.));
#29925=CARTESIAN_POINT('Ctrl Pts',(34.2471238425419,26.9093352037262,0.));
#29926=CARTESIAN_POINT('Ctrl Pts',(34.3497565255724,26.9231751225177,0.));
#29927=CARTESIAN_POINT('Ctrl Pts',(34.4731465943772,26.9392277420461,0.));
#29928=CARTESIAN_POINT('Ctrl Pts',(34.5762105502273,26.9520281195269,0.));
#29929=CARTESIAN_POINT('Ctrl Pts',(34.6588137898952,26.9619003236529,0.));
#29930=CARTESIAN_POINT('Ctrl Pts',(34.7208516760814,26.9690976283147,0.));
#29931=CARTESIAN_POINT('Ctrl Pts',(34.7622482477091,26.9738038986838,0.));
#29932=CARTESIAN_POINT('',(34.762248247709,26.9738038986839,15.));
#29933=CARTESIAN_POINT('Ctrl Pts',(34.7622482477091,26.9738038986838,15.));
#29934=CARTESIAN_POINT('Ctrl Pts',(34.7415499619104,26.9714507634923,15.));
#29935=CARTESIAN_POINT('Ctrl Pts',(34.700172380686,26.9666985267608,15.));
#29936=CARTESIAN_POINT('Ctrl Pts',(34.6381629799782,26.9594322726214,15.));
#29937=CARTESIAN_POINT('Ctrl Pts',(34.5555977590573,26.9494680440307,15.));
#29938=CARTESIAN_POINT('Ctrl Pts',(34.4525815829097,26.936552305458,15.));
#29939=CARTESIAN_POINT('Ctrl Pts',(34.3497565255724,26.9231751225177,15.));
#29940=CARTESIAN_POINT('Ctrl Pts',(34.2471238425419,26.9093352037262,15.));
#29941=CARTESIAN_POINT('Ctrl Pts',(34.1446853651051,26.8950310138939,15.));
#29942=CARTESIAN_POINT('Ctrl Pts',(34.0424436187397,26.880260834701,15.));
#29943=CARTESIAN_POINT('Ctrl Pts',(33.9404016650487,26.8650228056313,15.));
#29944=CARTESIAN_POINT('Ctrl Pts',(33.838562905895,26.8493149627661,15.));
#29945=CARTESIAN_POINT('Ctrl Pts',(33.7369308933173,26.8331352836666,15.));
#29946=CARTESIAN_POINT('Ctrl Pts',(33.6355091508895,26.8164817280846,15.));
#29947=CARTESIAN_POINT('Ctrl Pts',(33.5343009499673,26.7993522966985,15.));
#29948=CARTESIAN_POINT('Ctrl Pts',(33.4333093513694,26.7817450041181,15.));
#29949=CARTESIAN_POINT('Ctrl Pts',(33.3325373307046,26.7636578270526,15.));
#29950=CARTESIAN_POINT('Ctrl Pts',(33.2319878786519,26.7450886617884,15.));
#29951=CARTESIAN_POINT('Ctrl Pts',(33.131664100194,26.7260352861619,15.));
#29952=CARTESIAN_POINT('Ctrl Pts',(33.03156933761,26.7064953106254,15.));
#29953=CARTESIAN_POINT('Ctrl Pts',(32.9317071576181,26.6864661988935,15.));
#29954=CARTESIAN_POINT('Ctrl Pts',(32.8320812678271,26.6659453236976,15.));
#29955=CARTESIAN_POINT('Ctrl Pts',(32.7326954489334,26.6449300199763,15.));
#29956=CARTESIAN_POINT('Ctrl Pts',(32.6335534898935,26.6234176311244,15.));
#29957=CARTESIAN_POINT('Ctrl Pts',(32.5346590925498,26.6014055904817,15.));
#29958=CARTESIAN_POINT('Ctrl Pts',(32.4360159072985,26.5788913672813,15.));
#29959=CARTESIAN_POINT('Ctrl Pts',(32.3376276606981,26.5558723200361,15.));
#29960=CARTESIAN_POINT('Ctrl Pts',(32.2394982626669,26.5323455701117,15.));
#29961=CARTESIAN_POINT('Ctrl Pts',(32.1416319023705,26.5083078928862,15.));
#29962=CARTESIAN_POINT('Ctrl Pts',(32.0440331917233,26.4837555495616,15.));
#29963=CARTESIAN_POINT('Ctrl Pts',(31.9467071093816,26.4586843683627,15.));
#29964=CARTESIAN_POINT('Ctrl Pts',(31.849658771403,26.433090040836,15.));
#29965=CARTESIAN_POINT('Ctrl Pts',(31.7528932299312,26.4069683862784,15.));
#29966=CARTESIAN_POINT('Ctrl Pts',(31.6564152990236,26.3803155790949,15.));
#29967=CARTESIAN_POINT('Ctrl Pts',(31.5602292672984,26.353128528169,15.));
#29968=CARTESIAN_POINT('Ctrl Pts',(31.4643390378084,26.3254046890485,15.));
#29969=CARTESIAN_POINT('Ctrl Pts',(31.3687486937246,26.2971413115295,15.));
#29970=CARTESIAN_POINT('Ctrl Pts',(31.2734629900041,26.2683347859175,15.));
#29971=CARTESIAN_POINT('Ctrl Pts',(31.1784877826858,26.2389800738215,15.));
#29972=CARTESIAN_POINT('Ctrl Pts',(31.0838307058369,26.2090698085494,15.));
#29973=CARTESIAN_POINT('Ctrl Pts',(30.9895009017073,26.1785946616165,15.));
#29974=CARTESIAN_POINT('Ctrl Pts',(30.8955077633644,26.1475450294082,15.));
#29975=CARTESIAN_POINT('Ctrl Pts',(30.8018598357461,26.1159125093178,15.));
#29976=CARTESIAN_POINT('Ctrl Pts',(30.7085638682391,26.0836911730968,15.));
#29977=CARTESIAN_POINT('Ctrl Pts',(30.6156232634061,26.0508796503166,15.));
#29978=CARTESIAN_POINT('Ctrl Pts',(30.5230388264271,26.0174801292225,15.));
#29979=CARTESIAN_POINT('Ctrl Pts',(30.4308118142473,25.9834942765902,15.));
#29980=CARTESIAN_POINT('Ctrl Pts',(30.3389466074503,25.9489196635424,15.));
#29981=CARTESIAN_POINT('Ctrl Pts',(30.2474530144827,25.9137466853317,15.));
#29982=CARTESIAN_POINT('Ctrl Pts',(30.1563500154165,25.8779535511027,15.));
#29983=CARTESIAN_POINT('Ctrl Pts',(30.0656638016321,25.8415089241134,15.));
#29984=CARTESIAN_POINT('Ctrl Pts',(29.9754208429384,25.8043812318214,15.));
#29985=CARTESIAN_POINT('Ctrl Pts',(29.8856417535786,25.7665469042913,15.));
#29986=CARTESIAN_POINT('Ctrl Pts',(29.7963360859334,25.7279973711305,15.));
#29987=CARTESIAN_POINT('Ctrl Pts',(29.7074935910931,25.6887507922748,15.));
#29988=CARTESIAN_POINT('Ctrl Pts',(29.6190903904157,25.6488438125835,15.));
#29989=CARTESIAN_POINT('Ctrl Pts',(29.5311055094509,25.6083094352667,15.));
#29990=CARTESIAN_POINT('Ctrl Pts',(29.443535683207,25.5671572096726,15.));
#29991=CARTESIAN_POINT('Ctrl Pts',(29.356408021119,25.5253562922582,15.));
#29992=CARTESIAN_POINT('Ctrl Pts',(29.2698007967907,25.4828076101654,15.));
#29993=CARTESIAN_POINT('Ctrl Pts',(29.183825549991,25.4393679214513,15.));
#29994=CARTESIAN_POINT('Ctrl Pts',(29.098589927237,25.3948997321279,15.));
#29995=CARTESIAN_POINT('Ctrl Pts',(29.0141637699076,25.3493168206005,15.));
#29996=CARTESIAN_POINT('Ctrl Pts',(28.9305499160476,25.3026235249214,15.));
#29997=CARTESIAN_POINT('Ctrl Pts',(28.8476372998748,25.2549775629725,15.));
#29998=CARTESIAN_POINT('Ctrl Pts',(28.7652594076549,25.2066127148845,15.));
#29999=CARTESIAN_POINT('Ctrl Pts',(28.6832861366762,25.1577170374459,15.));
#30000=CARTESIAN_POINT('Ctrl Pts',(28.6017081342376,25.1083211582389,15.));
#30001=CARTESIAN_POINT('Ctrl Pts',(28.5207164321473,25.0581926620043,15.));
#30002=CARTESIAN_POINT('Ctrl Pts',(28.4408053900206,25.0066999111736,15.));
#30003=CARTESIAN_POINT('Ctrl Pts',(28.3626431274892,24.9529811166897,15.));
#30004=CARTESIAN_POINT('Ctrl Pts',(28.3020534756061,24.9075246543798,15.));
#30005=CARTESIAN_POINT('Ctrl Pts',(28.2579420132101,24.8717258526943,15.));
#30006=CARTESIAN_POINT('Ctrl Pts',(28.2291563988796,24.8470618363541,15.));
#30007=CARTESIAN_POINT('Ctrl Pts',(28.2149191006269,24.8345302882955,15.));
#30008=CARTESIAN_POINT('',(34.762248247709,26.9738038986839,0.));
#30009=CARTESIAN_POINT('Origin',(9.16871631793044E-12,6.66146233219319E-12,
0.));
#30010=CARTESIAN_POINT('',(36.3957374383337,24.725498909423,0.));
#30011=CARTESIAN_POINT('Origin',(9.16871631793044E-12,6.66146233219319E-12,
0.));
#30012=CARTESIAN_POINT('',(36.3957374383337,24.725498909423,15.));
#30013=CARTESIAN_POINT('Origin',(9.16871631793044E-12,6.66146233219319E-12,
15.));
#30014=CARTESIAN_POINT('',(36.3957374383337,24.725498909423,0.));
#30015=CARTESIAN_POINT('Ctrl Pts',(32.3379313568208,19.1596907609891,0.));
#30016=CARTESIAN_POINT('Ctrl Pts',(32.3379313568208,19.1596907609891,18.));
#30017=CARTESIAN_POINT('Ctrl Pts',(32.3542491343753,19.1693587749508,0.));
#30018=CARTESIAN_POINT('Ctrl Pts',(32.3542491343753,19.1693587749508,18.));
#30019=CARTESIAN_POINT('Ctrl Pts',(32.3866012518553,19.1891139208368,0.));
#30020=CARTESIAN_POINT('Ctrl Pts',(32.3866012518553,19.1891139208368,18.));
#30021=CARTESIAN_POINT('Ctrl Pts',(32.4342791270009,19.2200039764927,0.));
#30022=CARTESIAN_POINT('Ctrl Pts',(32.4342791270009,19.2200039764927,18.));
#30023=CARTESIAN_POINT('Ctrl Pts',(32.4962340238036,19.2635813403783,0.));
#30024=CARTESIAN_POINT('Ctrl Pts',(32.4962340238036,19.2635813403783,18.));
#30025=CARTESIAN_POINT('Ctrl Pts',(32.5714771007861,19.3213180490743,0.));
#30026=CARTESIAN_POINT('Ctrl Pts',(32.5714771007861,19.3213180490743,18.));
#30027=CARTESIAN_POINT('Ctrl Pts',(32.6451434870609,19.381405831319,0.));
#30028=CARTESIAN_POINT('Ctrl Pts',(32.6451434870609,19.381405831319,18.));
#30029=CARTESIAN_POINT('Ctrl Pts',(32.7178463324062,19.4429429601189,0.));
#30030=CARTESIAN_POINT('Ctrl Pts',(32.7178463324062,19.4429429601189,18.));
#30031=CARTESIAN_POINT('Ctrl Pts',(32.7900335943248,19.5052640847974,0.));
#30032=CARTESIAN_POINT('Ctrl Pts',(32.7900335943248,19.5052640847974,18.));
#30033=CARTESIAN_POINT('Ctrl Pts',(32.8618672807884,19.5681157030437,0.));
#30034=CARTESIAN_POINT('Ctrl Pts',(32.8618672807884,19.5681157030437,18.));
#30035=CARTESIAN_POINT('Ctrl Pts',(32.9333211533788,19.6315161742485,0.));
#30036=CARTESIAN_POINT('Ctrl Pts',(32.9333211533788,19.6315161742485,18.));
#30037=CARTESIAN_POINT('Ctrl Pts',(33.004256563411,19.6956473461873,0.));
#30038=CARTESIAN_POINT('Ctrl Pts',(33.004256563411,19.6956473461873,18.));
#30039=CARTESIAN_POINT('Ctrl Pts',(33.0745026283418,19.7607398248651,0.));
#30040=CARTESIAN_POINT('Ctrl Pts',(33.0745026283418,19.7607398248651,18.));
#30041=CARTESIAN_POINT('Ctrl Pts',(33.1439436707661,19.8269479776239,0.));
#30042=CARTESIAN_POINT('Ctrl Pts',(33.1439436707661,19.8269479776239,18.));
#30043=CARTESIAN_POINT('Ctrl Pts',(33.2125746879471,19.8942704458546,0.));
#30044=CARTESIAN_POINT('Ctrl Pts',(33.2125746879471,19.8942704458546,18.));
#30045=CARTESIAN_POINT('Ctrl Pts',(33.2804560993213,19.9626141625205,0.));
#30046=CARTESIAN_POINT('Ctrl Pts',(33.2804560993213,19.9626141625205,18.));
#30047=CARTESIAN_POINT('Ctrl Pts',(33.3476854048385,20.0318342617212,0.));
#30048=CARTESIAN_POINT('Ctrl Pts',(33.3476854048385,20.0318342617212,18.));
#30049=CARTESIAN_POINT('Ctrl Pts',(33.4143643679979,20.1017803986381,0.));
#30050=CARTESIAN_POINT('Ctrl Pts',(33.4143643679979,20.1017803986381,18.));
#30051=CARTESIAN_POINT('Ctrl Pts',(33.480563024813,20.1723475154533,0.));
#30052=CARTESIAN_POINT('Ctrl Pts',(33.480563024813,20.1723475154533,18.));
#30053=CARTESIAN_POINT('Ctrl Pts',(33.5463023319603,20.243500298383,0.));
#30054=CARTESIAN_POINT('Ctrl Pts',(33.5463023319603,20.243500298383,18.));
#30055=CARTESIAN_POINT('Ctrl Pts',(33.6115742164079,20.3152448035298,0.));
#30056=CARTESIAN_POINT('Ctrl Pts',(33.6115742164079,20.3152448035298,18.));
#30057=CARTESIAN_POINT('Ctrl Pts',(33.6763537716992,20.3876111773341,0.));
#30058=CARTESIAN_POINT('Ctrl Pts',(33.6763537716992,20.3876111773341,18.));
#30059=CARTESIAN_POINT('Ctrl Pts',(33.7406135254082,20.4606334536183,0.));
#30060=CARTESIAN_POINT('Ctrl Pts',(33.7406135254082,20.4606334536183,18.));
#30061=CARTESIAN_POINT('Ctrl Pts',(33.8043393734971,20.5343269914034,0.));
#30062=CARTESIAN_POINT('Ctrl Pts',(33.8043393734971,20.5343269914034,18.));
#30063=CARTESIAN_POINT('Ctrl Pts',(33.8675365150454,20.6086800574386,0.));
#30064=CARTESIAN_POINT('Ctrl Pts',(33.8675365150454,20.6086800574386,18.));
#30065=CARTESIAN_POINT('Ctrl Pts',(33.9302209962425,20.683665762903,0.));
#30066=CARTESIAN_POINT('Ctrl Pts',(33.9302209962425,20.683665762903,18.));
#30067=CARTESIAN_POINT('Ctrl Pts',(33.9924146647395,20.7592491770603,0.));
#30068=CARTESIAN_POINT('Ctrl Pts',(33.9924146647395,20.7592491770603,18.));
#30069=CARTESIAN_POINT('Ctrl Pts',(34.0541392299678,20.8353957068415,0.));
#30070=CARTESIAN_POINT('Ctrl Pts',(34.0541392299678,20.8353957068415,18.));
#30071=CARTESIAN_POINT('Ctrl Pts',(34.1154095510973,20.9120805673809,0.));
#30072=CARTESIAN_POINT('Ctrl Pts',(34.1154095510973,20.9120805673809,18.));
#30073=CARTESIAN_POINT('Ctrl Pts',(34.176231731809,20.9892914622612,0.));
#30074=CARTESIAN_POINT('Ctrl Pts',(34.176231731809,20.9892914622612,18.));
#30075=CARTESIAN_POINT('Ctrl Pts',(34.2366067284279,21.0670234747355,0.));
#30076=CARTESIAN_POINT('Ctrl Pts',(34.2366067284279,21.0670234747355,18.));
#30077=CARTESIAN_POINT('Ctrl Pts',(34.2965325673384,21.1452759244399,0.));
#30078=CARTESIAN_POINT('Ctrl Pts',(34.2965325673384,21.1452759244399,18.));
#30079=CARTESIAN_POINT('Ctrl Pts',(34.3560069185815,21.2240487218079,0.));
#30080=CARTESIAN_POINT('Ctrl Pts',(34.3560069185815,21.2240487218079,18.));
#30081=CARTESIAN_POINT('Ctrl Pts',(34.4150300340623,21.3033382073239,0.));
#30082=CARTESIAN_POINT('Ctrl Pts',(34.4150300340623,21.3033382073239,18.));
#30083=CARTESIAN_POINT('Ctrl Pts',(34.4736054662052,21.3831361300104,0.));
#30084=CARTESIAN_POINT('Ctrl Pts',(34.4736054662052,21.3831361300104,18.));
#30085=CARTESIAN_POINT('Ctrl Pts',(34.5317385658329,21.4634317666005,0.));
#30086=CARTESIAN_POINT('Ctrl Pts',(34.5317385658329,21.4634317666005,18.));
#30087=CARTESIAN_POINT('Ctrl Pts',(34.5894355639082,21.5442132160757,0.));
#30088=CARTESIAN_POINT('Ctrl Pts',(34.5894355639082,21.5442132160757,18.));
#30089=CARTESIAN_POINT('Ctrl Pts',(34.6467025072367,21.6254689009796,0.));
#30090=CARTESIAN_POINT('Ctrl Pts',(34.6467025072367,21.6254689009796,18.));
#30091=CARTESIAN_POINT('Ctrl Pts',(34.7035440429025,21.7071892844497,0.));
#30092=CARTESIAN_POINT('Ctrl Pts',(34.7035440429025,21.7071892844497,18.));
#30093=CARTESIAN_POINT('Ctrl Pts',(34.7599631530844,21.7893672401137,0.));
#30094=CARTESIAN_POINT('Ctrl Pts',(34.7599631530844,21.7893672401137,18.));
#30095=CARTESIAN_POINT('Ctrl Pts',(34.8159618014436,21.8719971302817,0.));
#30096=CARTESIAN_POINT('Ctrl Pts',(34.8159618014436,21.8719971302817,18.));
#30097=CARTESIAN_POINT('Ctrl Pts',(34.8715413418101,21.9550742217675,0.));
#30098=CARTESIAN_POINT('Ctrl Pts',(34.8715413418101,21.9550742217675,18.));
#30099=CARTESIAN_POINT('Ctrl Pts',(34.9267029879922,22.0385940162683,0.));
#30100=CARTESIAN_POINT('Ctrl Pts',(34.9267029879922,22.0385940162683,18.));
#30101=CARTESIAN_POINT('Ctrl Pts',(34.9814483545602,22.1225514798584,0.));
#30102=CARTESIAN_POINT('Ctrl Pts',(34.9814483545602,22.1225514798584,18.));
#30103=CARTESIAN_POINT('Ctrl Pts',(35.0357795922459,22.2069408519232,0.));
#30104=CARTESIAN_POINT('Ctrl Pts',(35.0357795922459,22.2069408519232,18.));
#30105=CARTESIAN_POINT('Ctrl Pts',(35.0896991159359,22.2917560356803,0.));
#30106=CARTESIAN_POINT('Ctrl Pts',(35.0896991159359,22.2917560356803,18.));
#30107=CARTESIAN_POINT('Ctrl Pts',(35.1432094422642,22.3769908340843,0.));
#30108=CARTESIAN_POINT('Ctrl Pts',(35.1432094422642,22.3769908340843,18.));
#30109=CARTESIAN_POINT('Ctrl Pts',(35.1963130003352,22.4626392230023,0.));
#30110=CARTESIAN_POINT('Ctrl Pts',(35.1963130003352,22.4626392230023,18.));
#30111=CARTESIAN_POINT('Ctrl Pts',(35.2490119207975,22.5486956608909,0.));
#30112=CARTESIAN_POINT('Ctrl Pts',(35.2490119207975,22.5486956608909,18.));
#30113=CARTESIAN_POINT('Ctrl Pts',(35.3013079759252,22.635155167154,0.));
#30114=CARTESIAN_POINT('Ctrl Pts',(35.3013079759252,22.635155167154,18.));
#30115=CARTESIAN_POINT('Ctrl Pts',(35.3532026952313,22.7220131336912,0.));
#30116=CARTESIAN_POINT('Ctrl Pts',(35.3532026952313,22.7220131336912,18.));
#30117=CARTESIAN_POINT('Ctrl Pts',(35.4046974393492,22.8092652000706,0.));
#30118=CARTESIAN_POINT('Ctrl Pts',(35.4046974393492,22.8092652000706,18.));
#30119=CARTESIAN_POINT('Ctrl Pts',(35.4557934871468,22.8969071125089,0.));
#30120=CARTESIAN_POINT('Ctrl Pts',(35.4557934871468,22.8969071125089,18.));
#30121=CARTESIAN_POINT('Ctrl Pts',(35.5064921357308,22.9849345572033,0.));
#30122=CARTESIAN_POINT('Ctrl Pts',(35.5064921357308,22.9849345572033,18.));
#30123=CARTESIAN_POINT('Ctrl Pts',(35.5567947408311,23.0733431097058,0.));
#30124=CARTESIAN_POINT('Ctrl Pts',(35.5567947408311,23.0733431097058,18.));
#30125=CARTESIAN_POINT('Ctrl Pts',(35.6067026687722,23.1621283508111,0.));
#30126=CARTESIAN_POINT('Ctrl Pts',(35.6067026687722,23.1621283508111,18.));
#30127=CARTESIAN_POINT('Ctrl Pts',(35.6562172725207,23.2512859425032,0.));
#30128=CARTESIAN_POINT('Ctrl Pts',(35.6562172725207,23.2512859425032,18.));
#30129=CARTESIAN_POINT('Ctrl Pts',(35.7053398620512,23.3408117088761,0.));
#30130=CARTESIAN_POINT('Ctrl Pts',(35.7053398620512,23.3408117088761,18.));
#30131=CARTESIAN_POINT('Ctrl Pts',(35.7540716771372,23.4307017328227,0.));
#30132=CARTESIAN_POINT('Ctrl Pts',(35.7540716771372,23.4307017328227,18.));
#30133=CARTESIAN_POINT('Ctrl Pts',(35.8024138716897,23.5209523746427,0.));
#30134=CARTESIAN_POINT('Ctrl Pts',(35.8024138716897,23.5209523746427,18.));
#30135=CARTESIAN_POINT('Ctrl Pts',(35.8503675222884,23.611560139948,0.));
#30136=CARTESIAN_POINT('Ctrl Pts',(35.8503675222884,23.611560139948,18.));
#30137=CARTESIAN_POINT('Ctrl Pts',(35.8979336336837,23.7025215735353,0.));
#30138=CARTESIAN_POINT('Ctrl Pts',(35.8979336336837,23.7025215735353,18.));
#30139=CARTESIAN_POINT('Ctrl Pts',(35.9451131482488,23.7938331508737,0.));
#30140=CARTESIAN_POINT('Ctrl Pts',(35.9451131482488,23.7938331508737,18.));
#30141=CARTESIAN_POINT('Ctrl Pts',(35.991906956547,23.8854911428946,0.));
#30142=CARTESIAN_POINT('Ctrl Pts',(35.991906956547,23.8854911428946,18.));
#30143=CARTESIAN_POINT('Ctrl Pts',(36.0383159101253,23.9774915680089,0.));
#30144=CARTESIAN_POINT('Ctrl Pts',(36.0383159101253,23.9774915680089,18.));
#30145=CARTESIAN_POINT('Ctrl Pts',(36.0843408347974,24.0698304230588,0.));
#30146=CARTESIAN_POINT('Ctrl Pts',(36.0843408347974,24.0698304230588,18.));
#30147=CARTESIAN_POINT('Ctrl Pts',(36.1299825471271,24.1625038657964,0.));
#30148=CARTESIAN_POINT('Ctrl Pts',(36.1299825471271,24.1625038657964,18.));
#30149=CARTESIAN_POINT('Ctrl Pts',(36.1752418704833,24.2555084095332,0.));
#30150=CARTESIAN_POINT('Ctrl Pts',(36.1752418704833,24.2555084095332,18.));
#30151=CARTESIAN_POINT('Ctrl Pts',(36.2201196586696,24.3488411214068,0.));
#30152=CARTESIAN_POINT('Ctrl Pts',(36.2201196586696,24.3488411214068,18.));
#30153=CARTESIAN_POINT('Ctrl Pts',(36.2646168058395,24.4424997853604,0.));
#30154=CARTESIAN_POINT('Ctrl Pts',(36.2646168058395,24.4424997853604,18.));
#30155=CARTESIAN_POINT('Ctrl Pts',(36.308734152297,24.5364828082556,0.));
#30156=CARTESIAN_POINT('Ctrl Pts',(36.308734152297,24.5364828082556,18.));
#30157=CARTESIAN_POINT('Ctrl Pts',(36.3437247532368,24.6119278836614,0.));
#30158=CARTESIAN_POINT('Ctrl Pts',(36.3437247532368,24.6119278836614,18.));
#30159=CARTESIAN_POINT('Ctrl Pts',(36.369797330215,24.6686569322616,0.));
#30160=CARTESIAN_POINT('Ctrl Pts',(36.369797330215,24.6686569322616,18.));
#30161=CARTESIAN_POINT('Ctrl Pts',(36.3871033517098,24.7065408286023,0.));
#30162=CARTESIAN_POINT('Ctrl Pts',(36.3871033517098,24.7065408286023,18.));
#30163=CARTESIAN_POINT('Ctrl Pts',(36.3957374383337,24.725498909423,0.));
#30164=CARTESIAN_POINT('Ctrl Pts',(36.3957374383337,24.725498909423,18.));
#30165=CARTESIAN_POINT('Ctrl Pts',(32.3379313568208,19.1596907609891,0.));
#30166=CARTESIAN_POINT('Ctrl Pts',(32.3542491343753,19.1693587749508,0.));
#30167=CARTESIAN_POINT('Ctrl Pts',(32.3866012518553,19.1891139208368,0.));
#30168=CARTESIAN_POINT('Ctrl Pts',(32.4342791270009,19.2200039764927,0.));
#30169=CARTESIAN_POINT('Ctrl Pts',(32.4962340238036,19.2635813403783,0.));
#30170=CARTESIAN_POINT('Ctrl Pts',(32.5714771007861,19.3213180490743,0.));
#30171=CARTESIAN_POINT('Ctrl Pts',(32.6451434870609,19.381405831319,0.));
#30172=CARTESIAN_POINT('Ctrl Pts',(32.7178463324062,19.4429429601189,0.));
#30173=CARTESIAN_POINT('Ctrl Pts',(32.7900335943248,19.5052640847974,0.));
#30174=CARTESIAN_POINT('Ctrl Pts',(32.8618672807884,19.5681157030437,0.));
#30175=CARTESIAN_POINT('Ctrl Pts',(32.9333211533788,19.6315161742485,0.));
#30176=CARTESIAN_POINT('Ctrl Pts',(33.004256563411,19.6956473461873,0.));
#30177=CARTESIAN_POINT('Ctrl Pts',(33.0745026283418,19.7607398248651,0.));
#30178=CARTESIAN_POINT('Ctrl Pts',(33.1439436707661,19.8269479776239,0.));
#30179=CARTESIAN_POINT('Ctrl Pts',(33.2125746879471,19.8942704458546,0.));
#30180=CARTESIAN_POINT('Ctrl Pts',(33.2804560993213,19.9626141625205,0.));
#30181=CARTESIAN_POINT('Ctrl Pts',(33.3476854048385,20.0318342617212,0.));
#30182=CARTESIAN_POINT('Ctrl Pts',(33.4143643679979,20.1017803986381,0.));
#30183=CARTESIAN_POINT('Ctrl Pts',(33.480563024813,20.1723475154533,0.));
#30184=CARTESIAN_POINT('Ctrl Pts',(33.5463023319603,20.243500298383,0.));
#30185=CARTESIAN_POINT('Ctrl Pts',(33.6115742164079,20.3152448035298,0.));
#30186=CARTESIAN_POINT('Ctrl Pts',(33.6763537716992,20.3876111773341,0.));
#30187=CARTESIAN_POINT('Ctrl Pts',(33.7406135254082,20.4606334536183,0.));
#30188=CARTESIAN_POINT('Ctrl Pts',(33.8043393734971,20.5343269914034,0.));
#30189=CARTESIAN_POINT('Ctrl Pts',(33.8675365150454,20.6086800574386,0.));
#30190=CARTESIAN_POINT('Ctrl Pts',(33.9302209962425,20.683665762903,0.));
#30191=CARTESIAN_POINT('Ctrl Pts',(33.9924146647395,20.7592491770603,0.));
#30192=CARTESIAN_POINT('Ctrl Pts',(34.0541392299678,20.8353957068415,0.));
#30193=CARTESIAN_POINT('Ctrl Pts',(34.1154095510973,20.9120805673809,0.));
#30194=CARTESIAN_POINT('Ctrl Pts',(34.176231731809,20.9892914622612,0.));
#30195=CARTESIAN_POINT('Ctrl Pts',(34.2366067284279,21.0670234747355,0.));
#30196=CARTESIAN_POINT('Ctrl Pts',(34.2965325673384,21.1452759244399,0.));
#30197=CARTESIAN_POINT('Ctrl Pts',(34.3560069185815,21.2240487218079,0.));
#30198=CARTESIAN_POINT('Ctrl Pts',(34.4150300340623,21.3033382073239,0.));
#30199=CARTESIAN_POINT('Ctrl Pts',(34.4736054662052,21.3831361300104,0.));
#30200=CARTESIAN_POINT('Ctrl Pts',(34.5317385658329,21.4634317666005,0.));
#30201=CARTESIAN_POINT('Ctrl Pts',(34.5894355639082,21.5442132160757,0.));
#30202=CARTESIAN_POINT('Ctrl Pts',(34.6467025072367,21.6254689009796,0.));
#30203=CARTESIAN_POINT('Ctrl Pts',(34.7035440429025,21.7071892844497,0.));
#30204=CARTESIAN_POINT('Ctrl Pts',(34.7599631530844,21.7893672401137,0.));
#30205=CARTESIAN_POINT('Ctrl Pts',(34.8159618014436,21.8719971302817,0.));
#30206=CARTESIAN_POINT('Ctrl Pts',(34.8715413418101,21.9550742217675,0.));
#30207=CARTESIAN_POINT('Ctrl Pts',(34.9267029879922,22.0385940162683,0.));
#30208=CARTESIAN_POINT('Ctrl Pts',(34.9814483545602,22.1225514798584,0.));
#30209=CARTESIAN_POINT('Ctrl Pts',(35.0357795922459,22.2069408519232,0.));
#30210=CARTESIAN_POINT('Ctrl Pts',(35.0896991159359,22.2917560356803,0.));
#30211=CARTESIAN_POINT('Ctrl Pts',(35.1432094422642,22.3769908340843,0.));
#30212=CARTESIAN_POINT('Ctrl Pts',(35.1963130003352,22.4626392230023,0.));
#30213=CARTESIAN_POINT('Ctrl Pts',(35.2490119207975,22.5486956608909,0.));
#30214=CARTESIAN_POINT('Ctrl Pts',(35.3013079759252,22.635155167154,0.));
#30215=CARTESIAN_POINT('Ctrl Pts',(35.3532026952313,22.7220131336912,0.));
#30216=CARTESIAN_POINT('Ctrl Pts',(35.4046974393492,22.8092652000706,0.));
#30217=CARTESIAN_POINT('Ctrl Pts',(35.4557934871468,22.8969071125089,0.));
#30218=CARTESIAN_POINT('Ctrl Pts',(35.5064921357308,22.9849345572033,0.));
#30219=CARTESIAN_POINT('Ctrl Pts',(35.5567947408311,23.0733431097058,0.));
#30220=CARTESIAN_POINT('Ctrl Pts',(35.6067026687722,23.1621283508111,0.));
#30221=CARTESIAN_POINT('Ctrl Pts',(35.6562172725207,23.2512859425032,0.));
#30222=CARTESIAN_POINT('Ctrl Pts',(35.7053398620512,23.3408117088761,0.));
#30223=CARTESIAN_POINT('Ctrl Pts',(35.7540716771372,23.4307017328227,0.));
#30224=CARTESIAN_POINT('Ctrl Pts',(35.8024138716897,23.5209523746427,0.));
#30225=CARTESIAN_POINT('Ctrl Pts',(35.8503675222884,23.611560139948,0.));
#30226=CARTESIAN_POINT('Ctrl Pts',(35.8979336336837,23.7025215735353,0.));
#30227=CARTESIAN_POINT('Ctrl Pts',(35.9451131482488,23.7938331508737,0.));
#30228=CARTESIAN_POINT('Ctrl Pts',(35.991906956547,23.8854911428946,0.));
#30229=CARTESIAN_POINT('Ctrl Pts',(36.0383159101253,23.9774915680089,0.));
#30230=CARTESIAN_POINT('Ctrl Pts',(36.0843408347974,24.0698304230588,0.));
#30231=CARTESIAN_POINT('Ctrl Pts',(36.1299825471271,24.1625038657964,0.));
#30232=CARTESIAN_POINT('Ctrl Pts',(36.1752418704833,24.2555084095332,0.));
#30233=CARTESIAN_POINT('Ctrl Pts',(36.2201196586696,24.3488411214068,0.));
#30234=CARTESIAN_POINT('Ctrl Pts',(36.2735162352735,24.4612315181511,0.));
#30235=CARTESIAN_POINT('Ctrl Pts',(36.3175386315529,24.5552956307817,0.));
#30236=CARTESIAN_POINT('Ctrl Pts',(36.3524534604648,24.630805301288,0.));
#30237=CARTESIAN_POINT('Ctrl Pts',(36.3784692650901,24.6875827477484,0.));
#30238=CARTESIAN_POINT('Ctrl Pts',(36.3957374383337,24.725498909423,0.));
#30239=CARTESIAN_POINT('Ctrl Pts',(32.3379313568208,19.1596907609891,15.));
#30240=CARTESIAN_POINT('Ctrl Pts',(32.3542491343753,19.1693587749508,15.));
#30241=CARTESIAN_POINT('Ctrl Pts',(32.3866012518553,19.1891139208368,15.));
#30242=CARTESIAN_POINT('Ctrl Pts',(32.4342791270009,19.2200039764927,15.));
#30243=CARTESIAN_POINT('Ctrl Pts',(32.4962340238036,19.2635813403783,15.));
#30244=CARTESIAN_POINT('Ctrl Pts',(32.5714771007861,19.3213180490743,15.));
#30245=CARTESIAN_POINT('Ctrl Pts',(32.6451434870609,19.381405831319,15.));
#30246=CARTESIAN_POINT('Ctrl Pts',(32.7178463324062,19.4429429601189,15.));
#30247=CARTESIAN_POINT('Ctrl Pts',(32.7900335943248,19.5052640847974,15.));
#30248=CARTESIAN_POINT('Ctrl Pts',(32.8618672807884,19.5681157030437,15.));
#30249=CARTESIAN_POINT('Ctrl Pts',(32.9333211533788,19.6315161742485,15.));
#30250=CARTESIAN_POINT('Ctrl Pts',(33.004256563411,19.6956473461873,15.));
#30251=CARTESIAN_POINT('Ctrl Pts',(33.0745026283418,19.7607398248651,15.));
#30252=CARTESIAN_POINT('Ctrl Pts',(33.1439436707661,19.8269479776239,15.));
#30253=CARTESIAN_POINT('Ctrl Pts',(33.2125746879471,19.8942704458546,15.));
#30254=CARTESIAN_POINT('Ctrl Pts',(33.2804560993213,19.9626141625205,15.));
#30255=CARTESIAN_POINT('Ctrl Pts',(33.3476854048385,20.0318342617212,15.));
#30256=CARTESIAN_POINT('Ctrl Pts',(33.4143643679979,20.1017803986381,15.));
#30257=CARTESIAN_POINT('Ctrl Pts',(33.480563024813,20.1723475154533,15.));
#30258=CARTESIAN_POINT('Ctrl Pts',(33.5463023319603,20.243500298383,15.));
#30259=CARTESIAN_POINT('Ctrl Pts',(33.6115742164079,20.3152448035298,15.));
#30260=CARTESIAN_POINT('Ctrl Pts',(33.6763537716992,20.3876111773341,15.));
#30261=CARTESIAN_POINT('Ctrl Pts',(33.7406135254082,20.4606334536183,15.));
#30262=CARTESIAN_POINT('Ctrl Pts',(33.8043393734971,20.5343269914034,15.));
#30263=CARTESIAN_POINT('Ctrl Pts',(33.8675365150454,20.6086800574386,15.));
#30264=CARTESIAN_POINT('Ctrl Pts',(33.9302209962425,20.683665762903,15.));
#30265=CARTESIAN_POINT('Ctrl Pts',(33.9924146647395,20.7592491770603,15.));
#30266=CARTESIAN_POINT('Ctrl Pts',(34.0541392299678,20.8353957068415,15.));
#30267=CARTESIAN_POINT('Ctrl Pts',(34.1154095510973,20.9120805673809,15.));
#30268=CARTESIAN_POINT('Ctrl Pts',(34.176231731809,20.9892914622612,15.));
#30269=CARTESIAN_POINT('Ctrl Pts',(34.2366067284279,21.0670234747355,15.));
#30270=CARTESIAN_POINT('Ctrl Pts',(34.2965325673384,21.1452759244399,15.));
#30271=CARTESIAN_POINT('Ctrl Pts',(34.3560069185815,21.2240487218079,15.));
#30272=CARTESIAN_POINT('Ctrl Pts',(34.4150300340623,21.3033382073239,15.));
#30273=CARTESIAN_POINT('Ctrl Pts',(34.4736054662052,21.3831361300104,15.));
#30274=CARTESIAN_POINT('Ctrl Pts',(34.5317385658329,21.4634317666005,15.));
#30275=CARTESIAN_POINT('Ctrl Pts',(34.5894355639082,21.5442132160757,15.));
#30276=CARTESIAN_POINT('Ctrl Pts',(34.6467025072367,21.6254689009796,15.));
#30277=CARTESIAN_POINT('Ctrl Pts',(34.7035440429025,21.7071892844497,15.));
#30278=CARTESIAN_POINT('Ctrl Pts',(34.7599631530844,21.7893672401137,15.));
#30279=CARTESIAN_POINT('Ctrl Pts',(34.8159618014436,21.8719971302817,15.));
#30280=CARTESIAN_POINT('Ctrl Pts',(34.8715413418101,21.9550742217675,15.));
#30281=CARTESIAN_POINT('Ctrl Pts',(34.9267029879922,22.0385940162683,15.));
#30282=CARTESIAN_POINT('Ctrl Pts',(34.9814483545602,22.1225514798584,15.));
#30283=CARTESIAN_POINT('Ctrl Pts',(35.0357795922459,22.2069408519232,15.));
#30284=CARTESIAN_POINT('Ctrl Pts',(35.0896991159359,22.2917560356803,15.));
#30285=CARTESIAN_POINT('Ctrl Pts',(35.1432094422642,22.3769908340843,15.));
#30286=CARTESIAN_POINT('Ctrl Pts',(35.1963130003352,22.4626392230023,15.));
#30287=CARTESIAN_POINT('Ctrl Pts',(35.2490119207975,22.5486956608909,15.));
#30288=CARTESIAN_POINT('Ctrl Pts',(35.3013079759252,22.635155167154,15.));
#30289=CARTESIAN_POINT('Ctrl Pts',(35.3532026952313,22.7220131336912,15.));
#30290=CARTESIAN_POINT('Ctrl Pts',(35.4046974393492,22.8092652000706,15.));
#30291=CARTESIAN_POINT('Ctrl Pts',(35.4557934871468,22.8969071125089,15.));
#30292=CARTESIAN_POINT('Ctrl Pts',(35.5064921357308,22.9849345572033,15.));
#30293=CARTESIAN_POINT('Ctrl Pts',(35.5567947408311,23.0733431097058,15.));
#30294=CARTESIAN_POINT('Ctrl Pts',(35.6067026687722,23.1621283508111,15.));
#30295=CARTESIAN_POINT('Ctrl Pts',(35.6562172725207,23.2512859425032,15.));
#30296=CARTESIAN_POINT('Ctrl Pts',(35.7053398620512,23.3408117088761,15.));
#30297=CARTESIAN_POINT('Ctrl Pts',(35.7540716771372,23.4307017328227,15.));
#30298=CARTESIAN_POINT('Ctrl Pts',(35.8024138716897,23.5209523746427,15.));
#30299=CARTESIAN_POINT('Ctrl Pts',(35.8503675222884,23.611560139948,15.));
#30300=CARTESIAN_POINT('Ctrl Pts',(35.8979336336837,23.7025215735353,15.));
#30301=CARTESIAN_POINT('Ctrl Pts',(35.9451131482488,23.7938331508737,15.));
#30302=CARTESIAN_POINT('Ctrl Pts',(35.991906956547,23.8854911428946,15.));
#30303=CARTESIAN_POINT('Ctrl Pts',(36.0383159101253,23.9774915680089,15.));
#30304=CARTESIAN_POINT('Ctrl Pts',(36.0843408347974,24.0698304230588,15.));
#30305=CARTESIAN_POINT('Ctrl Pts',(36.1299825471271,24.1625038657964,15.));
#30306=CARTESIAN_POINT('Ctrl Pts',(36.1752418704833,24.2555084095332,15.));
#30307=CARTESIAN_POINT('Ctrl Pts',(36.2201196586696,24.3488411214068,15.));
#30308=CARTESIAN_POINT('Ctrl Pts',(36.2735162352735,24.4612315181511,15.));
#30309=CARTESIAN_POINT('Ctrl Pts',(36.3175386315529,24.5552956307817,15.));
#30310=CARTESIAN_POINT('Ctrl Pts',(36.3524534604648,24.630805301288,15.));
#30311=CARTESIAN_POINT('Ctrl Pts',(36.3784692650901,24.6875827477484,15.));
#30312=CARTESIAN_POINT('Ctrl Pts',(36.3957374383337,24.725498909423,15.));
#30313=CARTESIAN_POINT('Ctrl Pts',(41.396226524684,14.911486495888,0.));
#30314=CARTESIAN_POINT('Ctrl Pts',(41.396226524684,14.911486495888,18.));
#30315=CARTESIAN_POINT('Ctrl Pts',(41.3758141263348,14.9156446533966,0.));
#30316=CARTESIAN_POINT('Ctrl Pts',(41.3758141263348,14.9156446533966,18.));
#30317=CARTESIAN_POINT('Ctrl Pts',(41.3349931861715,14.9239113834707,0.));
#30318=CARTESIAN_POINT('Ctrl Pts',(41.3349931861715,14.9239113834707,18.));
#30319=CARTESIAN_POINT('Ctrl Pts',(41.2737733455422,14.936162723752,0.));
#30320=CARTESIAN_POINT('Ctrl Pts',(41.2737733455422,14.936162723752,18.));
#30321=CARTESIAN_POINT('Ctrl Pts',(41.1921700381957,14.9522002356298,0.));
#30322=CARTESIAN_POINT('Ctrl Pts',(41.1921700381957,14.9522002356298,18.));
#30323=CARTESIAN_POINT('Ctrl Pts',(41.0902046498729,14.9717503874227,0.));
#30324=CARTESIAN_POINT('Ctrl Pts',(41.0902046498729,14.9717503874227,18.));
#30325=CARTESIAN_POINT('Ctrl Pts',(40.9882784321884,14.9908026205824,0.));
#30326=CARTESIAN_POINT('Ctrl Pts',(40.9882784321884,14.9908026205824,18.));
#30327=CARTESIAN_POINT('Ctrl Pts',(40.8863921801,15.0093553188655,0.));
#30328=CARTESIAN_POINT('Ctrl Pts',(40.8863921801,15.0093553188655,18.));
#30329=CARTESIAN_POINT('Ctrl Pts',(40.7845471608654,15.0274064563211,0.));
#30330=CARTESIAN_POINT('Ctrl Pts',(40.7845471608654,15.0274064563211,18.));
#30331=CARTESIAN_POINT('Ctrl Pts',(40.6827452453667,15.0449536183143,0.));
#30332=CARTESIAN_POINT('Ctrl Pts',(40.6827452453667,15.0449536183143,18.));
#30333=CARTESIAN_POINT('Ctrl Pts',(40.58098877043,15.0619940893017,0.));
#30334=CARTESIAN_POINT('Ctrl Pts',(40.58098877043,15.0619940893017,18.));
#30335=CARTESIAN_POINT('Ctrl Pts',(40.4792803645352,15.0785249502524,0.));
#30336=CARTESIAN_POINT('Ctrl Pts',(40.4792803645352,15.0785249502524,18.));
#30337=CARTESIAN_POINT('Ctrl Pts',(40.3776227809037,15.0945431800723,0.));
#30338=CARTESIAN_POINT('Ctrl Pts',(40.3776227809037,15.0945431800723,18.));
#30339=CARTESIAN_POINT('Ctrl Pts',(40.2760187401821,15.1100457495259,0.));
#30340=CARTESIAN_POINT('Ctrl Pts',(40.2760187401821,15.1100457495259,18.));
#30341=CARTESIAN_POINT('Ctrl Pts',(40.1744707357902,15.1250297462408,0.));
#30342=CARTESIAN_POINT('Ctrl Pts',(40.1744707357902,15.1250297462408,18.));
#30343=CARTESIAN_POINT('Ctrl Pts',(40.0729810652204,15.1394923361537,0.));
#30344=CARTESIAN_POINT('Ctrl Pts',(40.0729810652204,15.1394923361537,18.));
#30345=CARTESIAN_POINT('Ctrl Pts',(39.9715519332134,15.1534306754871,0.));
#30346=CARTESIAN_POINT('Ctrl Pts',(39.9715519332134,15.1534306754871,18.));
#30347=CARTESIAN_POINT('Ctrl Pts',(39.8701855339908,15.1668418393198,0.));
#30348=CARTESIAN_POINT('Ctrl Pts',(39.8701855339908,15.1668418393198,18.));
#30349=CARTESIAN_POINT('Ctrl Pts',(39.7688841338802,15.1797227547561,0.));
#30350=CARTESIAN_POINT('Ctrl Pts',(39.7688841338802,15.1797227547561,18.));
#30351=CARTESIAN_POINT('Ctrl Pts',(39.6676501731673,15.1920701163803,0.));
#30352=CARTESIAN_POINT('Ctrl Pts',(39.6676501731673,15.1920701163803,18.));
#30353=CARTESIAN_POINT('Ctrl Pts',(39.5664862602472,15.2038804098649,0.));
#30354=CARTESIAN_POINT('Ctrl Pts',(39.5664862602472,15.2038804098649,18.));
#30355=CARTESIAN_POINT('Ctrl Pts',(39.4653951093947,15.2151499908149,0.));
#30356=CARTESIAN_POINT('Ctrl Pts',(39.4653951093947,15.2151499908149,18.));
#30357=CARTESIAN_POINT('Ctrl Pts',(39.3643794927167,15.225875156307,0.));
#30358=CARTESIAN_POINT('Ctrl Pts',(39.3643794927167,15.225875156307,18.));
#30359=CARTESIAN_POINT('Ctrl Pts',(39.2634421927888,15.2360522089072,0.));
#30360=CARTESIAN_POINT('Ctrl Pts',(39.2634421927888,15.2360522089072,18.));
#30361=CARTESIAN_POINT('Ctrl Pts',(39.1625859371304,15.2456775636447,0.));
#30362=CARTESIAN_POINT('Ctrl Pts',(39.1625859371304,15.2456775636447,18.));
#30363=CARTESIAN_POINT('Ctrl Pts',(39.061813415425,15.2547476855825,0.));
#30364=CARTESIAN_POINT('Ctrl Pts',(39.061813415425,15.2547476855825,18.));
#30365=CARTESIAN_POINT('Ctrl Pts',(38.9611273555758,15.2632589109473,0.));
#30366=CARTESIAN_POINT('Ctrl Pts',(38.9611273555758,15.2632589109473,18.));
#30367=CARTESIAN_POINT('Ctrl Pts',(38.860530586589,15.2712072937639,0.));
#30368=CARTESIAN_POINT('Ctrl Pts',(38.860530586589,15.2712072937639,18.));
#30369=CARTESIAN_POINT('Ctrl Pts',(38.7600260961351,15.2785884727112,0.));
#30370=CARTESIAN_POINT('Ctrl Pts',(38.7600260961351,15.2785884727112,18.));
#30371=CARTESIAN_POINT('Ctrl Pts',(38.659617115053,15.2853974668211,0.));
#30372=CARTESIAN_POINT('Ctrl Pts',(38.659617115053,15.2853974668211,18.));
#30373=CARTESIAN_POINT('Ctrl Pts',(38.5593070891769,15.2916287700102,0.));
#30374=CARTESIAN_POINT('Ctrl Pts',(38.5593070891769,15.2916287700102,18.));
#30375=CARTESIAN_POINT('Ctrl Pts',(38.4590995527814,15.2972767037469,0.));
#30376=CARTESIAN_POINT('Ctrl Pts',(38.4590995527814,15.2972767037469,18.));
#30377=CARTESIAN_POINT('Ctrl Pts',(38.3589980188324,15.3023357307483,0.));
#30378=CARTESIAN_POINT('Ctrl Pts',(38.3589980188324,15.3023357307483,18.));
#30379=CARTESIAN_POINT('Ctrl Pts',(38.2590058835965,15.3068007250314,0.));
#30380=CARTESIAN_POINT('Ctrl Pts',(38.2590058835965,15.3068007250314,18.));
#30381=CARTESIAN_POINT('Ctrl Pts',(38.1591262705847,15.310667421514,0.));
#30382=CARTESIAN_POINT('Ctrl Pts',(38.1591262705847,15.310667421514,18.));
#30383=CARTESIAN_POINT('Ctrl Pts',(38.0593621055415,15.3139321941687,0.));
#30384=CARTESIAN_POINT('Ctrl Pts',(38.0593621055415,15.3139321941687,18.));
#30385=CARTESIAN_POINT('Ctrl Pts',(37.959716421934,15.3165911656268,0.));
#30386=CARTESIAN_POINT('Ctrl Pts',(37.959716421934,15.3165911656268,18.));
#30387=CARTESIAN_POINT('Ctrl Pts',(37.8601926265378,15.3186394335023,0.));
#30388=CARTESIAN_POINT('Ctrl Pts',(37.8601926265378,15.3186394335023,18.));
#30389=CARTESIAN_POINT('Ctrl Pts',(37.7607947318286,15.320070396385,0.));
#30390=CARTESIAN_POINT('Ctrl Pts',(37.7607947318286,15.320070396385,18.));
#30391=CARTESIAN_POINT('Ctrl Pts',(37.6615277218027,15.320874689078,0.));
#30392=CARTESIAN_POINT('Ctrl Pts',(37.6615277218027,15.320874689078,18.));
#30393=CARTESIAN_POINT('Ctrl Pts',(37.562397408596,15.3210406145546,0.));
#30394=CARTESIAN_POINT('Ctrl Pts',(37.562397408596,15.3210406145546,18.));
#30395=CARTESIAN_POINT('Ctrl Pts',(37.4634097578665,15.3205561366169,0.));
#30396=CARTESIAN_POINT('Ctrl Pts',(37.4634097578665,15.3205561366169,18.));
#30397=CARTESIAN_POINT('Ctrl Pts',(37.3645702997848,15.3194106233801,0.));
#30398=CARTESIAN_POINT('Ctrl Pts',(37.3645702997848,15.3194106233801,18.));
#30399=CARTESIAN_POINT('Ctrl Pts',(37.2658836214694,15.3175963510698,0.));
#30400=CARTESIAN_POINT('Ctrl Pts',(37.2658836214694,15.3175963510698,18.));
#30401=CARTESIAN_POINT('Ctrl Pts',(37.1673525354642,15.3151109648809,0.));
#30402=CARTESIAN_POINT('Ctrl Pts',(37.1673525354642,15.3151109648809,18.));
#30403=CARTESIAN_POINT('Ctrl Pts',(37.0689784837457,15.3119562971444,0.));
#30404=CARTESIAN_POINT('Ctrl Pts',(37.0689784837457,15.3119562971444,18.));
#30405=CARTESIAN_POINT('Ctrl Pts',(36.970763176802,15.3081335446406,0.));
#30406=CARTESIAN_POINT('Ctrl Pts',(36.970763176802,15.3081335446406,18.));
#30407=CARTESIAN_POINT('Ctrl Pts',(36.8727100302512,15.3036390436952,0.));
#30408=CARTESIAN_POINT('Ctrl Pts',(36.8727100302512,15.3036390436952,18.));
#30409=CARTESIAN_POINT('Ctrl Pts',(36.7748254044502,15.2984606286737,0.));
#30410=CARTESIAN_POINT('Ctrl Pts',(36.7748254044502,15.2984606286737,18.));
#30411=CARTESIAN_POINT('Ctrl Pts',(36.6771206167755,15.2925717100767,0.));
#30412=CARTESIAN_POINT('Ctrl Pts',(36.6771206167755,15.2925717100767,18.));
#30413=CARTESIAN_POINT('Ctrl Pts',(36.5796108931244,15.2859343913094,0.));
#30414=CARTESIAN_POINT('Ctrl Pts',(36.5796108931244,15.2859343913094,18.));
#30415=CARTESIAN_POINT('Ctrl Pts',(36.4823116513289,15.2785104654792,0.));
#30416=CARTESIAN_POINT('Ctrl Pts',(36.4823116513289,15.2785104654792,18.));
#30417=CARTESIAN_POINT('Ctrl Pts',(36.3852352131887,15.2702711460937,0.));
#30418=CARTESIAN_POINT('Ctrl Pts',(36.3852352131887,15.2702711460937,18.));
#30419=CARTESIAN_POINT('Ctrl Pts',(36.2883880151607,15.2612053303773,0.));
#30420=CARTESIAN_POINT('Ctrl Pts',(36.2883880151607,15.2612053303773,18.));
#30421=CARTESIAN_POINT('Ctrl Pts',(36.1917659216814,15.2513334565427,0.));
#30422=CARTESIAN_POINT('Ctrl Pts',(36.1917659216814,15.2513334565427,18.));
#30423=CARTESIAN_POINT('Ctrl Pts',(36.095357546697,15.240697754828,0.));
#30424=CARTESIAN_POINT('Ctrl Pts',(36.095357546697,15.240697754828,18.));
#30425=CARTESIAN_POINT('Ctrl Pts',(35.9991531408727,15.2293360946131,0.));
#30426=CARTESIAN_POINT('Ctrl Pts',(35.9991531408727,15.2293360946131,18.));
#30427=CARTESIAN_POINT('Ctrl Pts',(35.9031525499277,15.2172585668056,0.));
#30428=CARTESIAN_POINT('Ctrl Pts',(35.9031525499277,15.2172585668056,18.));
#30429=CARTESIAN_POINT('Ctrl Pts',(35.8073720252878,15.2044274601769,0.));
#30430=CARTESIAN_POINT('Ctrl Pts',(35.8073720252878,15.2044274601769,18.));
#30431=CARTESIAN_POINT('Ctrl Pts',(35.7118553943773,15.1907243629659,0.));
#30432=CARTESIAN_POINT('Ctrl Pts',(35.7118553943773,15.1907243629659,18.));
#30433=CARTESIAN_POINT('Ctrl Pts',(35.6166644736253,15.1759785763051,0.));
#30434=CARTESIAN_POINT('Ctrl Pts',(35.6166644736253,15.1759785763051,18.));
#30435=CARTESIAN_POINT('Ctrl Pts',(35.5218591529745,15.1600260710384,0.));
#30436=CARTESIAN_POINT('Ctrl Pts',(35.5218591529745,15.1600260710384,18.));
#30437=CARTESIAN_POINT('Ctrl Pts',(35.4274792115856,15.1427632633831,0.));
#30438=CARTESIAN_POINT('Ctrl Pts',(35.4274792115856,15.1427632633831,18.));
#30439=CARTESIAN_POINT('Ctrl Pts',(35.3335286891314,15.1241934020681,0.));
#30440=CARTESIAN_POINT('Ctrl Pts',(35.3335286891314,15.1241934020681,18.));
#30441=CARTESIAN_POINT('Ctrl Pts',(35.2399506932815,15.104500806927,0.));
#30442=CARTESIAN_POINT('Ctrl Pts',(35.2399506932815,15.104500806927,18.));
#30443=CARTESIAN_POINT('Ctrl Pts',(35.1466591020976,15.08395927165,0.));
#30444=CARTESIAN_POINT('Ctrl Pts',(35.1466591020976,15.08395927165,18.));
#30445=CARTESIAN_POINT('Ctrl Pts',(35.0535882932913,15.0627878528202,0.));
#30446=CARTESIAN_POINT('Ctrl Pts',(35.0535882932913,15.0627878528202,18.));
#30447=CARTESIAN_POINT('Ctrl Pts',(34.9607388363587,15.041018569143,0.));
#30448=CARTESIAN_POINT('Ctrl Pts',(34.9607388363587,15.041018569143,18.));
#30449=CARTESIAN_POINT('Ctrl Pts',(34.8682205930809,15.0183713484962,0.));
#30450=CARTESIAN_POINT('Ctrl Pts',(34.8682205930809,15.0183713484962,18.));
#30451=CARTESIAN_POINT('Ctrl Pts',(34.7763085406486,14.9940927023322,0.));
#30452=CARTESIAN_POINT('Ctrl Pts',(34.7763085406486,14.9940927023322,18.));
#30453=CARTESIAN_POINT('Ctrl Pts',(34.6853717911268,14.9671565602316,0.));
#30454=CARTESIAN_POINT('Ctrl Pts',(34.6853717911268,14.9671565602316,18.));
#30455=CARTESIAN_POINT('Ctrl Pts',(34.6137007885254,14.9426481276593,0.));
#30456=CARTESIAN_POINT('Ctrl Pts',(34.6137007885254,14.9426481276593,18.));
#30457=CARTESIAN_POINT('Ctrl Pts',(34.5606858566713,14.9222326355678,0.));
#30458=CARTESIAN_POINT('Ctrl Pts',(34.5606858566713,14.9222326355678,18.));
#30459=CARTESIAN_POINT('Ctrl Pts',(34.525687510388,14.9076710061311,0.));
#30460=CARTESIAN_POINT('Ctrl Pts',(34.525687510388,14.9076710061311,18.));
#30461=CARTESIAN_POINT('Ctrl Pts',(34.5082745737944,14.9001523628048,0.));
#30462=CARTESIAN_POINT('Ctrl Pts',(34.5082745737944,14.9001523628048,18.));
#30463=CARTESIAN_POINT('',(41.3962265246839,14.9114864958881,0.));
#30464=CARTESIAN_POINT('Ctrl Pts',(34.5082745737944,14.9001523628048,0.));
#30465=CARTESIAN_POINT('Ctrl Pts',(34.525687510388,14.9076710061311,0.));
#30466=CARTESIAN_POINT('Ctrl Pts',(34.5606858566713,14.9222326355678,0.));
#30467=CARTESIAN_POINT('Ctrl Pts',(34.6137007885254,14.9426481276593,0.));
#30468=CARTESIAN_POINT('Ctrl Pts',(34.6853717911268,14.9671565602316,0.));
#30469=CARTESIAN_POINT('Ctrl Pts',(34.7763085406486,14.9940927023322,0.));
#30470=CARTESIAN_POINT('Ctrl Pts',(34.8682205930809,15.0183713484962,0.));
#30471=CARTESIAN_POINT('Ctrl Pts',(34.9607388363587,15.041018569143,0.));
#30472=CARTESIAN_POINT('Ctrl Pts',(35.0535882932913,15.0627878528202,0.));
#30473=CARTESIAN_POINT('Ctrl Pts',(35.1466591020976,15.08395927165,0.));
#30474=CARTESIAN_POINT('Ctrl Pts',(35.2399506932815,15.104500806927,0.));
#30475=CARTESIAN_POINT('Ctrl Pts',(35.3335286891314,15.1241934020681,0.));
#30476=CARTESIAN_POINT('Ctrl Pts',(35.4274792115856,15.1427632633831,0.));
#30477=CARTESIAN_POINT('Ctrl Pts',(35.5218591529745,15.1600260710384,0.));
#30478=CARTESIAN_POINT('Ctrl Pts',(35.6166644736253,15.1759785763051,0.));
#30479=CARTESIAN_POINT('Ctrl Pts',(35.7118553943773,15.1907243629659,0.));
#30480=CARTESIAN_POINT('Ctrl Pts',(35.8073720252878,15.2044274601769,0.));
#30481=CARTESIAN_POINT('Ctrl Pts',(35.9031525499277,15.2172585668056,0.));
#30482=CARTESIAN_POINT('Ctrl Pts',(35.9991531408727,15.2293360946131,0.));
#30483=CARTESIAN_POINT('Ctrl Pts',(36.095357546697,15.240697754828,0.));
#30484=CARTESIAN_POINT('Ctrl Pts',(36.1917659216814,15.2513334565427,0.));
#30485=CARTESIAN_POINT('Ctrl Pts',(36.2883880151607,15.2612053303773,0.));
#30486=CARTESIAN_POINT('Ctrl Pts',(36.3852352131887,15.2702711460937,0.));
#30487=CARTESIAN_POINT('Ctrl Pts',(36.4823116513289,15.2785104654792,0.));
#30488=CARTESIAN_POINT('Ctrl Pts',(36.5796108931244,15.2859343913094,0.));
#30489=CARTESIAN_POINT('Ctrl Pts',(36.6771206167755,15.2925717100767,0.));
#30490=CARTESIAN_POINT('Ctrl Pts',(36.7748254044502,15.2984606286737,0.));
#30491=CARTESIAN_POINT('Ctrl Pts',(36.8727100302512,15.3036390436952,0.));
#30492=CARTESIAN_POINT('Ctrl Pts',(36.970763176802,15.3081335446406,0.));
#30493=CARTESIAN_POINT('Ctrl Pts',(37.0689784837457,15.3119562971444,0.));
#30494=CARTESIAN_POINT('Ctrl Pts',(37.1673525354642,15.3151109648809,0.));
#30495=CARTESIAN_POINT('Ctrl Pts',(37.2658836214694,15.3175963510698,0.));
#30496=CARTESIAN_POINT('Ctrl Pts',(37.3645702997848,15.3194106233801,0.));
#30497=CARTESIAN_POINT('Ctrl Pts',(37.4634097578665,15.3205561366169,0.));
#30498=CARTESIAN_POINT('Ctrl Pts',(37.562397408596,15.3210406145546,0.));
#30499=CARTESIAN_POINT('Ctrl Pts',(37.6615277218027,15.320874689078,0.));
#30500=CARTESIAN_POINT('Ctrl Pts',(37.7607947318286,15.320070396385,0.));
#30501=CARTESIAN_POINT('Ctrl Pts',(37.8601926265378,15.3186394335023,0.));
#30502=CARTESIAN_POINT('Ctrl Pts',(37.959716421934,15.3165911656268,0.));
#30503=CARTESIAN_POINT('Ctrl Pts',(38.0593621055415,15.3139321941687,0.));
#30504=CARTESIAN_POINT('Ctrl Pts',(38.1591262705847,15.310667421514,0.));
#30505=CARTESIAN_POINT('Ctrl Pts',(38.2590058835965,15.3068007250314,0.));
#30506=CARTESIAN_POINT('Ctrl Pts',(38.3589980188324,15.3023357307483,0.));
#30507=CARTESIAN_POINT('Ctrl Pts',(38.4590995527814,15.2972767037469,0.));
#30508=CARTESIAN_POINT('Ctrl Pts',(38.5593070891769,15.2916287700102,0.));
#30509=CARTESIAN_POINT('Ctrl Pts',(38.659617115053,15.2853974668211,0.));
#30510=CARTESIAN_POINT('Ctrl Pts',(38.7600260961351,15.2785884727112,0.));
#30511=CARTESIAN_POINT('Ctrl Pts',(38.860530586589,15.2712072937639,0.));
#30512=CARTESIAN_POINT('Ctrl Pts',(38.9611273555758,15.2632589109473,0.));
#30513=CARTESIAN_POINT('Ctrl Pts',(39.061813415425,15.2547476855825,0.));
#30514=CARTESIAN_POINT('Ctrl Pts',(39.1625859371304,15.2456775636447,0.));
#30515=CARTESIAN_POINT('Ctrl Pts',(39.2634421927888,15.2360522089072,0.));
#30516=CARTESIAN_POINT('Ctrl Pts',(39.3643794927167,15.225875156307,0.));
#30517=CARTESIAN_POINT('Ctrl Pts',(39.4653951093947,15.2151499908149,0.));
#30518=CARTESIAN_POINT('Ctrl Pts',(39.5664862602472,15.2038804098649,0.));
#30519=CARTESIAN_POINT('Ctrl Pts',(39.6676501731673,15.1920701163803,0.));
#30520=CARTESIAN_POINT('Ctrl Pts',(39.7688841338802,15.1797227547561,0.));
#30521=CARTESIAN_POINT('Ctrl Pts',(39.8701855339908,15.1668418393198,0.));
#30522=CARTESIAN_POINT('Ctrl Pts',(39.9715519332134,15.1534306754871,0.));
#30523=CARTESIAN_POINT('Ctrl Pts',(40.0729810652204,15.1394923361537,0.));
#30524=CARTESIAN_POINT('Ctrl Pts',(40.1744707357902,15.1250297462408,0.));
#30525=CARTESIAN_POINT('Ctrl Pts',(40.2760187401821,15.1100457495259,0.));
#30526=CARTESIAN_POINT('Ctrl Pts',(40.3776227809037,15.0945431800723,0.));
#30527=CARTESIAN_POINT('Ctrl Pts',(40.4792803645352,15.0785249502524,0.));
#30528=CARTESIAN_POINT('Ctrl Pts',(40.58098877043,15.0619940893017,0.));
#30529=CARTESIAN_POINT('Ctrl Pts',(40.6827452453667,15.0449536183143,0.));
#30530=CARTESIAN_POINT('Ctrl Pts',(40.7845471608654,15.0274064563211,0.));
#30531=CARTESIAN_POINT('Ctrl Pts',(40.8863921801,15.0093553188655,0.));
#30532=CARTESIAN_POINT('Ctrl Pts',(40.9882784321884,14.9908026205824,0.));
#30533=CARTESIAN_POINT('Ctrl Pts',(41.1105898934098,14.9679399407908,0.));
#30534=CARTESIAN_POINT('Ctrl Pts',(41.2125650743922,14.9482653093396,0.));
#30535=CARTESIAN_POINT('Ctrl Pts',(41.2941761025922,14.9321285285561,0.));
#30536=CARTESIAN_POINT('Ctrl Pts',(41.3554017279611,14.919802810928,0.));
#30537=CARTESIAN_POINT('Ctrl Pts',(41.396226524684,14.911486495888,0.));
#30538=CARTESIAN_POINT('',(41.3962265246839,14.9114864958881,15.));
#30539=CARTESIAN_POINT('Ctrl Pts',(41.396226524684,14.911486495888,15.));
#30540=CARTESIAN_POINT('Ctrl Pts',(41.3758141263348,14.9156446533966,15.));
#30541=CARTESIAN_POINT('Ctrl Pts',(41.3349931861715,14.9239113834707,15.));
#30542=CARTESIAN_POINT('Ctrl Pts',(41.2737733455422,14.936162723752,15.));
#30543=CARTESIAN_POINT('Ctrl Pts',(41.1921700381957,14.9522002356298,15.));
#30544=CARTESIAN_POINT('Ctrl Pts',(41.0902046498729,14.9717503874227,15.));
#30545=CARTESIAN_POINT('Ctrl Pts',(40.9882784321884,14.9908026205824,15.));
#30546=CARTESIAN_POINT('Ctrl Pts',(40.8863921801,15.0093553188655,15.));
#30547=CARTESIAN_POINT('Ctrl Pts',(40.7845471608654,15.0274064563211,15.));
#30548=CARTESIAN_POINT('Ctrl Pts',(40.6827452453667,15.0449536183143,15.));
#30549=CARTESIAN_POINT('Ctrl Pts',(40.58098877043,15.0619940893017,15.));
#30550=CARTESIAN_POINT('Ctrl Pts',(40.4792803645352,15.0785249502524,15.));
#30551=CARTESIAN_POINT('Ctrl Pts',(40.3776227809037,15.0945431800723,15.));
#30552=CARTESIAN_POINT('Ctrl Pts',(40.2760187401821,15.1100457495259,15.));
#30553=CARTESIAN_POINT('Ctrl Pts',(40.1744707357902,15.1250297462408,15.));
#30554=CARTESIAN_POINT('Ctrl Pts',(40.0729810652204,15.1394923361537,15.));
#30555=CARTESIAN_POINT('Ctrl Pts',(39.9715519332134,15.1534306754871,15.));
#30556=CARTESIAN_POINT('Ctrl Pts',(39.8701855339908,15.1668418393198,15.));
#30557=CARTESIAN_POINT('Ctrl Pts',(39.7688841338802,15.1797227547561,15.));
#30558=CARTESIAN_POINT('Ctrl Pts',(39.6676501731673,15.1920701163803,15.));
#30559=CARTESIAN_POINT('Ctrl Pts',(39.5664862602472,15.2038804098649,15.));
#30560=CARTESIAN_POINT('Ctrl Pts',(39.4653951093947,15.2151499908149,15.));
#30561=CARTESIAN_POINT('Ctrl Pts',(39.3643794927167,15.225875156307,15.));
#30562=CARTESIAN_POINT('Ctrl Pts',(39.2634421927888,15.2360522089072,15.));
#30563=CARTESIAN_POINT('Ctrl Pts',(39.1625859371304,15.2456775636447,15.));
#30564=CARTESIAN_POINT('Ctrl Pts',(39.061813415425,15.2547476855825,15.));
#30565=CARTESIAN_POINT('Ctrl Pts',(38.9611273555758,15.2632589109473,15.));
#30566=CARTESIAN_POINT('Ctrl Pts',(38.860530586589,15.2712072937639,15.));
#30567=CARTESIAN_POINT('Ctrl Pts',(38.7600260961351,15.2785884727112,15.));
#30568=CARTESIAN_POINT('Ctrl Pts',(38.659617115053,15.2853974668211,15.));
#30569=CARTESIAN_POINT('Ctrl Pts',(38.5593070891769,15.2916287700102,15.));
#30570=CARTESIAN_POINT('Ctrl Pts',(38.4590995527814,15.2972767037469,15.));
#30571=CARTESIAN_POINT('Ctrl Pts',(38.3589980188324,15.3023357307483,15.));
#30572=CARTESIAN_POINT('Ctrl Pts',(38.2590058835965,15.3068007250314,15.));
#30573=CARTESIAN_POINT('Ctrl Pts',(38.1591262705847,15.310667421514,15.));
#30574=CARTESIAN_POINT('Ctrl Pts',(38.0593621055415,15.3139321941687,15.));
#30575=CARTESIAN_POINT('Ctrl Pts',(37.959716421934,15.3165911656268,15.));
#30576=CARTESIAN_POINT('Ctrl Pts',(37.8601926265378,15.3186394335023,15.));
#30577=CARTESIAN_POINT('Ctrl Pts',(37.7607947318286,15.320070396385,15.));
#30578=CARTESIAN_POINT('Ctrl Pts',(37.6615277218027,15.320874689078,15.));
#30579=CARTESIAN_POINT('Ctrl Pts',(37.562397408596,15.3210406145546,15.));
#30580=CARTESIAN_POINT('Ctrl Pts',(37.4634097578665,15.3205561366169,15.));
#30581=CARTESIAN_POINT('Ctrl Pts',(37.3645702997848,15.3194106233801,15.));
#30582=CARTESIAN_POINT('Ctrl Pts',(37.2658836214694,15.3175963510698,15.));
#30583=CARTESIAN_POINT('Ctrl Pts',(37.1673525354642,15.3151109648809,15.));
#30584=CARTESIAN_POINT('Ctrl Pts',(37.0689784837457,15.3119562971444,15.));
#30585=CARTESIAN_POINT('Ctrl Pts',(36.970763176802,15.3081335446406,15.));
#30586=CARTESIAN_POINT('Ctrl Pts',(36.8727100302512,15.3036390436952,15.));
#30587=CARTESIAN_POINT('Ctrl Pts',(36.7748254044502,15.2984606286737,15.));
#30588=CARTESIAN_POINT('Ctrl Pts',(36.6771206167755,15.2925717100767,15.));
#30589=CARTESIAN_POINT('Ctrl Pts',(36.5796108931244,15.2859343913094,15.));
#30590=CARTESIAN_POINT('Ctrl Pts',(36.4823116513289,15.2785104654792,15.));
#30591=CARTESIAN_POINT('Ctrl Pts',(36.3852352131887,15.2702711460937,15.));
#30592=CARTESIAN_POINT('Ctrl Pts',(36.2883880151607,15.2612053303773,15.));
#30593=CARTESIAN_POINT('Ctrl Pts',(36.1917659216814,15.2513334565427,15.));
#30594=CARTESIAN_POINT('Ctrl Pts',(36.095357546697,15.240697754828,15.));
#30595=CARTESIAN_POINT('Ctrl Pts',(35.9991531408727,15.2293360946131,15.));
#30596=CARTESIAN_POINT('Ctrl Pts',(35.9031525499277,15.2172585668056,15.));
#30597=CARTESIAN_POINT('Ctrl Pts',(35.8073720252878,15.2044274601769,15.));
#30598=CARTESIAN_POINT('Ctrl Pts',(35.7118553943773,15.1907243629659,15.));
#30599=CARTESIAN_POINT('Ctrl Pts',(35.6166644736253,15.1759785763051,15.));
#30600=CARTESIAN_POINT('Ctrl Pts',(35.5218591529745,15.1600260710384,15.));
#30601=CARTESIAN_POINT('Ctrl Pts',(35.4274792115856,15.1427632633831,15.));
#30602=CARTESIAN_POINT('Ctrl Pts',(35.3335286891314,15.1241934020681,15.));
#30603=CARTESIAN_POINT('Ctrl Pts',(35.2399506932815,15.104500806927,15.));
#30604=CARTESIAN_POINT('Ctrl Pts',(35.1466591020976,15.08395927165,15.));
#30605=CARTESIAN_POINT('Ctrl Pts',(35.0535882932913,15.0627878528202,15.));
#30606=CARTESIAN_POINT('Ctrl Pts',(34.9607388363587,15.041018569143,15.));
#30607=CARTESIAN_POINT('Ctrl Pts',(34.8682205930809,15.0183713484962,15.));
#30608=CARTESIAN_POINT('Ctrl Pts',(34.7763085406486,14.9940927023322,15.));
#30609=CARTESIAN_POINT('Ctrl Pts',(34.6853717911268,14.9671565602316,15.));
#30610=CARTESIAN_POINT('Ctrl Pts',(34.6137007885254,14.9426481276593,15.));
#30611=CARTESIAN_POINT('Ctrl Pts',(34.5606858566713,14.9222326355678,15.));
#30612=CARTESIAN_POINT('Ctrl Pts',(34.525687510388,14.9076710061311,15.));
#30613=CARTESIAN_POINT('Ctrl Pts',(34.5082745737944,14.9001523628048,15.));
#30614=CARTESIAN_POINT('',(41.3962265246839,14.9114864958881,0.));
#30615=CARTESIAN_POINT('Origin',(1.07784724682657E-11,3.50213800024364E-12,
0.));
#30616=CARTESIAN_POINT('',(42.2550026135057,12.2684454652018,0.));
#30617=CARTESIAN_POINT('Origin',(1.07784724682657E-11,3.50213800024364E-12,
0.));
#30618=CARTESIAN_POINT('',(42.2550026135057,12.2684454652018,15.));
#30619=CARTESIAN_POINT('Origin',(1.07784724682657E-11,3.50213800024364E-12,
15.));
#30620=CARTESIAN_POINT('',(42.2550026135057,12.2684454652018,0.));
#30621=CARTESIAN_POINT('Ctrl Pts',(36.6758703925241,8.22897839625061,0.));
#30622=CARTESIAN_POINT('Ctrl Pts',(36.6758703925241,8.22897839625061,18.));
#30623=CARTESIAN_POINT('Ctrl Pts',(36.6943771018148,8.23313075335376,0.));
#30624=CARTESIAN_POINT('Ctrl Pts',(36.6943771018148,8.23313075335376,18.));
#30625=CARTESIAN_POINT('Ctrl Pts',(36.7312504697652,8.24192165947367,0.));
#30626=CARTESIAN_POINT('Ctrl Pts',(36.7312504697652,8.24192165947367,18.));
#30627=CARTESIAN_POINT('Ctrl Pts',(36.7861403757604,8.2565665745182,0.));
#30628=CARTESIAN_POINT('Ctrl Pts',(36.7861403757604,8.2565665745182,18.));
#30629=CARTESIAN_POINT('Ctrl Pts',(36.8585291300917,8.27886599440785,0.));
#30630=CARTESIAN_POINT('Ctrl Pts',(36.8585291300917,8.27886599440785,18.));
#30631=CARTESIAN_POINT('Ctrl Pts',(36.9479311729484,8.31052547794591,0.));
#30632=CARTESIAN_POINT('Ctrl Pts',(36.9479311729484,8.31052547794591,18.));
#30633=CARTESIAN_POINT('Ctrl Pts',(37.0365602155148,8.34490818952639,0.));
#30634=CARTESIAN_POINT('Ctrl Pts',(37.0365602155148,8.34490818952639,18.));
#30635=CARTESIAN_POINT('Ctrl Pts',(37.1247207489179,8.38096706211448,0.));
#30636=CARTESIAN_POINT('Ctrl Pts',(37.1247207489179,8.38096706211448,18.));
#30637=CARTESIAN_POINT('Ctrl Pts',(37.2126332013933,8.4179308831326,0.));
#30638=CARTESIAN_POINT('Ctrl Pts',(37.2126332013933,8.4179308831326,18.));
#30639=CARTESIAN_POINT('Ctrl Pts',(37.3003733151561,8.4555084943396,0.));
#30640=CARTESIAN_POINT('Ctrl Pts',(37.3003733151561,8.4555084943396,18.));
#30641=CARTESIAN_POINT('Ctrl Pts',(37.3879218093514,8.49372546467076,0.));
#30642=CARTESIAN_POINT('Ctrl Pts',(37.3879218093514,8.49372546467076,18.));
#30643=CARTESIAN_POINT('Ctrl Pts',(37.4752030152968,8.53279758643784,0.));
#30644=CARTESIAN_POINT('Ctrl Pts',(37.4752030152968,8.53279758643784,18.));
#30645=CARTESIAN_POINT('Ctrl Pts',(37.5621256752108,8.57299698459465,0.));
#30646=CARTESIAN_POINT('Ctrl Pts',(37.5621256752108,8.57299698459465,18.));
#30647=CARTESIAN_POINT('Ctrl Pts',(37.6486274754754,8.61450621749155,0.));
#30648=CARTESIAN_POINT('Ctrl Pts',(37.6486274754754,8.61450621749155,18.));
#30649=CARTESIAN_POINT('Ctrl Pts',(37.7347032383719,8.65732553894524,0.));
#30650=CARTESIAN_POINT('Ctrl Pts',(37.7347032383719,8.65732553894524,18.));
#30651=CARTESIAN_POINT('Ctrl Pts',(37.8203816669031,8.70134776631143,0.));
#30652=CARTESIAN_POINT('Ctrl Pts',(37.8203816669031,8.70134776631143,18.));
#30653=CARTESIAN_POINT('Ctrl Pts',(37.9057107230066,8.74640499479002,0.));
#30654=CARTESIAN_POINT('Ctrl Pts',(37.9057107230066,8.74640499479002,18.));
#30655=CARTESIAN_POINT('Ctrl Pts',(37.9907407304174,8.79232279131092,0.));
#30656=CARTESIAN_POINT('Ctrl Pts',(37.9907407304174,8.79232279131092,18.));
#30657=CARTESIAN_POINT('Ctrl Pts',(38.0755058326913,8.83897959763349,0.));
#30658=CARTESIAN_POINT('Ctrl Pts',(38.0755058326913,8.83897959763349,18.));
#30659=CARTESIAN_POINT('Ctrl Pts',(38.1600150482528,8.88633535238434,0.));
#30660=CARTESIAN_POINT('Ctrl Pts',(38.1600150482528,8.88633535238434,18.));
#30661=CARTESIAN_POINT('Ctrl Pts',(38.2442625706309,8.93439830996339,0.));
#30662=CARTESIAN_POINT('Ctrl Pts',(38.2442625706309,8.93439830996339,18.));
#30663=CARTESIAN_POINT('Ctrl Pts',(38.3282340281403,8.9832048378576,0.));
#30664=CARTESIAN_POINT('Ctrl Pts',(38.3282340281403,8.9832048378576,18.));
#30665=CARTESIAN_POINT('Ctrl Pts',(38.4119138099805,9.03279579360191,0.));
#30666=CARTESIAN_POINT('Ctrl Pts',(38.4119138099805,9.03279579360191,18.));
#30667=CARTESIAN_POINT('Ctrl Pts',(38.4952932486131,9.08319014288086,0.));
#30668=CARTESIAN_POINT('Ctrl Pts',(38.4952932486131,9.08319014288086,18.));
#30669=CARTESIAN_POINT('Ctrl Pts',(38.5783736628826,9.13437512010586,0.));
#30670=CARTESIAN_POINT('Ctrl Pts',(38.5783736628826,9.13437512010586,18.));
#30671=CARTESIAN_POINT('Ctrl Pts',(38.6611620045193,9.1863201939433,0.));
#30672=CARTESIAN_POINT('Ctrl Pts',(38.6611620045193,9.1863201939433,18.));
#30673=CARTESIAN_POINT('Ctrl Pts',(38.7436682576832,9.23898539199331,0.));
#30674=CARTESIAN_POINT('Ctrl Pts',(38.7436682576832,9.23898539199331,18.));
#30675=CARTESIAN_POINT('Ctrl Pts',(38.8259023794241,9.29233110570903,0.));
#30676=CARTESIAN_POINT('Ctrl Pts',(38.8259023794241,9.29233110570903,18.));
#30677=CARTESIAN_POINT('Ctrl Pts',(38.9078708427078,9.34632917154637,0.));
#30678=CARTESIAN_POINT('Ctrl Pts',(38.9078708427078,9.34632917154637,18.));
#30679=CARTESIAN_POINT('Ctrl Pts',(38.9895756526779,9.40096600877644,0.));
#30680=CARTESIAN_POINT('Ctrl Pts',(38.9895756526779,9.40096600877644,18.));
#30681=CARTESIAN_POINT('Ctrl Pts',(39.0710161994951,9.45623664577431,0.));
#30682=CARTESIAN_POINT('Ctrl Pts',(39.0710161994951,9.45623664577431,18.));
#30683=CARTESIAN_POINT('Ctrl Pts',(39.1521903958955,9.51214104535621,0.));
#30684=CARTESIAN_POINT('Ctrl Pts',(39.1521903958955,9.51214104535621,18.));
#30685=CARTESIAN_POINT('Ctrl Pts',(39.2330959982788,9.56867984233623,0.));
#30686=CARTESIAN_POINT('Ctrl Pts',(39.2330959982788,9.56867984233623,18.));
#30687=CARTESIAN_POINT('Ctrl Pts',(39.3137321153686,9.62584947846543,0.));
#30688=CARTESIAN_POINT('Ctrl Pts',(39.3137321153686,9.62584947846543,18.));
#30689=CARTESIAN_POINT('Ctrl Pts',(39.3940995760289,9.68364100883826,0.));
#30690=CARTESIAN_POINT('Ctrl Pts',(39.3940995760289,9.68364100883826,18.));
#30691=CARTESIAN_POINT('Ctrl Pts',(39.4742001555227,9.74204258152663,0.));
#30692=CARTESIAN_POINT('Ctrl Pts',(39.4742001555227,9.74204258152663,18.));
#30693=CARTESIAN_POINT('Ctrl Pts',(39.5540361022309,9.80104095251613,0.));
#30694=CARTESIAN_POINT('Ctrl Pts',(39.5540361022309,9.80104095251613,18.));
#30695=CARTESIAN_POINT('Ctrl Pts',(39.6336095893767,9.86062324242559,0.));
#30696=CARTESIAN_POINT('Ctrl Pts',(39.6336095893767,9.86062324242559,18.));
#30697=CARTESIAN_POINT('Ctrl Pts',(39.712922089547,9.92077894513191,0.));
#30698=CARTESIAN_POINT('Ctrl Pts',(39.712922089547,9.92077894513191,18.));
#30699=CARTESIAN_POINT('Ctrl Pts',(39.7919742367922,9.98150036150823,0.));
#30700=CARTESIAN_POINT('Ctrl Pts',(39.7919742367922,9.98150036150823,18.));
#30701=CARTESIAN_POINT('Ctrl Pts',(39.8707661565233,10.0427815229883,0.));
#30702=CARTESIAN_POINT('Ctrl Pts',(39.8707661565233,10.0427815229883,18.));
#30703=CARTESIAN_POINT('Ctrl Pts',(39.9492976736738,10.1046175096878,0.));
#30704=CARTESIAN_POINT('Ctrl Pts',(39.9492976736738,10.1046175096878,18.));
#30705=CARTESIAN_POINT('Ctrl Pts',(40.0275685525923,10.1670036683795,0.));
#30706=CARTESIAN_POINT('Ctrl Pts',(40.0275685525923,10.1670036683795,18.));
#30707=CARTESIAN_POINT('Ctrl Pts',(40.1055787732578,10.2299347125857,0.));
#30708=CARTESIAN_POINT('Ctrl Pts',(40.1055787732578,10.2299347125857,18.));
#30709=CARTESIAN_POINT('Ctrl Pts',(40.1833286010098,10.2934044990237,0.));
#30710=CARTESIAN_POINT('Ctrl Pts',(40.1833286010098,10.2934044990237,18.));
#30711=CARTESIAN_POINT('Ctrl Pts',(40.2608184485326,10.3574064830678,0.));
#30712=CARTESIAN_POINT('Ctrl Pts',(40.2608184485326,10.3574064830678,18.));
#30713=CARTESIAN_POINT('Ctrl Pts',(40.3380487942952,10.421933993295,0.));
#30714=CARTESIAN_POINT('Ctrl Pts',(40.3380487942952,10.421933993295,18.));
#30715=CARTESIAN_POINT('Ctrl Pts',(40.4150200869536,10.48698054978,0.));
#30716=CARTESIAN_POINT('Ctrl Pts',(40.4150200869536,10.48698054978,18.));
#30717=CARTESIAN_POINT('Ctrl Pts',(40.4917326404439,10.5525402237951,0.));
#30718=CARTESIAN_POINT('Ctrl Pts',(40.4917326404439,10.5525402237951,18.));
#30719=CARTESIAN_POINT('Ctrl Pts',(40.5681866012103,10.618607730849,0.));
#30720=CARTESIAN_POINT('Ctrl Pts',(40.5681866012103,10.618607730849,18.));
#30721=CARTESIAN_POINT('Ctrl Pts',(40.6443819999244,10.6851782157325,0.));
#30722=CARTESIAN_POINT('Ctrl Pts',(40.6443819999244,10.6851782157325,18.));
#30723=CARTESIAN_POINT('Ctrl Pts',(40.7203187831783,10.7522471109694,0.));
#30724=CARTESIAN_POINT('Ctrl Pts',(40.7203187831783,10.7522471109694,18.));
#30725=CARTESIAN_POINT('Ctrl Pts',(40.795996852756,10.8198099757795,0.));
#30726=CARTESIAN_POINT('Ctrl Pts',(40.795996852756,10.8198099757795,18.));
#30727=CARTESIAN_POINT('Ctrl Pts',(40.8714161092412,10.8878623066646,0.));
#30728=CARTESIAN_POINT('Ctrl Pts',(40.8714161092412,10.8878623066646,18.));
#30729=CARTESIAN_POINT('Ctrl Pts',(40.9465764747798,10.956399476781,0.));
#30730=CARTESIAN_POINT('Ctrl Pts',(40.9465764747798,10.956399476781,18.));
#30731=CARTESIAN_POINT('Ctrl Pts',(41.0214778832142,11.0254168609972,0.));
#30732=CARTESIAN_POINT('Ctrl Pts',(41.0214778832142,11.0254168609972,18.));
#30733=CARTESIAN_POINT('Ctrl Pts',(41.0961202807715,11.0949099155251,0.));
#30734=CARTESIAN_POINT('Ctrl Pts',(41.0961202807715,11.0949099155251,18.));
#30735=CARTESIAN_POINT('Ctrl Pts',(41.1705036228854,11.1648742640378,0.));
#30736=CARTESIAN_POINT('Ctrl Pts',(41.1705036228854,11.1648742640378,18.));
#30737=CARTESIAN_POINT('Ctrl Pts',(41.2446278781981,11.2353057980338,0.));
#30738=CARTESIAN_POINT('Ctrl Pts',(41.2446278781981,11.2353057980338,18.));
#30739=CARTESIAN_POINT('Ctrl Pts',(41.3184930194148,11.3062006993745,0.));
#30740=CARTESIAN_POINT('Ctrl Pts',(41.3184930194148,11.3062006993745,18.));
#30741=CARTESIAN_POINT('Ctrl Pts',(41.3920989905986,11.3775553120176,0.));
#30742=CARTESIAN_POINT('Ctrl Pts',(41.3920989905986,11.3775553120176,18.));
#30743=CARTESIAN_POINT('Ctrl Pts',(41.4654456796071,11.4493660393849,0.));
#30744=CARTESIAN_POINT('Ctrl Pts',(41.4654456796071,11.4493660393849,18.));
#30745=CARTESIAN_POINT('Ctrl Pts',(41.5385328935506,11.5216292382388,0.));
#30746=CARTESIAN_POINT('Ctrl Pts',(41.5385328935506,11.5216292382388,18.));
#30747=CARTESIAN_POINT('Ctrl Pts',(41.6113603270596,11.5943410868252,0.));
#30748=CARTESIAN_POINT('Ctrl Pts',(41.6113603270596,11.5943410868252,18.));
#30749=CARTESIAN_POINT('Ctrl Pts',(41.6839275596248,11.6674975352851,0.));
#30750=CARTESIAN_POINT('Ctrl Pts',(41.6839275596248,11.6674975352851,18.));
#30751=CARTESIAN_POINT('Ctrl Pts',(41.7562341395977,11.7410945211992,0.));
#30752=CARTESIAN_POINT('Ctrl Pts',(41.7562341395977,11.7410945211992,18.));
#30753=CARTESIAN_POINT('Ctrl Pts',(41.8282796562569,11.81512813804,0.));
#30754=CARTESIAN_POINT('Ctrl Pts',(41.8282796562569,11.81512813804,18.));
#30755=CARTESIAN_POINT('Ctrl Pts',(41.9000638152266,11.8895948153349,0.));
#30756=CARTESIAN_POINT('Ctrl Pts',(41.9000638152266,11.8895948153349,18.));
#30757=CARTESIAN_POINT('Ctrl Pts',(41.9715865222182,11.9644914999263,0.));
#30758=CARTESIAN_POINT('Ctrl Pts',(41.9715865222182,11.9644914999263,18.));
#30759=CARTESIAN_POINT('Ctrl Pts',(42.0428479428228,12.0398158079102,0.));
#30760=CARTESIAN_POINT('Ctrl Pts',(42.0428479428228,12.0398158079102,18.));
#30761=CARTESIAN_POINT('Ctrl Pts',(42.1138483839101,12.1155659644537,0.));
#30762=CARTESIAN_POINT('Ctrl Pts',(42.1138483839101,12.1155659644537,18.));
#30763=CARTESIAN_POINT('Ctrl Pts',(42.1704402333854,12.1765058047069,0.));
#30764=CARTESIAN_POINT('Ctrl Pts',(42.1704402333854,12.1765058047069,18.));
#30765=CARTESIAN_POINT('Ctrl Pts',(42.2127669677092,12.222401466668,0.));
#30766=CARTESIAN_POINT('Ctrl Pts',(42.2127669677092,12.222401466668,18.));
#30767=CARTESIAN_POINT('Ctrl Pts',(42.2409327400055,12.2530833383985,0.));
#30768=CARTESIAN_POINT('Ctrl Pts',(42.2409327400055,12.2530833383985,18.));
#30769=CARTESIAN_POINT('Ctrl Pts',(42.2550026135057,12.2684454652018,0.));
#30770=CARTESIAN_POINT('Ctrl Pts',(42.2550026135057,12.2684454652018,18.));
#30771=CARTESIAN_POINT('Ctrl Pts',(36.6758703925241,8.22897839625061,0.));
#30772=CARTESIAN_POINT('Ctrl Pts',(36.6943771018148,8.23313075335376,0.));
#30773=CARTESIAN_POINT('Ctrl Pts',(36.7312504697652,8.24192165947367,0.));
#30774=CARTESIAN_POINT('Ctrl Pts',(36.7861403757604,8.2565665745182,0.));
#30775=CARTESIAN_POINT('Ctrl Pts',(36.8585291300917,8.27886599440785,0.));
#30776=CARTESIAN_POINT('Ctrl Pts',(36.9479311729484,8.31052547794591,0.));
#30777=CARTESIAN_POINT('Ctrl Pts',(37.0365602155148,8.34490818952639,0.));
#30778=CARTESIAN_POINT('Ctrl Pts',(37.1247207489179,8.38096706211448,0.));
#30779=CARTESIAN_POINT('Ctrl Pts',(37.2126332013933,8.4179308831326,0.));
#30780=CARTESIAN_POINT('Ctrl Pts',(37.3003733151561,8.4555084943396,0.));
#30781=CARTESIAN_POINT('Ctrl Pts',(37.3879218093514,8.49372546467076,0.));
#30782=CARTESIAN_POINT('Ctrl Pts',(37.4752030152968,8.53279758643784,0.));
#30783=CARTESIAN_POINT('Ctrl Pts',(37.5621256752108,8.57299698459465,0.));
#30784=CARTESIAN_POINT('Ctrl Pts',(37.6486274754754,8.61450621749155,0.));
#30785=CARTESIAN_POINT('Ctrl Pts',(37.7347032383719,8.65732553894524,0.));
#30786=CARTESIAN_POINT('Ctrl Pts',(37.8203816669031,8.70134776631143,0.));
#30787=CARTESIAN_POINT('Ctrl Pts',(37.9057107230066,8.74640499479002,0.));
#30788=CARTESIAN_POINT('Ctrl Pts',(37.9907407304174,8.79232279131092,0.));
#30789=CARTESIAN_POINT('Ctrl Pts',(38.0755058326913,8.83897959763349,0.));
#30790=CARTESIAN_POINT('Ctrl Pts',(38.1600150482528,8.88633535238434,0.));
#30791=CARTESIAN_POINT('Ctrl Pts',(38.2442625706309,8.93439830996339,0.));
#30792=CARTESIAN_POINT('Ctrl Pts',(38.3282340281403,8.9832048378576,0.));
#30793=CARTESIAN_POINT('Ctrl Pts',(38.4119138099805,9.03279579360191,0.));
#30794=CARTESIAN_POINT('Ctrl Pts',(38.4952932486131,9.08319014288086,0.));
#30795=CARTESIAN_POINT('Ctrl Pts',(38.5783736628826,9.13437512010586,0.));
#30796=CARTESIAN_POINT('Ctrl Pts',(38.6611620045193,9.1863201939433,0.));
#30797=CARTESIAN_POINT('Ctrl Pts',(38.7436682576832,9.23898539199331,0.));
#30798=CARTESIAN_POINT('Ctrl Pts',(38.8259023794241,9.29233110570903,0.));
#30799=CARTESIAN_POINT('Ctrl Pts',(38.9078708427078,9.34632917154637,0.));
#30800=CARTESIAN_POINT('Ctrl Pts',(38.9895756526779,9.40096600877644,0.));
#30801=CARTESIAN_POINT('Ctrl Pts',(39.0710161994951,9.45623664577431,0.));
#30802=CARTESIAN_POINT('Ctrl Pts',(39.1521903958955,9.51214104535621,0.));
#30803=CARTESIAN_POINT('Ctrl Pts',(39.2330959982788,9.56867984233623,0.));
#30804=CARTESIAN_POINT('Ctrl Pts',(39.3137321153686,9.62584947846543,0.));
#30805=CARTESIAN_POINT('Ctrl Pts',(39.3940995760289,9.68364100883826,0.));
#30806=CARTESIAN_POINT('Ctrl Pts',(39.4742001555227,9.74204258152663,0.));
#30807=CARTESIAN_POINT('Ctrl Pts',(39.5540361022309,9.80104095251613,0.));
#30808=CARTESIAN_POINT('Ctrl Pts',(39.6336095893767,9.86062324242559,0.));
#30809=CARTESIAN_POINT('Ctrl Pts',(39.712922089547,9.92077894513191,0.));
#30810=CARTESIAN_POINT('Ctrl Pts',(39.7919742367922,9.98150036150823,0.));
#30811=CARTESIAN_POINT('Ctrl Pts',(39.8707661565233,10.0427815229883,0.));
#30812=CARTESIAN_POINT('Ctrl Pts',(39.9492976736738,10.1046175096878,0.));
#30813=CARTESIAN_POINT('Ctrl Pts',(40.0275685525923,10.1670036683795,0.));
#30814=CARTESIAN_POINT('Ctrl Pts',(40.1055787732578,10.2299347125857,0.));
#30815=CARTESIAN_POINT('Ctrl Pts',(40.1833286010098,10.2934044990237,0.));
#30816=CARTESIAN_POINT('Ctrl Pts',(40.2608184485326,10.3574064830678,0.));
#30817=CARTESIAN_POINT('Ctrl Pts',(40.3380487942952,10.421933993295,0.));
#30818=CARTESIAN_POINT('Ctrl Pts',(40.4150200869536,10.48698054978,0.));
#30819=CARTESIAN_POINT('Ctrl Pts',(40.4917326404439,10.5525402237951,0.));
#30820=CARTESIAN_POINT('Ctrl Pts',(40.5681866012103,10.618607730849,0.));
#30821=CARTESIAN_POINT('Ctrl Pts',(40.6443819999244,10.6851782157325,0.));
#30822=CARTESIAN_POINT('Ctrl Pts',(40.7203187831783,10.7522471109694,0.));
#30823=CARTESIAN_POINT('Ctrl Pts',(40.795996852756,10.8198099757795,0.));
#30824=CARTESIAN_POINT('Ctrl Pts',(40.8714161092412,10.8878623066646,0.));
#30825=CARTESIAN_POINT('Ctrl Pts',(40.9465764747798,10.956399476781,0.));
#30826=CARTESIAN_POINT('Ctrl Pts',(41.0214778832142,11.0254168609972,0.));
#30827=CARTESIAN_POINT('Ctrl Pts',(41.0961202807715,11.0949099155251,0.));
#30828=CARTESIAN_POINT('Ctrl Pts',(41.1705036228854,11.1648742640378,0.));
#30829=CARTESIAN_POINT('Ctrl Pts',(41.2446278781981,11.2353057980338,0.));
#30830=CARTESIAN_POINT('Ctrl Pts',(41.3184930194148,11.3062006993745,0.));
#30831=CARTESIAN_POINT('Ctrl Pts',(41.3920989905986,11.3775553120176,0.));
#30832=CARTESIAN_POINT('Ctrl Pts',(41.4654456796071,11.4493660393849,0.));
#30833=CARTESIAN_POINT('Ctrl Pts',(41.5385328935506,11.5216292382388,0.));
#30834=CARTESIAN_POINT('Ctrl Pts',(41.6113603270596,11.5943410868252,0.));
#30835=CARTESIAN_POINT('Ctrl Pts',(41.6839275596248,11.6674975352851,0.));
#30836=CARTESIAN_POINT('Ctrl Pts',(41.7562341395977,11.7410945211992,0.));
#30837=CARTESIAN_POINT('Ctrl Pts',(41.8282796562569,11.81512813804,0.));
#30838=CARTESIAN_POINT('Ctrl Pts',(41.9000638152266,11.8895948153349,0.));
#30839=CARTESIAN_POINT('Ctrl Pts',(41.9715865222182,11.9644914999263,0.));
#30840=CARTESIAN_POINT('Ctrl Pts',(42.0571002269437,12.054880669507,0.));
#30841=CARTESIAN_POINT('Ctrl Pts',(42.1280354231517,12.1307372881904,0.));
#30842=CARTESIAN_POINT('Ctrl Pts',(42.18457517013,12.1917619768791,0.));
#30843=CARTESIAN_POINT('Ctrl Pts',(42.2268628664988,12.2377212115625,0.));
#30844=CARTESIAN_POINT('Ctrl Pts',(42.2550026135057,12.2684454652018,0.));
#30845=CARTESIAN_POINT('Ctrl Pts',(36.6758703925241,8.22897839625061,15.));
#30846=CARTESIAN_POINT('Ctrl Pts',(36.6943771018148,8.23313075335376,15.));
#30847=CARTESIAN_POINT('Ctrl Pts',(36.7312504697652,8.24192165947367,15.));
#30848=CARTESIAN_POINT('Ctrl Pts',(36.7861403757604,8.2565665745182,15.));
#30849=CARTESIAN_POINT('Ctrl Pts',(36.8585291300917,8.27886599440785,15.));
#30850=CARTESIAN_POINT('Ctrl Pts',(36.9479311729484,8.31052547794591,15.));
#30851=CARTESIAN_POINT('Ctrl Pts',(37.0365602155148,8.34490818952639,15.));
#30852=CARTESIAN_POINT('Ctrl Pts',(37.1247207489179,8.38096706211448,15.));
#30853=CARTESIAN_POINT('Ctrl Pts',(37.2126332013933,8.4179308831326,15.));
#30854=CARTESIAN_POINT('Ctrl Pts',(37.3003733151561,8.4555084943396,15.));
#30855=CARTESIAN_POINT('Ctrl Pts',(37.3879218093514,8.49372546467076,15.));
#30856=CARTESIAN_POINT('Ctrl Pts',(37.4752030152968,8.53279758643784,15.));
#30857=CARTESIAN_POINT('Ctrl Pts',(37.5621256752108,8.57299698459465,15.));
#30858=CARTESIAN_POINT('Ctrl Pts',(37.6486274754754,8.61450621749155,15.));
#30859=CARTESIAN_POINT('Ctrl Pts',(37.7347032383719,8.65732553894524,15.));
#30860=CARTESIAN_POINT('Ctrl Pts',(37.8203816669031,8.70134776631143,15.));
#30861=CARTESIAN_POINT('Ctrl Pts',(37.9057107230066,8.74640499479002,15.));
#30862=CARTESIAN_POINT('Ctrl Pts',(37.9907407304174,8.79232279131092,15.));
#30863=CARTESIAN_POINT('Ctrl Pts',(38.0755058326913,8.83897959763349,15.));
#30864=CARTESIAN_POINT('Ctrl Pts',(38.1600150482528,8.88633535238434,15.));
#30865=CARTESIAN_POINT('Ctrl Pts',(38.2442625706309,8.93439830996339,15.));
#30866=CARTESIAN_POINT('Ctrl Pts',(38.3282340281403,8.9832048378576,15.));
#30867=CARTESIAN_POINT('Ctrl Pts',(38.4119138099805,9.03279579360191,15.));
#30868=CARTESIAN_POINT('Ctrl Pts',(38.4952932486131,9.08319014288086,15.));
#30869=CARTESIAN_POINT('Ctrl Pts',(38.5783736628826,9.13437512010586,15.));
#30870=CARTESIAN_POINT('Ctrl Pts',(38.6611620045193,9.1863201939433,15.));
#30871=CARTESIAN_POINT('Ctrl Pts',(38.7436682576832,9.23898539199331,15.));
#30872=CARTESIAN_POINT('Ctrl Pts',(38.8259023794241,9.29233110570903,15.));
#30873=CARTESIAN_POINT('Ctrl Pts',(38.9078708427078,9.34632917154637,15.));
#30874=CARTESIAN_POINT('Ctrl Pts',(38.9895756526779,9.40096600877644,15.));
#30875=CARTESIAN_POINT('Ctrl Pts',(39.0710161994951,9.45623664577431,15.));
#30876=CARTESIAN_POINT('Ctrl Pts',(39.1521903958955,9.51214104535621,15.));
#30877=CARTESIAN_POINT('Ctrl Pts',(39.2330959982788,9.56867984233623,15.));
#30878=CARTESIAN_POINT('Ctrl Pts',(39.3137321153686,9.62584947846543,15.));
#30879=CARTESIAN_POINT('Ctrl Pts',(39.3940995760289,9.68364100883826,15.));
#30880=CARTESIAN_POINT('Ctrl Pts',(39.4742001555227,9.74204258152663,15.));
#30881=CARTESIAN_POINT('Ctrl Pts',(39.5540361022309,9.80104095251613,15.));
#30882=CARTESIAN_POINT('Ctrl Pts',(39.6336095893767,9.86062324242559,15.));
#30883=CARTESIAN_POINT('Ctrl Pts',(39.712922089547,9.92077894513191,15.));
#30884=CARTESIAN_POINT('Ctrl Pts',(39.7919742367922,9.98150036150823,15.));
#30885=CARTESIAN_POINT('Ctrl Pts',(39.8707661565233,10.0427815229883,15.));
#30886=CARTESIAN_POINT('Ctrl Pts',(39.9492976736738,10.1046175096878,15.));
#30887=CARTESIAN_POINT('Ctrl Pts',(40.0275685525923,10.1670036683795,15.));
#30888=CARTESIAN_POINT('Ctrl Pts',(40.1055787732578,10.2299347125857,15.));
#30889=CARTESIAN_POINT('Ctrl Pts',(40.1833286010098,10.2934044990237,15.));
#30890=CARTESIAN_POINT('Ctrl Pts',(40.2608184485326,10.3574064830678,15.));
#30891=CARTESIAN_POINT('Ctrl Pts',(40.3380487942952,10.421933993295,15.));
#30892=CARTESIAN_POINT('Ctrl Pts',(40.4150200869536,10.48698054978,15.));
#30893=CARTESIAN_POINT('Ctrl Pts',(40.4917326404439,10.5525402237951,15.));
#30894=CARTESIAN_POINT('Ctrl Pts',(40.5681866012103,10.618607730849,15.));
#30895=CARTESIAN_POINT('Ctrl Pts',(40.6443819999244,10.6851782157325,15.));
#30896=CARTESIAN_POINT('Ctrl Pts',(40.7203187831783,10.7522471109694,15.));
#30897=CARTESIAN_POINT('Ctrl Pts',(40.795996852756,10.8198099757795,15.));
#30898=CARTESIAN_POINT('Ctrl Pts',(40.8714161092412,10.8878623066646,15.));
#30899=CARTESIAN_POINT('Ctrl Pts',(40.9465764747798,10.956399476781,15.));
#30900=CARTESIAN_POINT('Ctrl Pts',(41.0214778832142,11.0254168609972,15.));
#30901=CARTESIAN_POINT('Ctrl Pts',(41.0961202807715,11.0949099155251,15.));
#30902=CARTESIAN_POINT('Ctrl Pts',(41.1705036228854,11.1648742640378,15.));
#30903=CARTESIAN_POINT('Ctrl Pts',(41.2446278781981,11.2353057980338,15.));
#30904=CARTESIAN_POINT('Ctrl Pts',(41.3184930194148,11.3062006993745,15.));
#30905=CARTESIAN_POINT('Ctrl Pts',(41.3920989905986,11.3775553120176,15.));
#30906=CARTESIAN_POINT('Ctrl Pts',(41.4654456796071,11.4493660393849,15.));
#30907=CARTESIAN_POINT('Ctrl Pts',(41.5385328935506,11.5216292382388,15.));
#30908=CARTESIAN_POINT('Ctrl Pts',(41.6113603270596,11.5943410868252,15.));
#30909=CARTESIAN_POINT('Ctrl Pts',(41.6839275596248,11.6674975352851,15.));
#30910=CARTESIAN_POINT('Ctrl Pts',(41.7562341395977,11.7410945211992,15.));
#30911=CARTESIAN_POINT('Ctrl Pts',(41.8282796562569,11.81512813804,15.));
#30912=CARTESIAN_POINT('Ctrl Pts',(41.9000638152266,11.8895948153349,15.));
#30913=CARTESIAN_POINT('Ctrl Pts',(41.9715865222182,11.9644914999263,15.));
#30914=CARTESIAN_POINT('Ctrl Pts',(42.0571002269437,12.054880669507,15.));
#30915=CARTESIAN_POINT('Ctrl Pts',(42.1280354231517,12.1307372881904,15.));
#30916=CARTESIAN_POINT('Ctrl Pts',(42.18457517013,12.1917619768791,15.));
#30917=CARTESIAN_POINT('Ctrl Pts',(42.2268628664988,12.2377212115625,15.));
#30918=CARTESIAN_POINT('Ctrl Pts',(42.2550026135057,12.2684454652018,15.));
#30919=CARTESIAN_POINT('Origin',(0.,0.,0.));
#30920=CARTESIAN_POINT('Origin',(0.,0.,0.));
#30921=CARTESIAN_POINT('Origin',(0.,0.,0.));
#30922=CARTESIAN_POINT('Origin',(0.,0.,0.));
#30923=CARTESIAN_POINT('Origin',(0.,0.,0.));
#30924=CARTESIAN_POINT('Origin',(0.,0.,0.));
#30925=CARTESIAN_POINT('Origin',(0.,0.,0.));
#30926=CARTESIAN_POINT('Origin',(0.,0.,0.));
#30927=CARTESIAN_POINT('Origin',(0.,0.,0.));
#30928=CARTESIAN_POINT('Origin',(0.,0.,0.));
#30929=CARTESIAN_POINT('Origin',(0.,0.,0.));
#30930=CARTESIAN_POINT('Origin',(0.,0.,0.));
#30931=CARTESIAN_POINT('Origin',(0.,0.,0.));
#30932=CARTESIAN_POINT('Origin',(0.,0.,0.));
#30933=CARTESIAN_POINT('Origin',(0.,0.,0.));
#30934=CARTESIAN_POINT('Origin',(0.,0.,0.));
#30935=CARTESIAN_POINT('Origin',(0.,0.,0.));
#30936=CARTESIAN_POINT('Origin',(0.,0.,0.));
#30937=CARTESIAN_POINT('',(35.1136254352094,4.26751599830831,0.));
#30938=CARTESIAN_POINT('Origin',(0.,0.,0.));
#30939=CARTESIAN_POINT('',(36.199629211057,3.39252545782466,0.));
#30940=CARTESIAN_POINT('Origin',(36.1063209411239,4.38816272448461,0.));
#30941=CARTESIAN_POINT('',(37.4237196983922,3.50724370857673,0.));
#30942=CARTESIAN_POINT('',(35.2077250236291,3.2995670413737,0.));
#30943=CARTESIAN_POINT('',(43.9780537249529,1.38952890043929,0.));
#30944=CARTESIAN_POINT('Ctrl Pts',(37.4237196983922,3.50724370857673,0.));
#30945=CARTESIAN_POINT('Ctrl Pts',(37.4426037737699,3.50901346997657,0.));
#30946=CARTESIAN_POINT('Ctrl Pts',(37.4803889700239,3.51204731876361,0.));
#30947=CARTESIAN_POINT('Ctrl Pts',(37.5371179004295,3.5150810906521,0.));
#30948=CARTESIAN_POINT('Ctrl Pts',(37.6128545966533,3.51624243734645,0.));
#30949=CARTESIAN_POINT('Ctrl Pts',(37.7076643105286,3.51375922979957,0.));
#30950=CARTESIAN_POINT('Ctrl Pts',(37.8025803811856,3.50844720825128,0.));
#30951=CARTESIAN_POINT('Ctrl Pts',(37.8975688353863,3.50139628556084,0.));
#30952=CARTESIAN_POINT('Ctrl Pts',(37.9926009950482,3.49340804454645,0.));
#30953=CARTESIAN_POINT('Ctrl Pts',(38.0876589224537,3.48478279878233,0.));
#30954=CARTESIAN_POINT('Ctrl Pts',(38.1827321816559,3.47549027265411,0.));
#30955=CARTESIAN_POINT('Ctrl Pts',(38.2778154909527,3.46530185256872,0.));
#30956=CARTESIAN_POINT('Ctrl Pts',(38.3729061502716,3.45393053211023,0.));
#30957=CARTESIAN_POINT('Ctrl Pts',(38.4680013094732,3.44118343200303,0.));
#30958=CARTESIAN_POINT('Ctrl Pts',(38.5630961226878,3.42705871084997,0.));
#30959=CARTESIAN_POINT('Ctrl Pts',(38.6581847668347,3.41166717511901,0.));
#30960=CARTESIAN_POINT('Ctrl Pts',(38.7532609709905,3.39518333281818,0.));
#30961=CARTESIAN_POINT('Ctrl Pts',(38.8483186930884,3.37778863054482,0.));
#30962=CARTESIAN_POINT('Ctrl Pts',(38.9433528420174,3.35960922799481,0.));
#30963=CARTESIAN_POINT('Ctrl Pts',(39.0383596151636,3.34068601264472,0.));
#30964=CARTESIAN_POINT('Ctrl Pts',(39.1333360409949,3.32100933979557,0.));
#30965=CARTESIAN_POINT('Ctrl Pts',(39.2282796893977,3.30054018081687,0.));
#30966=CARTESIAN_POINT('Ctrl Pts',(39.3231883392913,3.27923485388117,0.));
#30967=CARTESIAN_POINT('Ctrl Pts',(39.4180596080755,3.25707264313388,0.));
#30968=CARTESIAN_POINT('Ctrl Pts',(39.5128908052622,3.23406609691661,0.));
#30969=CARTESIAN_POINT('Ctrl Pts',(39.607679107639,3.21024640045595,0.));
#30970=CARTESIAN_POINT('Ctrl Pts',(39.7024216585552,3.18565465503835,0.));
#30971=CARTESIAN_POINT('Ctrl Pts',(39.7971156880138,3.16033160752804,0.));
#30972=CARTESIAN_POINT('Ctrl Pts',(39.8917586491576,3.13430604330356,0.));
#30973=CARTESIAN_POINT('Ctrl Pts',(39.9863482523153,3.10759149802908,0.));
#30974=CARTESIAN_POINT('Ctrl Pts',(40.0808823811787,3.08019251155015,0.));
#30975=CARTESIAN_POINT('Ctrl Pts',(40.1753590391515,3.05210847423071,0.));
#30976=CARTESIAN_POINT('Ctrl Pts',(40.2697762886113,3.02333808901595,0.));
#30977=CARTESIAN_POINT('Ctrl Pts',(40.3641321823444,2.9938844645822,0.));
#30978=CARTESIAN_POINT('Ctrl Pts',(40.4584247445196,2.96375636417323,0.));
#30979=CARTESIAN_POINT('Ctrl Pts',(40.5526520010651,2.93296560822894,0.));
#30980=CARTESIAN_POINT('Ctrl Pts',(40.6468119976928,2.90152548734343,0.));
#30981=CARTESIAN_POINT('Ctrl Pts',(40.7409028213129,2.86944892209898,0.));
#30982=CARTESIAN_POINT('Ctrl Pts',(40.8349226258683,2.83674635946679,0.));
#30983=CARTESIAN_POINT('Ctrl Pts',(40.9288696352159,2.80342531768405,0.));
#30984=CARTESIAN_POINT('Ctrl Pts',(41.0227421242398,2.76949151194863,0.));
#30985=CARTESIAN_POINT('Ctrl Pts',(41.1165384061145,2.73494956725006,0.));
#30986=CARTESIAN_POINT('Ctrl Pts',(41.2102568187956,2.69980383625016,0.));
#30987=CARTESIAN_POINT('Ctrl Pts',(41.3038957096306,2.66405934050118,0.));
#30988=CARTESIAN_POINT('Ctrl Pts',(41.3974534325936,2.62772200460656,0.));
#30989=CARTESIAN_POINT('Ctrl Pts',(41.4909283577703,2.59079818040172,0.));
#30990=CARTESIAN_POINT('Ctrl Pts',(41.5843188786284,2.55329436064184,0.));
#30991=CARTESIAN_POINT('Ctrl Pts',(41.6776234194583,2.51521684674477,0.));
#30992=CARTESIAN_POINT('Ctrl Pts',(41.7708404467532,2.47657137427693,0.));
#30993=CARTESIAN_POINT('Ctrl Pts',(41.8639684667923,2.43736301434201,0.));
#30994=CARTESIAN_POINT('Ctrl Pts',(41.9570060084039,2.39759639399648,0.));
#30995=CARTESIAN_POINT('Ctrl Pts',(42.0499516093661,2.35727584066429,0.));
#30996=CARTESIAN_POINT('Ctrl Pts',(42.1428038039937,2.31640554742809,0.));
#30997=CARTESIAN_POINT('Ctrl Pts',(42.2355611060784,2.27498976664775,0.));
#30998=CARTESIAN_POINT('Ctrl Pts',(42.3282220118033,2.233032874655,0.));
#30999=CARTESIAN_POINT('Ctrl Pts',(42.4207850290047,2.19053924976738,0.));
#31000=CARTESIAN_POINT('Ctrl Pts',(42.5132487024335,2.14751319676745,0.));
#31001=CARTESIAN_POINT('Ctrl Pts',(42.6056116373455,2.10395886401771,0.));
#31002=CARTESIAN_POINT('Ctrl Pts',(42.6978725343209,2.05988014924519,0.));
#31003=CARTESIAN_POINT('Ctrl Pts',(42.7900301875309,2.0152806752809,0.));
#31004=CARTESIAN_POINT('Ctrl Pts',(42.8820834139973,1.97016390194216,0.));
#31005=CARTESIAN_POINT('Ctrl Pts',(42.9740309956624,1.92453321512436,0.));
#31006=CARTESIAN_POINT('Ctrl Pts',(43.065871623255,1.87839202014609,0.));
#31007=CARTESIAN_POINT('Ctrl Pts',(43.1576038253643,1.83174385734712,0.));
#31008=CARTESIAN_POINT('Ctrl Pts',(43.2492259505872,1.7845924484277,0.));
#31009=CARTESIAN_POINT('Ctrl Pts',(43.3407363140236,1.73694151741124,0.));
#31010=CARTESIAN_POINT('Ctrl Pts',(43.4321333178711,1.68879465270608,0.));
#31011=CARTESIAN_POINT('Ctrl Pts',(43.5234155788248,1.64015515906648,0.));
#31012=CARTESIAN_POINT('Ctrl Pts',(43.6145820637333,1.59102591108104,0.));
#31013=CARTESIAN_POINT('Ctrl Pts',(43.7238422193529,1.53148589036097,0.));
#31014=CARTESIAN_POINT('Ctrl Pts',(43.8147465842502,1.48126213998559,0.));
#31015=CARTESIAN_POINT('Ctrl Pts',(43.8873767449248,1.44069595482723,0.));
#31016=CARTESIAN_POINT('Ctrl Pts',(43.9417969186811,1.41005374202872,0.));
#31017=CARTESIAN_POINT('Ctrl Pts',(43.9780537249529,1.38952890043916,0.));
#31018=CARTESIAN_POINT('',(43.9780537249529,-1.38952890043916,0.));
#31019=CARTESIAN_POINT('Origin',(1.13331566353736E-11,0.,0.));
#31020=CARTESIAN_POINT('',(37.4237196983922,-3.50724370857673,0.));
#31021=CARTESIAN_POINT('Ctrl Pts',(37.4237196983922,-3.50724370857673,0.));
#31022=CARTESIAN_POINT('Ctrl Pts',(37.4426037737699,-3.50901346997657,0.));
#31023=CARTESIAN_POINT('Ctrl Pts',(37.4803889700239,-3.51204731876361,0.));
#31024=CARTESIAN_POINT('Ctrl Pts',(37.5371179004295,-3.5150810906521,0.));
#31025=CARTESIAN_POINT('Ctrl Pts',(37.6128545966533,-3.51624243734645,0.));
#31026=CARTESIAN_POINT('Ctrl Pts',(37.7076643105286,-3.51375922979957,0.));
#31027=CARTESIAN_POINT('Ctrl Pts',(37.8025803811856,-3.50844720825128,0.));
#31028=CARTESIAN_POINT('Ctrl Pts',(37.8975688353863,-3.50139628556084,0.));
#31029=CARTESIAN_POINT('Ctrl Pts',(37.9926009950482,-3.49340804454645,0.));
#31030=CARTESIAN_POINT('Ctrl Pts',(38.0876589224537,-3.48478279878233,0.));
#31031=CARTESIAN_POINT('Ctrl Pts',(38.1827321816559,-3.47549027265411,0.));
#31032=CARTESIAN_POINT('Ctrl Pts',(38.2778154909527,-3.46530185256872,0.));
#31033=CARTESIAN_POINT('Ctrl Pts',(38.3729061502716,-3.45393053211023,0.));
#31034=CARTESIAN_POINT('Ctrl Pts',(38.4680013094732,-3.44118343200303,0.));
#31035=CARTESIAN_POINT('Ctrl Pts',(38.5630961226878,-3.42705871084997,0.));
#31036=CARTESIAN_POINT('Ctrl Pts',(38.6581847668347,-3.41166717511901,0.));
#31037=CARTESIAN_POINT('Ctrl Pts',(38.7532609709905,-3.39518333281818,0.));
#31038=CARTESIAN_POINT('Ctrl Pts',(38.8483186930884,-3.37778863054482,0.));
#31039=CARTESIAN_POINT('Ctrl Pts',(38.9433528420174,-3.35960922799481,0.));
#31040=CARTESIAN_POINT('Ctrl Pts',(39.0383596151636,-3.34068601264472,0.));
#31041=CARTESIAN_POINT('Ctrl Pts',(39.1333360409949,-3.32100933979557,0.));
#31042=CARTESIAN_POINT('Ctrl Pts',(39.2282796893977,-3.30054018081687,0.));
#31043=CARTESIAN_POINT('Ctrl Pts',(39.3231883392913,-3.27923485388117,0.));
#31044=CARTESIAN_POINT('Ctrl Pts',(39.4180596080755,-3.25707264313388,0.));
#31045=CARTESIAN_POINT('Ctrl Pts',(39.5128908052622,-3.23406609691661,0.));
#31046=CARTESIAN_POINT('Ctrl Pts',(39.607679107639,-3.21024640045595,0.));
#31047=CARTESIAN_POINT('Ctrl Pts',(39.7024216585552,-3.18565465503835,0.));
#31048=CARTESIAN_POINT('Ctrl Pts',(39.7971156880138,-3.16033160752804,0.));
#31049=CARTESIAN_POINT('Ctrl Pts',(39.8917586491576,-3.13430604330356,0.));
#31050=CARTESIAN_POINT('Ctrl Pts',(39.9863482523153,-3.10759149802908,0.));
#31051=CARTESIAN_POINT('Ctrl Pts',(40.0808823811787,-3.08019251155015,0.));
#31052=CARTESIAN_POINT('Ctrl Pts',(40.1753590391515,-3.05210847423071,0.));
#31053=CARTESIAN_POINT('Ctrl Pts',(40.2697762886113,-3.02333808901595,0.));
#31054=CARTESIAN_POINT('Ctrl Pts',(40.3641321823444,-2.9938844645822,0.));
#31055=CARTESIAN_POINT('Ctrl Pts',(40.4584247445196,-2.96375636417323,0.));
#31056=CARTESIAN_POINT('Ctrl Pts',(40.5526520010651,-2.93296560822894,0.));
#31057=CARTESIAN_POINT('Ctrl Pts',(40.6468119976928,-2.90152548734343,0.));
#31058=CARTESIAN_POINT('Ctrl Pts',(40.7409028213129,-2.86944892209898,0.));
#31059=CARTESIAN_POINT('Ctrl Pts',(40.8349226258683,-2.83674635946679,0.));
#31060=CARTESIAN_POINT('Ctrl Pts',(40.9288696352159,-2.80342531768405,0.));
#31061=CARTESIAN_POINT('Ctrl Pts',(41.0227421242398,-2.76949151194863,0.));
#31062=CARTESIAN_POINT('Ctrl Pts',(41.1165384061145,-2.73494956725006,0.));
#31063=CARTESIAN_POINT('Ctrl Pts',(41.2102568187956,-2.69980383625016,0.));
#31064=CARTESIAN_POINT('Ctrl Pts',(41.3038957096306,-2.66405934050118,0.));
#31065=CARTESIAN_POINT('Ctrl Pts',(41.3974534325936,-2.62772200460656,0.));
#31066=CARTESIAN_POINT('Ctrl Pts',(41.4909283577703,-2.59079818040172,0.));
#31067=CARTESIAN_POINT('Ctrl Pts',(41.5843188786284,-2.55329436064184,0.));
#31068=CARTESIAN_POINT('Ctrl Pts',(41.6776234194583,-2.51521684674477,0.));
#31069=CARTESIAN_POINT('Ctrl Pts',(41.7708404467532,-2.47657137427693,0.));
#31070=CARTESIAN_POINT('Ctrl Pts',(41.8639684667923,-2.43736301434201,0.));
#31071=CARTESIAN_POINT('Ctrl Pts',(41.9570060084039,-2.39759639399648,0.));
#31072=CARTESIAN_POINT('Ctrl Pts',(42.0499516093661,-2.35727584066429,0.));
#31073=CARTESIAN_POINT('Ctrl Pts',(42.1428038039937,-2.31640554742809,0.));
#31074=CARTESIAN_POINT('Ctrl Pts',(42.2355611060784,-2.27498976664775,0.));
#31075=CARTESIAN_POINT('Ctrl Pts',(42.3282220118033,-2.233032874655,0.));
#31076=CARTESIAN_POINT('Ctrl Pts',(42.4207850290047,-2.19053924976738,0.));
#31077=CARTESIAN_POINT('Ctrl Pts',(42.5132487024335,-2.14751319676745,0.));
#31078=CARTESIAN_POINT('Ctrl Pts',(42.6056116373455,-2.10395886401771,0.));
#31079=CARTESIAN_POINT('Ctrl Pts',(42.6978725343209,-2.05988014924519,0.));
#31080=CARTESIAN_POINT('Ctrl Pts',(42.7900301875309,-2.0152806752809,0.));
#31081=CARTESIAN_POINT('Ctrl Pts',(42.8820834139973,-1.97016390194216,0.));
#31082=CARTESIAN_POINT('Ctrl Pts',(42.9740309956624,-1.92453321512436,0.));
#31083=CARTESIAN_POINT('Ctrl Pts',(43.065871623255,-1.87839202014609,0.));
#31084=CARTESIAN_POINT('Ctrl Pts',(43.1576038253643,-1.83174385734712,0.));
#31085=CARTESIAN_POINT('Ctrl Pts',(43.2492259505872,-1.7845924484277,0.));
#31086=CARTESIAN_POINT('Ctrl Pts',(43.3407363140236,-1.73694151741124,0.));
#31087=CARTESIAN_POINT('Ctrl Pts',(43.4321333178711,-1.68879465270608,0.));
#31088=CARTESIAN_POINT('Ctrl Pts',(43.5234155788248,-1.64015515906648,0.));
#31089=CARTESIAN_POINT('Ctrl Pts',(43.6145820637333,-1.59102591108104,0.));
#31090=CARTESIAN_POINT('Ctrl Pts',(43.7238422193529,-1.53148589036097,0.));
#31091=CARTESIAN_POINT('Ctrl Pts',(43.8147465842502,-1.48126213998559,0.));
#31092=CARTESIAN_POINT('Ctrl Pts',(43.8873767449248,-1.44069595482723,0.));
#31093=CARTESIAN_POINT('Ctrl Pts',(43.9417969186811,-1.41005374202872,0.));
#31094=CARTESIAN_POINT('Ctrl Pts',(43.9780537249529,-1.38952890043916,0.));
#31095=CARTESIAN_POINT('',(36.199629211057,-3.39252545782466,0.));
#31096=CARTESIAN_POINT('',(35.2077250236291,-3.2995670413737,0.));
#31097=CARTESIAN_POINT('',(35.1136254352094,-4.26751599830831,0.));
#31098=CARTESIAN_POINT('Origin',(36.1063209411239,-4.38816272448461,0.));
#31099=CARTESIAN_POINT('Origin',(0.,0.,0.));
#31100=CARTESIAN_POINT('Origin',(0.,0.,0.));
#31101=CARTESIAN_POINT('Origin',(0.,0.,15.));
#31102=CARTESIAN_POINT('',(35.1136254352094,-4.26751599830831,15.));
#31103=CARTESIAN_POINT('Origin',(0.,0.,15.));
#31104=CARTESIAN_POINT('',(36.199629211057,-3.39252545782466,15.));
#31105=CARTESIAN_POINT('Origin',(36.1063209411239,-4.38816272448461,15.));
#31106=CARTESIAN_POINT('',(37.4237196983922,-3.50724370857673,15.));
#31107=CARTESIAN_POINT('',(35.2077250236291,-3.2995670413737,15.));
#31108=CARTESIAN_POINT('',(43.9780537249529,-1.38952890043916,15.));
#31109=CARTESIAN_POINT('Ctrl Pts',(37.4237196983922,-3.50724370857673,15.));
#31110=CARTESIAN_POINT('Ctrl Pts',(37.4426037737699,-3.50901346997657,15.));
#31111=CARTESIAN_POINT('Ctrl Pts',(37.4803889700239,-3.51204731876361,15.));
#31112=CARTESIAN_POINT('Ctrl Pts',(37.5371179004295,-3.5150810906521,15.));
#31113=CARTESIAN_POINT('Ctrl Pts',(37.6128545966533,-3.51624243734645,15.));
#31114=CARTESIAN_POINT('Ctrl Pts',(37.7076643105286,-3.51375922979957,15.));
#31115=CARTESIAN_POINT('Ctrl Pts',(37.8025803811856,-3.50844720825128,15.));
#31116=CARTESIAN_POINT('Ctrl Pts',(37.8975688353863,-3.50139628556084,15.));
#31117=CARTESIAN_POINT('Ctrl Pts',(37.9926009950482,-3.49340804454645,15.));
#31118=CARTESIAN_POINT('Ctrl Pts',(38.0876589224537,-3.48478279878233,15.));
#31119=CARTESIAN_POINT('Ctrl Pts',(38.1827321816559,-3.47549027265411,15.));
#31120=CARTESIAN_POINT('Ctrl Pts',(38.2778154909527,-3.46530185256872,15.));
#31121=CARTESIAN_POINT('Ctrl Pts',(38.3729061502716,-3.45393053211023,15.));
#31122=CARTESIAN_POINT('Ctrl Pts',(38.4680013094732,-3.44118343200303,15.));
#31123=CARTESIAN_POINT('Ctrl Pts',(38.5630961226878,-3.42705871084997,15.));
#31124=CARTESIAN_POINT('Ctrl Pts',(38.6581847668347,-3.41166717511901,15.));
#31125=CARTESIAN_POINT('Ctrl Pts',(38.7532609709905,-3.39518333281818,15.));
#31126=CARTESIAN_POINT('Ctrl Pts',(38.8483186930884,-3.37778863054482,15.));
#31127=CARTESIAN_POINT('Ctrl Pts',(38.9433528420174,-3.35960922799481,15.));
#31128=CARTESIAN_POINT('Ctrl Pts',(39.0383596151636,-3.34068601264472,15.));
#31129=CARTESIAN_POINT('Ctrl Pts',(39.1333360409949,-3.32100933979557,15.));
#31130=CARTESIAN_POINT('Ctrl Pts',(39.2282796893977,-3.30054018081687,15.));
#31131=CARTESIAN_POINT('Ctrl Pts',(39.3231883392913,-3.27923485388117,15.));
#31132=CARTESIAN_POINT('Ctrl Pts',(39.4180596080755,-3.25707264313388,15.));
#31133=CARTESIAN_POINT('Ctrl Pts',(39.5128908052622,-3.23406609691661,15.));
#31134=CARTESIAN_POINT('Ctrl Pts',(39.607679107639,-3.21024640045595,15.));
#31135=CARTESIAN_POINT('Ctrl Pts',(39.7024216585552,-3.18565465503835,15.));
#31136=CARTESIAN_POINT('Ctrl Pts',(39.7971156880138,-3.16033160752804,15.));
#31137=CARTESIAN_POINT('Ctrl Pts',(39.8917586491576,-3.13430604330356,15.));
#31138=CARTESIAN_POINT('Ctrl Pts',(39.9863482523153,-3.10759149802908,15.));
#31139=CARTESIAN_POINT('Ctrl Pts',(40.0808823811787,-3.08019251155015,15.));
#31140=CARTESIAN_POINT('Ctrl Pts',(40.1753590391515,-3.05210847423071,15.));
#31141=CARTESIAN_POINT('Ctrl Pts',(40.2697762886113,-3.02333808901595,15.));
#31142=CARTESIAN_POINT('Ctrl Pts',(40.3641321823444,-2.9938844645822,15.));
#31143=CARTESIAN_POINT('Ctrl Pts',(40.4584247445196,-2.96375636417323,15.));
#31144=CARTESIAN_POINT('Ctrl Pts',(40.5526520010651,-2.93296560822894,15.));
#31145=CARTESIAN_POINT('Ctrl Pts',(40.6468119976928,-2.90152548734343,15.));
#31146=CARTESIAN_POINT('Ctrl Pts',(40.7409028213129,-2.86944892209898,15.));
#31147=CARTESIAN_POINT('Ctrl Pts',(40.8349226258683,-2.83674635946679,15.));
#31148=CARTESIAN_POINT('Ctrl Pts',(40.9288696352159,-2.80342531768405,15.));
#31149=CARTESIAN_POINT('Ctrl Pts',(41.0227421242398,-2.76949151194863,15.));
#31150=CARTESIAN_POINT('Ctrl Pts',(41.1165384061145,-2.73494956725006,15.));
#31151=CARTESIAN_POINT('Ctrl Pts',(41.2102568187956,-2.69980383625016,15.));
#31152=CARTESIAN_POINT('Ctrl Pts',(41.3038957096306,-2.66405934050118,15.));
#31153=CARTESIAN_POINT('Ctrl Pts',(41.3974534325936,-2.62772200460656,15.));
#31154=CARTESIAN_POINT('Ctrl Pts',(41.4909283577703,-2.59079818040172,15.));
#31155=CARTESIAN_POINT('Ctrl Pts',(41.5843188786284,-2.55329436064184,15.));
#31156=CARTESIAN_POINT('Ctrl Pts',(41.6776234194583,-2.51521684674477,15.));
#31157=CARTESIAN_POINT('Ctrl Pts',(41.7708404467532,-2.47657137427693,15.));
#31158=CARTESIAN_POINT('Ctrl Pts',(41.8639684667923,-2.43736301434201,15.));
#31159=CARTESIAN_POINT('Ctrl Pts',(41.9570060084039,-2.39759639399648,15.));
#31160=CARTESIAN_POINT('Ctrl Pts',(42.0499516093661,-2.35727584066429,15.));
#31161=CARTESIAN_POINT('Ctrl Pts',(42.1428038039937,-2.31640554742809,15.));
#31162=CARTESIAN_POINT('Ctrl Pts',(42.2355611060784,-2.27498976664775,15.));
#31163=CARTESIAN_POINT('Ctrl Pts',(42.3282220118033,-2.233032874655,15.));
#31164=CARTESIAN_POINT('Ctrl Pts',(42.4207850290047,-2.19053924976738,15.));
#31165=CARTESIAN_POINT('Ctrl Pts',(42.5132487024335,-2.14751319676745,15.));
#31166=CARTESIAN_POINT('Ctrl Pts',(42.6056116373455,-2.10395886401771,15.));
#31167=CARTESIAN_POINT('Ctrl Pts',(42.6978725343209,-2.05988014924519,15.));
#31168=CARTESIAN_POINT('Ctrl Pts',(42.7900301875309,-2.0152806752809,15.));
#31169=CARTESIAN_POINT('Ctrl Pts',(42.8820834139973,-1.97016390194216,15.));
#31170=CARTESIAN_POINT('Ctrl Pts',(42.9740309956624,-1.92453321512436,15.));
#31171=CARTESIAN_POINT('Ctrl Pts',(43.065871623255,-1.87839202014609,15.));
#31172=CARTESIAN_POINT('Ctrl Pts',(43.1576038253643,-1.83174385734712,15.));
#31173=CARTESIAN_POINT('Ctrl Pts',(43.2492259505872,-1.7845924484277,15.));
#31174=CARTESIAN_POINT('Ctrl Pts',(43.3407363140236,-1.73694151741124,15.));
#31175=CARTESIAN_POINT('Ctrl Pts',(43.4321333178711,-1.68879465270608,15.));
#31176=CARTESIAN_POINT('Ctrl Pts',(43.5234155788248,-1.64015515906648,15.));
#31177=CARTESIAN_POINT('Ctrl Pts',(43.6145820637333,-1.59102591108104,15.));
#31178=CARTESIAN_POINT('Ctrl Pts',(43.7238422193529,-1.53148589036097,15.));
#31179=CARTESIAN_POINT('Ctrl Pts',(43.8147465842502,-1.48126213998559,15.));
#31180=CARTESIAN_POINT('Ctrl Pts',(43.8873767449248,-1.44069595482723,15.));
#31181=CARTESIAN_POINT('Ctrl Pts',(43.9417969186811,-1.41005374202872,15.));
#31182=CARTESIAN_POINT('Ctrl Pts',(43.9780537249529,-1.38952890043916,15.));
#31183=CARTESIAN_POINT('',(43.9780537249529,1.38952890043929,15.));
#31184=CARTESIAN_POINT('Origin',(1.13331566353736E-11,0.,15.));
#31185=CARTESIAN_POINT('',(37.4237196983922,3.50724370857673,15.));
#31186=CARTESIAN_POINT('Ctrl Pts',(43.9780537249529,1.38952890043916,15.));
#31187=CARTESIAN_POINT('Ctrl Pts',(43.9599253218251,1.39979132121931,15.));
#31188=CARTESIAN_POINT('Ctrl Pts',(43.9236568607623,1.42026781296156,15.));
#31189=CARTESIAN_POINT('Ctrl Pts',(43.8692192047561,1.45083750111682,15.));
#31190=CARTESIAN_POINT('Ctrl Pts',(43.7965657112707,1.49130689006067,15.));
#31191=CARTESIAN_POINT('Ctrl Pts',(43.7056321934163,1.54140922714765,15.));
#31192=CARTESIAN_POINT('Ctrl Pts',(43.6145820637333,1.59102591108104,15.));
#31193=CARTESIAN_POINT('Ctrl Pts',(43.5234155788248,1.64015515906648,15.));
#31194=CARTESIAN_POINT('Ctrl Pts',(43.4321333178711,1.68879465270608,15.));
#31195=CARTESIAN_POINT('Ctrl Pts',(43.3407363140236,1.73694151741124,15.));
#31196=CARTESIAN_POINT('Ctrl Pts',(43.2492259505872,1.7845924484277,15.));
#31197=CARTESIAN_POINT('Ctrl Pts',(43.1576038253643,1.83174385734712,15.));
#31198=CARTESIAN_POINT('Ctrl Pts',(43.065871623255,1.87839202014609,15.));
#31199=CARTESIAN_POINT('Ctrl Pts',(42.9740309956624,1.92453321512436,15.));
#31200=CARTESIAN_POINT('Ctrl Pts',(42.8820834139973,1.97016390194216,15.));
#31201=CARTESIAN_POINT('Ctrl Pts',(42.7900301875309,2.0152806752809,15.));
#31202=CARTESIAN_POINT('Ctrl Pts',(42.6978725343209,2.05988014924519,15.));
#31203=CARTESIAN_POINT('Ctrl Pts',(42.6056116373455,2.10395886401771,15.));
#31204=CARTESIAN_POINT('Ctrl Pts',(42.5132487024335,2.14751319676745,15.));
#31205=CARTESIAN_POINT('Ctrl Pts',(42.4207850290047,2.19053924976738,15.));
#31206=CARTESIAN_POINT('Ctrl Pts',(42.3282220118033,2.233032874655,15.));
#31207=CARTESIAN_POINT('Ctrl Pts',(42.2355611060784,2.27498976664775,15.));
#31208=CARTESIAN_POINT('Ctrl Pts',(42.1428038039937,2.31640554742809,15.));
#31209=CARTESIAN_POINT('Ctrl Pts',(42.0499516093661,2.35727584066429,15.));
#31210=CARTESIAN_POINT('Ctrl Pts',(41.9570060084039,2.39759639399648,15.));
#31211=CARTESIAN_POINT('Ctrl Pts',(41.8639684667923,2.43736301434201,15.));
#31212=CARTESIAN_POINT('Ctrl Pts',(41.7708404467532,2.47657137427693,15.));
#31213=CARTESIAN_POINT('Ctrl Pts',(41.6776234194583,2.51521684674477,15.));
#31214=CARTESIAN_POINT('Ctrl Pts',(41.5843188786284,2.55329436064184,15.));
#31215=CARTESIAN_POINT('Ctrl Pts',(41.4909283577703,2.59079818040172,15.));
#31216=CARTESIAN_POINT('Ctrl Pts',(41.3974534325936,2.62772200460656,15.));
#31217=CARTESIAN_POINT('Ctrl Pts',(41.3038957096306,2.66405934050118,15.));
#31218=CARTESIAN_POINT('Ctrl Pts',(41.2102568187956,2.69980383625016,15.));
#31219=CARTESIAN_POINT('Ctrl Pts',(41.1165384061145,2.73494956725006,15.));
#31220=CARTESIAN_POINT('Ctrl Pts',(41.0227421242398,2.76949151194863,15.));
#31221=CARTESIAN_POINT('Ctrl Pts',(40.9288696352159,2.80342531768405,15.));
#31222=CARTESIAN_POINT('Ctrl Pts',(40.8349226258683,2.83674635946679,15.));
#31223=CARTESIAN_POINT('Ctrl Pts',(40.7409028213129,2.86944892209898,15.));
#31224=CARTESIAN_POINT('Ctrl Pts',(40.6468119976928,2.90152548734343,15.));
#31225=CARTESIAN_POINT('Ctrl Pts',(40.5526520010651,2.93296560822894,15.));
#31226=CARTESIAN_POINT('Ctrl Pts',(40.4584247445196,2.96375636417323,15.));
#31227=CARTESIAN_POINT('Ctrl Pts',(40.3641321823444,2.9938844645822,15.));
#31228=CARTESIAN_POINT('Ctrl Pts',(40.2697762886113,3.02333808901595,15.));
#31229=CARTESIAN_POINT('Ctrl Pts',(40.1753590391515,3.05210847423071,15.));
#31230=CARTESIAN_POINT('Ctrl Pts',(40.0808823811787,3.08019251155015,15.));
#31231=CARTESIAN_POINT('Ctrl Pts',(39.9863482523153,3.10759149802908,15.));
#31232=CARTESIAN_POINT('Ctrl Pts',(39.8917586491576,3.13430604330356,15.));
#31233=CARTESIAN_POINT('Ctrl Pts',(39.7971156880138,3.16033160752804,15.));
#31234=CARTESIAN_POINT('Ctrl Pts',(39.7024216585552,3.18565465503835,15.));
#31235=CARTESIAN_POINT('Ctrl Pts',(39.607679107639,3.21024640045595,15.));
#31236=CARTESIAN_POINT('Ctrl Pts',(39.5128908052622,3.23406609691661,15.));
#31237=CARTESIAN_POINT('Ctrl Pts',(39.4180596080755,3.25707264313388,15.));
#31238=CARTESIAN_POINT('Ctrl Pts',(39.3231883392913,3.27923485388117,15.));
#31239=CARTESIAN_POINT('Ctrl Pts',(39.2282796893977,3.30054018081687,15.));
#31240=CARTESIAN_POINT('Ctrl Pts',(39.1333360409949,3.32100933979557,15.));
#31241=CARTESIAN_POINT('Ctrl Pts',(39.0383596151636,3.34068601264472,15.));
#31242=CARTESIAN_POINT('Ctrl Pts',(38.9433528420174,3.35960922799481,15.));
#31243=CARTESIAN_POINT('Ctrl Pts',(38.8483186930884,3.37778863054482,15.));
#31244=CARTESIAN_POINT('Ctrl Pts',(38.7532609709905,3.39518333281818,15.));
#31245=CARTESIAN_POINT('Ctrl Pts',(38.6581847668347,3.41166717511901,15.));
#31246=CARTESIAN_POINT('Ctrl Pts',(38.5630961226878,3.42705871084997,15.));
#31247=CARTESIAN_POINT('Ctrl Pts',(38.4680013094732,3.44118343200303,15.));
#31248=CARTESIAN_POINT('Ctrl Pts',(38.3729061502716,3.45393053211023,15.));
#31249=CARTESIAN_POINT('Ctrl Pts',(38.2778154909527,3.46530185256872,15.));
#31250=CARTESIAN_POINT('Ctrl Pts',(38.1827321816559,3.47549027265411,15.));
#31251=CARTESIAN_POINT('Ctrl Pts',(38.0876589224537,3.48478279878233,15.));
#31252=CARTESIAN_POINT('Ctrl Pts',(37.9926009950482,3.49340804454645,15.));
#31253=CARTESIAN_POINT('Ctrl Pts',(37.8975688353863,3.50139628556084,15.));
#31254=CARTESIAN_POINT('Ctrl Pts',(37.8025803811856,3.50844720825128,15.));
#31255=CARTESIAN_POINT('Ctrl Pts',(37.7076643105286,3.51375922979957,15.));
#31256=CARTESIAN_POINT('Ctrl Pts',(37.6128545966533,3.51624243734645,15.));
#31257=CARTESIAN_POINT('Ctrl Pts',(37.5371179004295,3.5150810906521,15.));
#31258=CARTESIAN_POINT('Ctrl Pts',(37.4803889700239,3.51204731876361,15.));
#31259=CARTESIAN_POINT('Ctrl Pts',(37.4426037737699,3.50901346997657,15.));
#31260=CARTESIAN_POINT('Ctrl Pts',(37.4237196983922,3.50724370857673,15.));
#31261=CARTESIAN_POINT('',(36.199629211057,3.39252545782466,15.));
#31262=CARTESIAN_POINT('',(35.2077250236291,3.2995670413737,15.));
#31263=CARTESIAN_POINT('',(35.1136254352094,4.26751599830831,15.));
#31264=CARTESIAN_POINT('Origin',(36.1063209411239,4.38816272448461,15.));
#31265=CARTESIAN_POINT('Origin',(0.,0.,15.));
#31266=CARTESIAN_POINT('Origin',(0.,0.,15.));
#31267=CARTESIAN_POINT('Origin',(0.,0.,15.));
#31268=CARTESIAN_POINT('Origin',(0.,0.,15.));
#31269=CARTESIAN_POINT('Origin',(0.,0.,15.));
#31270=CARTESIAN_POINT('Origin',(0.,0.,15.));
#31271=CARTESIAN_POINT('Origin',(0.,0.,15.));
#31272=CARTESIAN_POINT('Origin',(0.,0.,15.));
#31273=CARTESIAN_POINT('Origin',(0.,0.,15.));
#31274=CARTESIAN_POINT('Origin',(0.,0.,15.));
#31275=CARTESIAN_POINT('Origin',(0.,0.,15.));
#31276=CARTESIAN_POINT('Origin',(0.,0.,15.));
#31277=CARTESIAN_POINT('Origin',(0.,0.,15.));
#31278=CARTESIAN_POINT('Origin',(0.,0.,15.));
#31279=CARTESIAN_POINT('Origin',(0.,0.,15.));
#31280=CARTESIAN_POINT('Origin',(0.,0.,15.));
#31281=CARTESIAN_POINT('Origin',(0.,0.,15.));
#31282=CARTESIAN_POINT('Origin',(0.,0.,15.));
#31283=CARTESIAN_POINT('Origin',(0.,0.,15.));
#31284=CARTESIAN_POINT('Origin',(0.,0.,0.));
#31285=CARTESIAN_POINT('',(35.1136254352094,4.26751599830831,0.));
#31286=CARTESIAN_POINT('Origin',(0.,0.,0.));
#31287=CARTESIAN_POINT('Origin',(0.,0.,0.));
#31288=CARTESIAN_POINT('Origin',(0.,0.,0.));
#31289=CARTESIAN_POINT('Origin',(0.,0.,0.));
#31290=CARTESIAN_POINT('Origin',(0.,0.,0.));
#31291=CARTESIAN_POINT('Origin',(0.,0.,0.));
#31292=CARTESIAN_POINT('Origin',(0.,0.,0.));
#31293=CARTESIAN_POINT('Origin',(0.,0.,0.));
#31294=CARTESIAN_POINT('Origin',(0.,0.,0.));
#31295=CARTESIAN_POINT('Origin',(0.,0.,0.));
#31296=CARTESIAN_POINT('Origin',(0.,0.,0.));
#31297=CARTESIAN_POINT('Origin',(0.,0.,0.));
#31298=CARTESIAN_POINT('Origin',(0.,0.,0.));
#31299=CARTESIAN_POINT('Origin',(0.,0.,0.));
#31300=CARTESIAN_POINT('Origin',(0.,0.,0.));
#31301=CARTESIAN_POINT('Origin',(0.,0.,0.));
#31302=CARTESIAN_POINT('Origin',(0.,0.,0.));
#31303=CARTESIAN_POINT('Origin',(0.,0.,0.));
#31304=CARTESIAN_POINT('Origin',(36.1063209411239,4.38816272448461,0.));
#31305=CARTESIAN_POINT('',(36.199629211057,3.39252545782466,0.));
#31306=CARTESIAN_POINT('Origin',(37.4237196983922,3.50724370857673,0.));
#31307=CARTESIAN_POINT('',(37.4237196983922,3.50724370857673,0.));
#31308=CARTESIAN_POINT('Origin',(36.1063209411239,-4.38816272448461,0.));
#31309=CARTESIAN_POINT('',(36.199629211057,-3.39252545782466,0.));
#31310=CARTESIAN_POINT('',(35.1136254352094,-4.26751599830831,0.));
#31311=CARTESIAN_POINT('Origin',(35.2077250236291,-3.2995670413737,0.));
#31312=CARTESIAN_POINT('',(37.4237196983922,-3.50724370857673,0.));
#31313=CARTESIAN_POINT('Ctrl Pts',(43.9780537249529,1.38952890043916,0.));
#31314=CARTESIAN_POINT('Ctrl Pts',(43.9780537249529,1.38952890043916,18.));
#31315=CARTESIAN_POINT('Ctrl Pts',(43.9599253218251,1.39979132121931,0.));
#31316=CARTESIAN_POINT('Ctrl Pts',(43.9599253218251,1.39979132121931,18.));
#31317=CARTESIAN_POINT('Ctrl Pts',(43.9236568607623,1.42026781296156,0.));
#31318=CARTESIAN_POINT('Ctrl Pts',(43.9236568607623,1.42026781296156,18.));
#31319=CARTESIAN_POINT('Ctrl Pts',(43.8692192047561,1.45083750111682,0.));
#31320=CARTESIAN_POINT('Ctrl Pts',(43.8692192047561,1.45083750111682,18.));
#31321=CARTESIAN_POINT('Ctrl Pts',(43.7965657112707,1.49130689006067,0.));
#31322=CARTESIAN_POINT('Ctrl Pts',(43.7965657112707,1.49130689006067,18.));
#31323=CARTESIAN_POINT('Ctrl Pts',(43.7056321934163,1.54140922714765,0.));
#31324=CARTESIAN_POINT('Ctrl Pts',(43.7056321934163,1.54140922714765,18.));
#31325=CARTESIAN_POINT('Ctrl Pts',(43.6145820637333,1.59102591108104,0.));
#31326=CARTESIAN_POINT('Ctrl Pts',(43.6145820637333,1.59102591108104,18.));
#31327=CARTESIAN_POINT('Ctrl Pts',(43.5234155788248,1.64015515906648,0.));
#31328=CARTESIAN_POINT('Ctrl Pts',(43.5234155788248,1.64015515906648,18.));
#31329=CARTESIAN_POINT('Ctrl Pts',(43.4321333178711,1.68879465270608,0.));
#31330=CARTESIAN_POINT('Ctrl Pts',(43.4321333178711,1.68879465270608,18.));
#31331=CARTESIAN_POINT('Ctrl Pts',(43.3407363140236,1.73694151741124,0.));
#31332=CARTESIAN_POINT('Ctrl Pts',(43.3407363140236,1.73694151741124,18.));
#31333=CARTESIAN_POINT('Ctrl Pts',(43.2492259505872,1.7845924484277,0.));
#31334=CARTESIAN_POINT('Ctrl Pts',(43.2492259505872,1.7845924484277,18.));
#31335=CARTESIAN_POINT('Ctrl Pts',(43.1576038253643,1.83174385734712,0.));
#31336=CARTESIAN_POINT('Ctrl Pts',(43.1576038253643,1.83174385734712,18.));
#31337=CARTESIAN_POINT('Ctrl Pts',(43.065871623255,1.87839202014609,0.));
#31338=CARTESIAN_POINT('Ctrl Pts',(43.065871623255,1.87839202014609,18.));
#31339=CARTESIAN_POINT('Ctrl Pts',(42.9740309956624,1.92453321512436,0.));
#31340=CARTESIAN_POINT('Ctrl Pts',(42.9740309956624,1.92453321512436,18.));
#31341=CARTESIAN_POINT('Ctrl Pts',(42.8820834139973,1.97016390194216,0.));
#31342=CARTESIAN_POINT('Ctrl Pts',(42.8820834139973,1.97016390194216,18.));
#31343=CARTESIAN_POINT('Ctrl Pts',(42.7900301875309,2.0152806752809,0.));
#31344=CARTESIAN_POINT('Ctrl Pts',(42.7900301875309,2.0152806752809,18.));
#31345=CARTESIAN_POINT('Ctrl Pts',(42.6978725343209,2.05988014924519,0.));
#31346=CARTESIAN_POINT('Ctrl Pts',(42.6978725343209,2.05988014924519,18.));
#31347=CARTESIAN_POINT('Ctrl Pts',(42.6056116373455,2.10395886401771,0.));
#31348=CARTESIAN_POINT('Ctrl Pts',(42.6056116373455,2.10395886401771,18.));
#31349=CARTESIAN_POINT('Ctrl Pts',(42.5132487024335,2.14751319676745,0.));
#31350=CARTESIAN_POINT('Ctrl Pts',(42.5132487024335,2.14751319676745,18.));
#31351=CARTESIAN_POINT('Ctrl Pts',(42.4207850290047,2.19053924976738,0.));
#31352=CARTESIAN_POINT('Ctrl Pts',(42.4207850290047,2.19053924976738,18.));
#31353=CARTESIAN_POINT('Ctrl Pts',(42.3282220118033,2.233032874655,0.));
#31354=CARTESIAN_POINT('Ctrl Pts',(42.3282220118033,2.233032874655,18.));
#31355=CARTESIAN_POINT('Ctrl Pts',(42.2355611060784,2.27498976664775,0.));
#31356=CARTESIAN_POINT('Ctrl Pts',(42.2355611060784,2.27498976664775,18.));
#31357=CARTESIAN_POINT('Ctrl Pts',(42.1428038039937,2.31640554742809,0.));
#31358=CARTESIAN_POINT('Ctrl Pts',(42.1428038039937,2.31640554742809,18.));
#31359=CARTESIAN_POINT('Ctrl Pts',(42.0499516093661,2.35727584066429,0.));
#31360=CARTESIAN_POINT('Ctrl Pts',(42.0499516093661,2.35727584066429,18.));
#31361=CARTESIAN_POINT('Ctrl Pts',(41.9570060084039,2.39759639399648,0.));
#31362=CARTESIAN_POINT('Ctrl Pts',(41.9570060084039,2.39759639399648,18.));
#31363=CARTESIAN_POINT('Ctrl Pts',(41.8639684667923,2.43736301434201,0.));
#31364=CARTESIAN_POINT('Ctrl Pts',(41.8639684667923,2.43736301434201,18.));
#31365=CARTESIAN_POINT('Ctrl Pts',(41.7708404467532,2.47657137427693,0.));
#31366=CARTESIAN_POINT('Ctrl Pts',(41.7708404467532,2.47657137427693,18.));
#31367=CARTESIAN_POINT('Ctrl Pts',(41.6776234194583,2.51521684674477,0.));
#31368=CARTESIAN_POINT('Ctrl Pts',(41.6776234194583,2.51521684674477,18.));
#31369=CARTESIAN_POINT('Ctrl Pts',(41.5843188786284,2.55329436064184,0.));
#31370=CARTESIAN_POINT('Ctrl Pts',(41.5843188786284,2.55329436064184,18.));
#31371=CARTESIAN_POINT('Ctrl Pts',(41.4909283577703,2.59079818040172,0.));
#31372=CARTESIAN_POINT('Ctrl Pts',(41.4909283577703,2.59079818040172,18.));
#31373=CARTESIAN_POINT('Ctrl Pts',(41.3974534325936,2.62772200460656,0.));
#31374=CARTESIAN_POINT('Ctrl Pts',(41.3974534325936,2.62772200460656,18.));
#31375=CARTESIAN_POINT('Ctrl Pts',(41.3038957096306,2.66405934050118,0.));
#31376=CARTESIAN_POINT('Ctrl Pts',(41.3038957096306,2.66405934050118,18.));
#31377=CARTESIAN_POINT('Ctrl Pts',(41.2102568187956,2.69980383625016,0.));
#31378=CARTESIAN_POINT('Ctrl Pts',(41.2102568187956,2.69980383625016,18.));
#31379=CARTESIAN_POINT('Ctrl Pts',(41.1165384061145,2.73494956725006,0.));
#31380=CARTESIAN_POINT('Ctrl Pts',(41.1165384061145,2.73494956725006,18.));
#31381=CARTESIAN_POINT('Ctrl Pts',(41.0227421242398,2.76949151194863,0.));
#31382=CARTESIAN_POINT('Ctrl Pts',(41.0227421242398,2.76949151194863,18.));
#31383=CARTESIAN_POINT('Ctrl Pts',(40.9288696352159,2.80342531768405,0.));
#31384=CARTESIAN_POINT('Ctrl Pts',(40.9288696352159,2.80342531768405,18.));
#31385=CARTESIAN_POINT('Ctrl Pts',(40.8349226258683,2.83674635946679,0.));
#31386=CARTESIAN_POINT('Ctrl Pts',(40.8349226258683,2.83674635946679,18.));
#31387=CARTESIAN_POINT('Ctrl Pts',(40.7409028213129,2.86944892209898,0.));
#31388=CARTESIAN_POINT('Ctrl Pts',(40.7409028213129,2.86944892209898,18.));
#31389=CARTESIAN_POINT('Ctrl Pts',(40.6468119976928,2.90152548734343,0.));
#31390=CARTESIAN_POINT('Ctrl Pts',(40.6468119976928,2.90152548734343,18.));
#31391=CARTESIAN_POINT('Ctrl Pts',(40.5526520010651,2.93296560822894,0.));
#31392=CARTESIAN_POINT('Ctrl Pts',(40.5526520010651,2.93296560822894,18.));
#31393=CARTESIAN_POINT('Ctrl Pts',(40.4584247445196,2.96375636417323,0.));
#31394=CARTESIAN_POINT('Ctrl Pts',(40.4584247445196,2.96375636417323,18.));
#31395=CARTESIAN_POINT('Ctrl Pts',(40.3641321823444,2.9938844645822,0.));
#31396=CARTESIAN_POINT('Ctrl Pts',(40.3641321823444,2.9938844645822,18.));
#31397=CARTESIAN_POINT('Ctrl Pts',(40.2697762886113,3.02333808901595,0.));
#31398=CARTESIAN_POINT('Ctrl Pts',(40.2697762886113,3.02333808901595,18.));
#31399=CARTESIAN_POINT('Ctrl Pts',(40.1753590391515,3.05210847423071,0.));
#31400=CARTESIAN_POINT('Ctrl Pts',(40.1753590391515,3.05210847423071,18.));
#31401=CARTESIAN_POINT('Ctrl Pts',(40.0808823811787,3.08019251155015,0.));
#31402=CARTESIAN_POINT('Ctrl Pts',(40.0808823811787,3.08019251155015,18.));
#31403=CARTESIAN_POINT('Ctrl Pts',(39.9863482523153,3.10759149802908,0.));
#31404=CARTESIAN_POINT('Ctrl Pts',(39.9863482523153,3.10759149802908,18.));
#31405=CARTESIAN_POINT('Ctrl Pts',(39.8917586491576,3.13430604330356,0.));
#31406=CARTESIAN_POINT('Ctrl Pts',(39.8917586491576,3.13430604330356,18.));
#31407=CARTESIAN_POINT('Ctrl Pts',(39.7971156880138,3.16033160752804,0.));
#31408=CARTESIAN_POINT('Ctrl Pts',(39.7971156880138,3.16033160752804,18.));
#31409=CARTESIAN_POINT('Ctrl Pts',(39.7024216585552,3.18565465503835,0.));
#31410=CARTESIAN_POINT('Ctrl Pts',(39.7024216585552,3.18565465503835,18.));
#31411=CARTESIAN_POINT('Ctrl Pts',(39.607679107639,3.21024640045595,0.));
#31412=CARTESIAN_POINT('Ctrl Pts',(39.607679107639,3.21024640045595,18.));
#31413=CARTESIAN_POINT('Ctrl Pts',(39.5128908052622,3.23406609691661,0.));
#31414=CARTESIAN_POINT('Ctrl Pts',(39.5128908052622,3.23406609691661,18.));
#31415=CARTESIAN_POINT('Ctrl Pts',(39.4180596080755,3.25707264313388,0.));
#31416=CARTESIAN_POINT('Ctrl Pts',(39.4180596080755,3.25707264313388,18.));
#31417=CARTESIAN_POINT('Ctrl Pts',(39.3231883392913,3.27923485388117,0.));
#31418=CARTESIAN_POINT('Ctrl Pts',(39.3231883392913,3.27923485388117,18.));
#31419=CARTESIAN_POINT('Ctrl Pts',(39.2282796893977,3.30054018081687,0.));
#31420=CARTESIAN_POINT('Ctrl Pts',(39.2282796893977,3.30054018081687,18.));
#31421=CARTESIAN_POINT('Ctrl Pts',(39.1333360409949,3.32100933979557,0.));
#31422=CARTESIAN_POINT('Ctrl Pts',(39.1333360409949,3.32100933979557,18.));
#31423=CARTESIAN_POINT('Ctrl Pts',(39.0383596151636,3.34068601264472,0.));
#31424=CARTESIAN_POINT('Ctrl Pts',(39.0383596151636,3.34068601264472,18.));
#31425=CARTESIAN_POINT('Ctrl Pts',(38.9433528420174,3.35960922799481,0.));
#31426=CARTESIAN_POINT('Ctrl Pts',(38.9433528420174,3.35960922799481,18.));
#31427=CARTESIAN_POINT('Ctrl Pts',(38.8483186930884,3.37778863054482,0.));
#31428=CARTESIAN_POINT('Ctrl Pts',(38.8483186930884,3.37778863054482,18.));
#31429=CARTESIAN_POINT('Ctrl Pts',(38.7532609709905,3.39518333281818,0.));
#31430=CARTESIAN_POINT('Ctrl Pts',(38.7532609709905,3.39518333281818,18.));
#31431=CARTESIAN_POINT('Ctrl Pts',(38.6581847668347,3.41166717511901,0.));
#31432=CARTESIAN_POINT('Ctrl Pts',(38.6581847668347,3.41166717511901,18.));
#31433=CARTESIAN_POINT('Ctrl Pts',(38.5630961226878,3.42705871084997,0.));
#31434=CARTESIAN_POINT('Ctrl Pts',(38.5630961226878,3.42705871084997,18.));
#31435=CARTESIAN_POINT('Ctrl Pts',(38.4680013094732,3.44118343200303,0.));
#31436=CARTESIAN_POINT('Ctrl Pts',(38.4680013094732,3.44118343200303,18.));
#31437=CARTESIAN_POINT('Ctrl Pts',(38.3729061502716,3.45393053211023,0.));
#31438=CARTESIAN_POINT('Ctrl Pts',(38.3729061502716,3.45393053211023,18.));
#31439=CARTESIAN_POINT('Ctrl Pts',(38.2778154909527,3.46530185256872,0.));
#31440=CARTESIAN_POINT('Ctrl Pts',(38.2778154909527,3.46530185256872,18.));
#31441=CARTESIAN_POINT('Ctrl Pts',(38.1827321816559,3.47549027265411,0.));
#31442=CARTESIAN_POINT('Ctrl Pts',(38.1827321816559,3.47549027265411,18.));
#31443=CARTESIAN_POINT('Ctrl Pts',(38.0876589224537,3.48478279878233,0.));
#31444=CARTESIAN_POINT('Ctrl Pts',(38.0876589224537,3.48478279878233,18.));
#31445=CARTESIAN_POINT('Ctrl Pts',(37.9926009950482,3.49340804454645,0.));
#31446=CARTESIAN_POINT('Ctrl Pts',(37.9926009950482,3.49340804454645,18.));
#31447=CARTESIAN_POINT('Ctrl Pts',(37.8975688353863,3.50139628556084,0.));
#31448=CARTESIAN_POINT('Ctrl Pts',(37.8975688353863,3.50139628556084,18.));
#31449=CARTESIAN_POINT('Ctrl Pts',(37.8025803811856,3.50844720825128,0.));
#31450=CARTESIAN_POINT('Ctrl Pts',(37.8025803811856,3.50844720825128,18.));
#31451=CARTESIAN_POINT('Ctrl Pts',(37.7076643105286,3.51375922979957,0.));
#31452=CARTESIAN_POINT('Ctrl Pts',(37.7076643105286,3.51375922979957,18.));
#31453=CARTESIAN_POINT('Ctrl Pts',(37.6128545966533,3.51624243734645,0.));
#31454=CARTESIAN_POINT('Ctrl Pts',(37.6128545966533,3.51624243734645,18.));
#31455=CARTESIAN_POINT('Ctrl Pts',(37.5371179004295,3.5150810906521,0.));
#31456=CARTESIAN_POINT('Ctrl Pts',(37.5371179004295,3.5150810906521,18.));
#31457=CARTESIAN_POINT('Ctrl Pts',(37.4803889700239,3.51204731876361,0.));
#31458=CARTESIAN_POINT('Ctrl Pts',(37.4803889700239,3.51204731876361,18.));
#31459=CARTESIAN_POINT('Ctrl Pts',(37.4426037737699,3.50901346997657,0.));
#31460=CARTESIAN_POINT('Ctrl Pts',(37.4426037737699,3.50901346997657,18.));
#31461=CARTESIAN_POINT('Ctrl Pts',(37.4237196983922,3.50724370857673,0.));
#31462=CARTESIAN_POINT('Ctrl Pts',(37.4237196983922,3.50724370857673,18.));
#31463=CARTESIAN_POINT('',(43.9780537249529,1.38952890043929,0.));
#31464=CARTESIAN_POINT('Origin',(1.13331566353736E-11,0.,0.));
#31465=CARTESIAN_POINT('',(43.9780537249529,-1.38952890043916,0.));
#31466=CARTESIAN_POINT('Ctrl Pts',(37.4237196983922,-3.50724370857673,0.));
#31467=CARTESIAN_POINT('Ctrl Pts',(37.4237196983922,-3.50724370857673,18.));
#31468=CARTESIAN_POINT('Ctrl Pts',(37.4426037737699,-3.50901346997657,0.));
#31469=CARTESIAN_POINT('Ctrl Pts',(37.4426037737699,-3.50901346997657,18.));
#31470=CARTESIAN_POINT('Ctrl Pts',(37.4803889700239,-3.51204731876361,0.));
#31471=CARTESIAN_POINT('Ctrl Pts',(37.4803889700239,-3.51204731876361,18.));
#31472=CARTESIAN_POINT('Ctrl Pts',(37.5371179004295,-3.5150810906521,0.));
#31473=CARTESIAN_POINT('Ctrl Pts',(37.5371179004295,-3.5150810906521,18.));
#31474=CARTESIAN_POINT('Ctrl Pts',(37.6128545966533,-3.51624243734645,0.));
#31475=CARTESIAN_POINT('Ctrl Pts',(37.6128545966533,-3.51624243734645,18.));
#31476=CARTESIAN_POINT('Ctrl Pts',(37.7076643105286,-3.51375922979957,0.));
#31477=CARTESIAN_POINT('Ctrl Pts',(37.7076643105286,-3.51375922979957,18.));
#31478=CARTESIAN_POINT('Ctrl Pts',(37.8025803811856,-3.50844720825128,0.));
#31479=CARTESIAN_POINT('Ctrl Pts',(37.8025803811856,-3.50844720825128,18.));
#31480=CARTESIAN_POINT('Ctrl Pts',(37.8975688353863,-3.50139628556084,0.));
#31481=CARTESIAN_POINT('Ctrl Pts',(37.8975688353863,-3.50139628556084,18.));
#31482=CARTESIAN_POINT('Ctrl Pts',(37.9926009950482,-3.49340804454645,0.));
#31483=CARTESIAN_POINT('Ctrl Pts',(37.9926009950482,-3.49340804454645,18.));
#31484=CARTESIAN_POINT('Ctrl Pts',(38.0876589224537,-3.48478279878233,0.));
#31485=CARTESIAN_POINT('Ctrl Pts',(38.0876589224537,-3.48478279878233,18.));
#31486=CARTESIAN_POINT('Ctrl Pts',(38.1827321816559,-3.47549027265411,0.));
#31487=CARTESIAN_POINT('Ctrl Pts',(38.1827321816559,-3.47549027265411,18.));
#31488=CARTESIAN_POINT('Ctrl Pts',(38.2778154909527,-3.46530185256872,0.));
#31489=CARTESIAN_POINT('Ctrl Pts',(38.2778154909527,-3.46530185256872,18.));
#31490=CARTESIAN_POINT('Ctrl Pts',(38.3729061502716,-3.45393053211023,0.));
#31491=CARTESIAN_POINT('Ctrl Pts',(38.3729061502716,-3.45393053211023,18.));
#31492=CARTESIAN_POINT('Ctrl Pts',(38.4680013094732,-3.44118343200303,0.));
#31493=CARTESIAN_POINT('Ctrl Pts',(38.4680013094732,-3.44118343200303,18.));
#31494=CARTESIAN_POINT('Ctrl Pts',(38.5630961226878,-3.42705871084997,0.));
#31495=CARTESIAN_POINT('Ctrl Pts',(38.5630961226878,-3.42705871084997,18.));
#31496=CARTESIAN_POINT('Ctrl Pts',(38.6581847668347,-3.41166717511901,0.));
#31497=CARTESIAN_POINT('Ctrl Pts',(38.6581847668347,-3.41166717511901,18.));
#31498=CARTESIAN_POINT('Ctrl Pts',(38.7532609709905,-3.39518333281818,0.));
#31499=CARTESIAN_POINT('Ctrl Pts',(38.7532609709905,-3.39518333281818,18.));
#31500=CARTESIAN_POINT('Ctrl Pts',(38.8483186930884,-3.37778863054482,0.));
#31501=CARTESIAN_POINT('Ctrl Pts',(38.8483186930884,-3.37778863054482,18.));
#31502=CARTESIAN_POINT('Ctrl Pts',(38.9433528420174,-3.35960922799481,0.));
#31503=CARTESIAN_POINT('Ctrl Pts',(38.9433528420174,-3.35960922799481,18.));
#31504=CARTESIAN_POINT('Ctrl Pts',(39.0383596151636,-3.34068601264472,0.));
#31505=CARTESIAN_POINT('Ctrl Pts',(39.0383596151636,-3.34068601264472,18.));
#31506=CARTESIAN_POINT('Ctrl Pts',(39.1333360409949,-3.32100933979557,0.));
#31507=CARTESIAN_POINT('Ctrl Pts',(39.1333360409949,-3.32100933979557,18.));
#31508=CARTESIAN_POINT('Ctrl Pts',(39.2282796893977,-3.30054018081687,0.));
#31509=CARTESIAN_POINT('Ctrl Pts',(39.2282796893977,-3.30054018081687,18.));
#31510=CARTESIAN_POINT('Ctrl Pts',(39.3231883392913,-3.27923485388117,0.));
#31511=CARTESIAN_POINT('Ctrl Pts',(39.3231883392913,-3.27923485388117,18.));
#31512=CARTESIAN_POINT('Ctrl Pts',(39.4180596080755,-3.25707264313388,0.));
#31513=CARTESIAN_POINT('Ctrl Pts',(39.4180596080755,-3.25707264313388,18.));
#31514=CARTESIAN_POINT('Ctrl Pts',(39.5128908052622,-3.23406609691661,0.));
#31515=CARTESIAN_POINT('Ctrl Pts',(39.5128908052622,-3.23406609691661,18.));
#31516=CARTESIAN_POINT('Ctrl Pts',(39.607679107639,-3.21024640045595,0.));
#31517=CARTESIAN_POINT('Ctrl Pts',(39.607679107639,-3.21024640045595,18.));
#31518=CARTESIAN_POINT('Ctrl Pts',(39.7024216585552,-3.18565465503835,0.));
#31519=CARTESIAN_POINT('Ctrl Pts',(39.7024216585552,-3.18565465503835,18.));
#31520=CARTESIAN_POINT('Ctrl Pts',(39.7971156880138,-3.16033160752804,0.));
#31521=CARTESIAN_POINT('Ctrl Pts',(39.7971156880138,-3.16033160752804,18.));
#31522=CARTESIAN_POINT('Ctrl Pts',(39.8917586491576,-3.13430604330356,0.));
#31523=CARTESIAN_POINT('Ctrl Pts',(39.8917586491576,-3.13430604330356,18.));
#31524=CARTESIAN_POINT('Ctrl Pts',(39.9863482523153,-3.10759149802908,0.));
#31525=CARTESIAN_POINT('Ctrl Pts',(39.9863482523153,-3.10759149802908,18.));
#31526=CARTESIAN_POINT('Ctrl Pts',(40.0808823811787,-3.08019251155015,0.));
#31527=CARTESIAN_POINT('Ctrl Pts',(40.0808823811787,-3.08019251155015,18.));
#31528=CARTESIAN_POINT('Ctrl Pts',(40.1753590391515,-3.05210847423071,0.));
#31529=CARTESIAN_POINT('Ctrl Pts',(40.1753590391515,-3.05210847423071,18.));
#31530=CARTESIAN_POINT('Ctrl Pts',(40.2697762886113,-3.02333808901595,0.));
#31531=CARTESIAN_POINT('Ctrl Pts',(40.2697762886113,-3.02333808901595,18.));
#31532=CARTESIAN_POINT('Ctrl Pts',(40.3641321823444,-2.9938844645822,0.));
#31533=CARTESIAN_POINT('Ctrl Pts',(40.3641321823444,-2.9938844645822,18.));
#31534=CARTESIAN_POINT('Ctrl Pts',(40.4584247445196,-2.96375636417323,0.));
#31535=CARTESIAN_POINT('Ctrl Pts',(40.4584247445196,-2.96375636417323,18.));
#31536=CARTESIAN_POINT('Ctrl Pts',(40.5526520010651,-2.93296560822894,0.));
#31537=CARTESIAN_POINT('Ctrl Pts',(40.5526520010651,-2.93296560822894,18.));
#31538=CARTESIAN_POINT('Ctrl Pts',(40.6468119976928,-2.90152548734343,0.));
#31539=CARTESIAN_POINT('Ctrl Pts',(40.6468119976928,-2.90152548734343,18.));
#31540=CARTESIAN_POINT('Ctrl Pts',(40.7409028213129,-2.86944892209898,0.));
#31541=CARTESIAN_POINT('Ctrl Pts',(40.7409028213129,-2.86944892209898,18.));
#31542=CARTESIAN_POINT('Ctrl Pts',(40.8349226258683,-2.83674635946679,0.));
#31543=CARTESIAN_POINT('Ctrl Pts',(40.8349226258683,-2.83674635946679,18.));
#31544=CARTESIAN_POINT('Ctrl Pts',(40.9288696352159,-2.80342531768405,0.));
#31545=CARTESIAN_POINT('Ctrl Pts',(40.9288696352159,-2.80342531768405,18.));
#31546=CARTESIAN_POINT('Ctrl Pts',(41.0227421242398,-2.76949151194863,0.));
#31547=CARTESIAN_POINT('Ctrl Pts',(41.0227421242398,-2.76949151194863,18.));
#31548=CARTESIAN_POINT('Ctrl Pts',(41.1165384061145,-2.73494956725006,0.));
#31549=CARTESIAN_POINT('Ctrl Pts',(41.1165384061145,-2.73494956725006,18.));
#31550=CARTESIAN_POINT('Ctrl Pts',(41.2102568187956,-2.69980383625016,0.));
#31551=CARTESIAN_POINT('Ctrl Pts',(41.2102568187956,-2.69980383625016,18.));
#31552=CARTESIAN_POINT('Ctrl Pts',(41.3038957096306,-2.66405934050118,0.));
#31553=CARTESIAN_POINT('Ctrl Pts',(41.3038957096306,-2.66405934050118,18.));
#31554=CARTESIAN_POINT('Ctrl Pts',(41.3974534325936,-2.62772200460656,0.));
#31555=CARTESIAN_POINT('Ctrl Pts',(41.3974534325936,-2.62772200460656,18.));
#31556=CARTESIAN_POINT('Ctrl Pts',(41.4909283577703,-2.59079818040172,0.));
#31557=CARTESIAN_POINT('Ctrl Pts',(41.4909283577703,-2.59079818040172,18.));
#31558=CARTESIAN_POINT('Ctrl Pts',(41.5843188786284,-2.55329436064184,0.));
#31559=CARTESIAN_POINT('Ctrl Pts',(41.5843188786284,-2.55329436064184,18.));
#31560=CARTESIAN_POINT('Ctrl Pts',(41.6776234194583,-2.51521684674477,0.));
#31561=CARTESIAN_POINT('Ctrl Pts',(41.6776234194583,-2.51521684674477,18.));
#31562=CARTESIAN_POINT('Ctrl Pts',(41.7708404467532,-2.47657137427693,0.));
#31563=CARTESIAN_POINT('Ctrl Pts',(41.7708404467532,-2.47657137427693,18.));
#31564=CARTESIAN_POINT('Ctrl Pts',(41.8639684667923,-2.43736301434201,0.));
#31565=CARTESIAN_POINT('Ctrl Pts',(41.8639684667923,-2.43736301434201,18.));
#31566=CARTESIAN_POINT('Ctrl Pts',(41.9570060084039,-2.39759639399648,0.));
#31567=CARTESIAN_POINT('Ctrl Pts',(41.9570060084039,-2.39759639399648,18.));
#31568=CARTESIAN_POINT('Ctrl Pts',(42.0499516093661,-2.35727584066429,0.));
#31569=CARTESIAN_POINT('Ctrl Pts',(42.0499516093661,-2.35727584066429,18.));
#31570=CARTESIAN_POINT('Ctrl Pts',(42.1428038039937,-2.31640554742809,0.));
#31571=CARTESIAN_POINT('Ctrl Pts',(42.1428038039937,-2.31640554742809,18.));
#31572=CARTESIAN_POINT('Ctrl Pts',(42.2355611060784,-2.27498976664775,0.));
#31573=CARTESIAN_POINT('Ctrl Pts',(42.2355611060784,-2.27498976664775,18.));
#31574=CARTESIAN_POINT('Ctrl Pts',(42.3282220118033,-2.233032874655,0.));
#31575=CARTESIAN_POINT('Ctrl Pts',(42.3282220118033,-2.233032874655,18.));
#31576=CARTESIAN_POINT('Ctrl Pts',(42.4207850290047,-2.19053924976738,0.));
#31577=CARTESIAN_POINT('Ctrl Pts',(42.4207850290047,-2.19053924976738,18.));
#31578=CARTESIAN_POINT('Ctrl Pts',(42.5132487024335,-2.14751319676745,0.));
#31579=CARTESIAN_POINT('Ctrl Pts',(42.5132487024335,-2.14751319676745,18.));
#31580=CARTESIAN_POINT('Ctrl Pts',(42.6056116373455,-2.10395886401771,0.));
#31581=CARTESIAN_POINT('Ctrl Pts',(42.6056116373455,-2.10395886401771,18.));
#31582=CARTESIAN_POINT('Ctrl Pts',(42.6978725343209,-2.05988014924519,0.));
#31583=CARTESIAN_POINT('Ctrl Pts',(42.6978725343209,-2.05988014924519,18.));
#31584=CARTESIAN_POINT('Ctrl Pts',(42.7900301875309,-2.0152806752809,0.));
#31585=CARTESIAN_POINT('Ctrl Pts',(42.7900301875309,-2.0152806752809,18.));
#31586=CARTESIAN_POINT('Ctrl Pts',(42.8820834139973,-1.97016390194216,0.));
#31587=CARTESIAN_POINT('Ctrl Pts',(42.8820834139973,-1.97016390194216,18.));
#31588=CARTESIAN_POINT('Ctrl Pts',(42.9740309956624,-1.92453321512436,0.));
#31589=CARTESIAN_POINT('Ctrl Pts',(42.9740309956624,-1.92453321512436,18.));
#31590=CARTESIAN_POINT('Ctrl Pts',(43.065871623255,-1.87839202014609,0.));
#31591=CARTESIAN_POINT('Ctrl Pts',(43.065871623255,-1.87839202014609,18.));
#31592=CARTESIAN_POINT('Ctrl Pts',(43.1576038253643,-1.83174385734712,0.));
#31593=CARTESIAN_POINT('Ctrl Pts',(43.1576038253643,-1.83174385734712,18.));
#31594=CARTESIAN_POINT('Ctrl Pts',(43.2492259505872,-1.7845924484277,0.));
#31595=CARTESIAN_POINT('Ctrl Pts',(43.2492259505872,-1.7845924484277,18.));
#31596=CARTESIAN_POINT('Ctrl Pts',(43.3407363140236,-1.73694151741124,0.));
#31597=CARTESIAN_POINT('Ctrl Pts',(43.3407363140236,-1.73694151741124,18.));
#31598=CARTESIAN_POINT('Ctrl Pts',(43.4321333178711,-1.68879465270608,0.));
#31599=CARTESIAN_POINT('Ctrl Pts',(43.4321333178711,-1.68879465270608,18.));
#31600=CARTESIAN_POINT('Ctrl Pts',(43.5234155788248,-1.64015515906648,0.));
#31601=CARTESIAN_POINT('Ctrl Pts',(43.5234155788248,-1.64015515906648,18.));
#31602=CARTESIAN_POINT('Ctrl Pts',(43.6145820637333,-1.59102591108104,0.));
#31603=CARTESIAN_POINT('Ctrl Pts',(43.6145820637333,-1.59102591108104,18.));
#31604=CARTESIAN_POINT('Ctrl Pts',(43.7056321934163,-1.54140922714765,0.));
#31605=CARTESIAN_POINT('Ctrl Pts',(43.7056321934163,-1.54140922714765,18.));
#31606=CARTESIAN_POINT('Ctrl Pts',(43.7965657112707,-1.49130689006067,0.));
#31607=CARTESIAN_POINT('Ctrl Pts',(43.7965657112707,-1.49130689006067,18.));
#31608=CARTESIAN_POINT('Ctrl Pts',(43.8692192047561,-1.45083750111682,0.));
#31609=CARTESIAN_POINT('Ctrl Pts',(43.8692192047561,-1.45083750111682,18.));
#31610=CARTESIAN_POINT('Ctrl Pts',(43.9236568607623,-1.42026781296156,0.));
#31611=CARTESIAN_POINT('Ctrl Pts',(43.9236568607623,-1.42026781296156,18.));
#31612=CARTESIAN_POINT('Ctrl Pts',(43.9599253218251,-1.39979132121931,0.));
#31613=CARTESIAN_POINT('Ctrl Pts',(43.9599253218251,-1.39979132121931,18.));
#31614=CARTESIAN_POINT('Ctrl Pts',(43.9780537249529,-1.38952890043916,0.));
#31615=CARTESIAN_POINT('Ctrl Pts',(43.9780537249529,-1.38952890043916,18.));
#31616=CARTESIAN_POINT('Origin',(0.,0.,0.));
#43763=UNCERTAINTY_MEASURE_WITH_UNIT(LENGTH_MEASURE(0.01),#43782,
'DISTANCE_ACCURACY_VALUE',
'Maximum model space distance between geometric entities at asserted c
onnectivities');
#43771=UNCERTAINTY_MEASURE_WITH_UNIT(LENGTH_MEASURE(0.01),#43782,
'DISTANCE_ACCURACY_VALUE',
'Maximum model space distance between geometric entities at asserted c
onnectivities');
#43773=(
GEOMETRIC_REPRESENTATION_CONTEXT(3)
GLOBAL_UNCERTAINTY_ASSIGNED_CONTEXT((#43763))
GLOBAL_UNIT_ASSIGNED_CONTEXT((#43782,#43784,#43785))
REPRESENTATION_CONTEXT('','3D')
);
#43781=(
GEOMETRIC_REPRESENTATION_CONTEXT(3)
GLOBAL_UNCERTAINTY_ASSIGNED_CONTEXT((#43771))
GLOBAL_UNIT_ASSIGNED_CONTEXT((#43782,#43784,#43785))
REPRESENTATION_CONTEXT('','3D')
);
#43782=(
LENGTH_UNIT()
NAMED_UNIT(*)
SI_UNIT(.MILLI.,.METRE.)
);
#43784=(
NAMED_UNIT(*)
PLANE_ANGLE_UNIT()
SI_UNIT($,.RADIAN.)
);
#43785=(
NAMED_UNIT(*)
SI_UNIT($,.STERADIAN.)
SOLID_ANGLE_UNIT()
);
#43787=SHAPE_DEFINITION_REPRESENTATION(#43796,#43813);
#43796=PRODUCT_DEFINITION_SHAPE('',$,#43823);
#43813=SHAPE_REPRESENTATION('',(#13185),#43773);
#43821=PRODUCT_DEFINITION_CONTEXT('part definition',#43850,'design');
#43823=PRODUCT_DEFINITION('Spur Gear 20 teeth','Spur Gear 20 teeth',#43832,
#43821);
#43832=PRODUCT_DEFINITION_FORMATION('',$,#43853);
#43850=APPLICATION_CONTEXT(
'Core Data for Automotive Mechanical Design Process');
#43851=PRODUCT_CONTEXT('part definition',#43850,'mechanical');
#43853=PRODUCT('Spur Gear 20 teeth','Spur Gear 20 teeth',
'Spur Gear; Module: 4.0; Num Teeth: 20; Pressure Angle: 20.0; Backlash
: 0.00 mm',(#43851));
#43862=PRESENTATION_STYLE_ASSIGNMENT((#43865));
#43865=SURFACE_STYLE_USAGE(.BOTH.,#43868);
#43868=SURFACE_SIDE_STYLE('',(#43871));
#43871=SURFACE_STYLE_FILL_AREA(#43874);
#43874=FILL_AREA_STYLE('Opaque(203,203,203)',(#43877));
#43877=FILL_AREA_STYLE_COLOUR('Opaque(203,203,203)',#43880);
#43880=COLOUR_RGB('Opaque(203,203,203)', 0.09019608, 0.27058824, 0.51372549);
ENDSEC;
END-ISO-10303-21;
